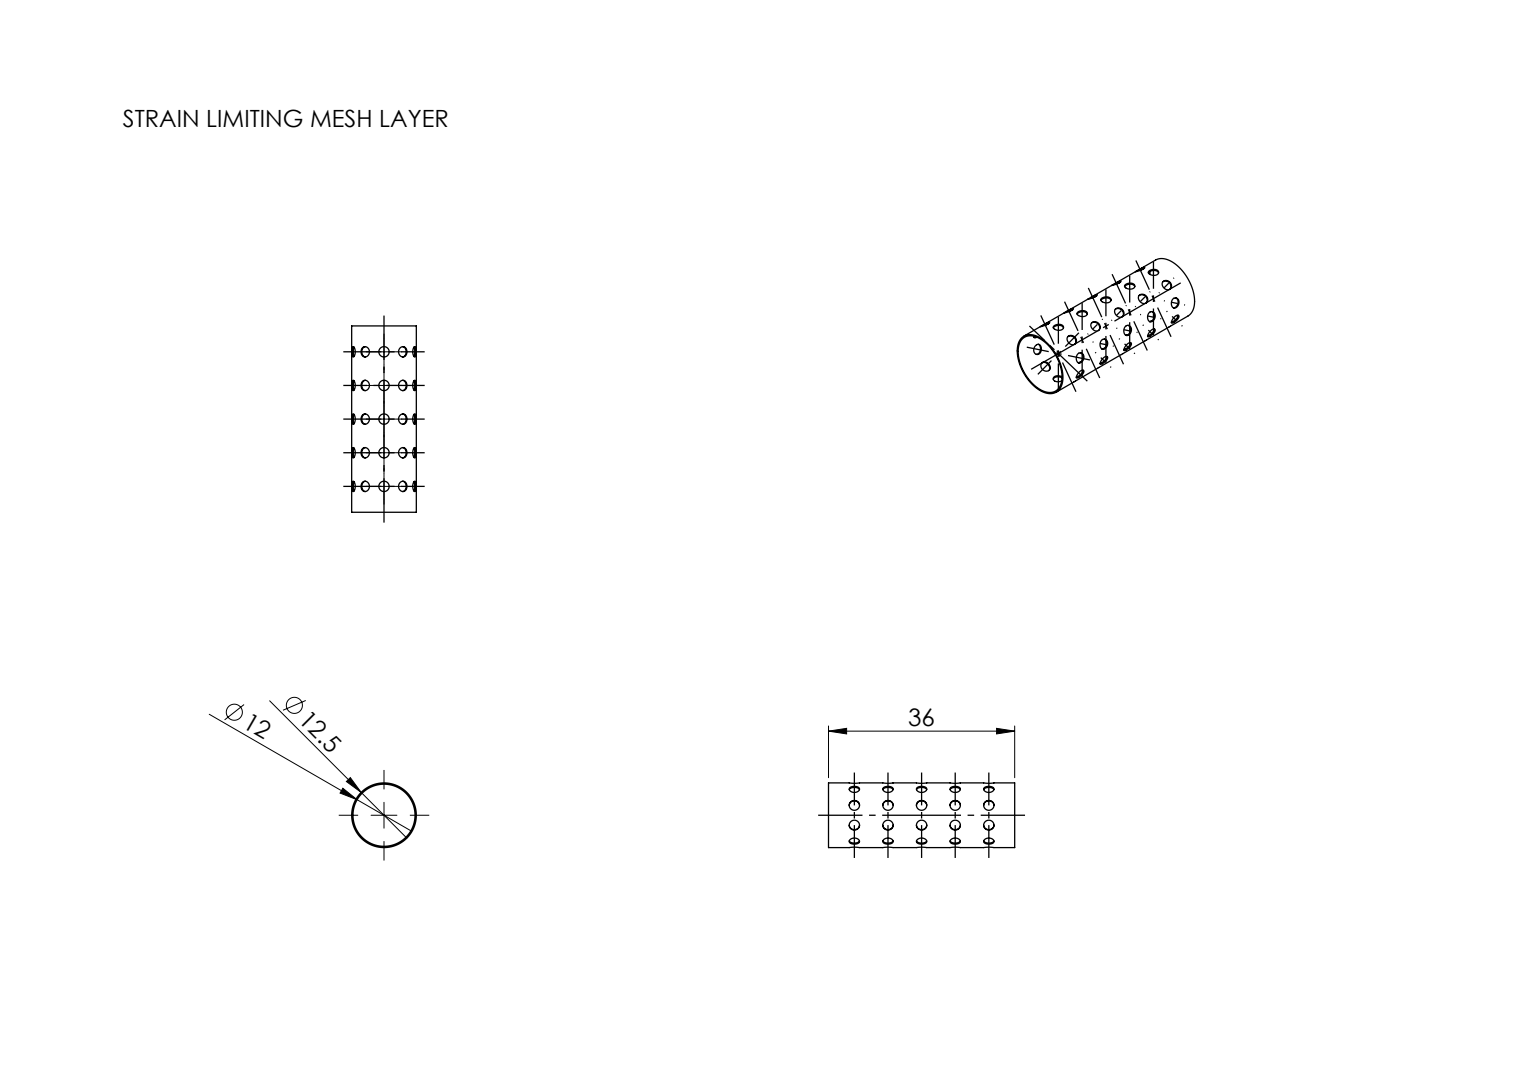
ISO-10303-21;
HEADER;
FILE_DESCRIPTION (('STEP AP214'),
    '1' );
FILE_NAME ('strain limiting mesh layer.step',
    '2026-10-04T10:31:01',
    ( '' ),
    ( '' ),
    'SwSTEP 2.0',
    'SolidWorks 2026',
    '' );
FILE_SCHEMA (( 'AUTOMOTIVE_DESIGN' ));
ENDSEC;

DATA;
#2=CARTESIAN_POINT ( 'NONE',  ( -5.408775798201173046, 2.598833957129639494, 10.88602261056916554 ) ) ;
#3=CARTESIAN_POINT ( 'NONE',  ( 5.866817325727491372, 1.260653813892048003, 4.199777826161211536 ) ) ;
#4=CARTESIAN_POINT ( 'NONE',  ( -5.621278735166248097, 2.101423246382425614, 30.02591947216899015 ) ) ;
#5=ORIENTED_EDGE ( 'NONE', *, *, #943, .F. ) ;
#6=ADVANCED_FACE ( 'NONE', ( #14827 ), #6324, .F. ) ;
#7=VECTOR ( 'NONE', #2853, 1000.000000000000000 ) ;
#11=EDGE_CURVE ( 'NONE', #6555, #15690, #9827, .T. ) ;
#12=EDGE_LOOP ( 'NONE', ( #2014, #1529, #7352, #6634 ) ) ;
#20=FACE_OUTER_BOUND ( 'NONE', #6226, .T. ) ;
#24=CARTESIAN_POINT ( 'NONE',  ( 6.081836621194421255, 1.445163676684907417, 5.873058915543010627 ) ) ;
#27=EDGE_LOOP ( 'NONE', ( #6618, #1977 ) ) ;
#28=VERTEX_POINT ( 'NONE', #11082 ) ;
#30=DIRECTION ( 'NONE',  ( 0.000000000000000000, 1.000000000000000000, 0.000000000000000000 ) ) ;
#32=CARTESIAN_POINT ( 'NONE',  ( -6.176542424588117974, 0.9554180641285662245, 31.13234125634169658 ) ) ;
#34=CARTESIAN_POINT ( 'NONE',  ( -3.107583187530418289, -5.133966411712689748, 12.37380682714709401 ) ) ;
#35=CARTESIAN_POINT ( 'NONE',  ( -5.769755079862331826, 2.405651898698942581, 5.873058915543010627 ) ) ;
#36=CARTESIAN_POINT ( 'NONE',  ( -6.176542424588075342, -0.9554180641288342324, 24.36765874365829987 ) ) ;
#37=CARTESIAN_POINT ( 'NONE',  ( 0.9999502950804096679, -5.916088184763849789, 24.63108149190011176 ) ) ;
#46=FACE_OUTER_BOUND ( 'NONE', #102, .T. ) ;
#47=CARTESIAN_POINT ( 'NONE',  ( 7.799024015210693328, -1.482594289696895551, 24.49999999999999289 ) ) ;
#50=CARTESIAN_POINT ( 'NONE',  ( -3.420311045507875125, 4.931422832349270813, 10.49992038825521767 ) ) ;
#51=EDGE_CURVE ( 'NONE', #13172, #10136, #3947, .T. ) ;
#53=LINE ( 'NONE', #4919, #15568 ) ;
#56=CARTESIAN_POINT ( 'NONE',  ( -4.070051655338111196, 4.744673454622471809, 5.873673286359928802 ) ) ;
#60=CARTESIAN_POINT ( 'NONE',  ( 5.558508435838322548, -2.857531096718671115, 24.49999999999999289 ) ) ;
#62=DIRECTION ( 'NONE',  ( -0.5877852522924685852, -0.8090169943749507819, 0.000000000000000000 ) ) ;
#66=CARTESIAN_POINT ( 'NONE',  ( 3.566234721238059624, 5.134387337253815353, 30.00008258189710730 ) ) ;
#69=CARTESIAN_POINT ( 'NONE',  ( 0.6151877315911880029, -6.220340188095996758, 25.29906673469669443 ) ) ;
#71=CARTESIAN_POINT ( 'NONE',  ( 2.817313151350924638, 5.579000502529565253, 24.49999999999999289 ) ) ;
#72=DIRECTION ( 'NONE',  ( -0.5877852522924685852, -0.8090169943749508930, 0.000000000000000000 ) ) ;
#74=CARTESIAN_POINT ( 'NONE',  ( 4.005785023174416537, -4.467917056767432449, 18.79952054102714243 ) ) ;
#76=CARTESIAN_POINT ( 'NONE',  ( -0.9737778612005270062, -5.920671847850523584, 30.73736375884650585 ) ) ;
#78=EDGE_CURVE ( 'NONE', #4035, #7910, #13252, .T. ) ;
#79=CARTESIAN_POINT ( 'NONE',  ( -0.9740012993918838458, -6.173846968979659344, 18.26164920628437471 ) ) ;
#83=B_SPLINE_CURVE_WITH_KNOTS ( 'NONE', 3,
 ( #5175, #14802, #5099, #8688, #8760, #13593, #1502, #6378, #11290, #544, #7481, #9951, #10027, #7789, #7554, #1580, #2625, #11212 ),
 .UNSPECIFIED., .F., .F.,
 ( 4, 2, 2, 2, 2, 2, 2, 2, 4 ),
 ( 0.000000000000000000, 0.0003914898357794967363, 0.0007829796715589934725, 0.001174469507338490263, 0.001565959343117986945, 0.001957449178897483627, 0.002348939014676980526, 0.002740428850456476991, 0.003131918686235973890 ),
 .UNSPECIFIED. ) ;
#85=ORIENTED_EDGE ( 'NONE', *, *, #14143, .F. ) ;
#86=CARTESIAN_POINT ( 'NONE',  ( -2.692215568229989753, 5.362327947133520567, 24.76229037835931734 ) ) ;
#89=CARTESIAN_POINT ( 'NONE',  ( 5.903472034603520768, 2.056448723545130974, 19.00008219321555103 ) ) ;
#90=CARTESIAN_POINT ( 'NONE',  ( 6.106056299406735555, 1.336851112280737386, 31.79887838423339730 ) ) ;
#92=EDGE_CURVE ( 'NONE', #15044, #5826, #4325, .T. ) ;
#95=LINE ( 'NONE', #7268, #828 ) ;
#97=CARTESIAN_POINT ( 'NONE',  ( 3.421280866381150698, 4.930711975950905490, 6.000049320733126024 ) ) ;
#99=CARTESIAN_POINT ( 'NONE',  ( 4.435347140101059793, -4.403429997944484420, 30.86762589283693714 ) ) ;
#102=EDGE_LOOP ( 'NONE', ( #11466, #15646, #12937, #12328 ) ) ;
#105=CARTESIAN_POINT ( 'NONE',  ( 1.354942165200771727E-13, 6.000000000000000888, 16.99999999999998579 ) ) ;
#107=CARTESIAN_POINT ( 'NONE',  ( 7.347880431581855163E-16, -6.250000000000000888, 4.000000000000004441 ) ) ;
#108=CARTESIAN_POINT ( 'NONE',  ( 3.010624175977998807, -5.190832888732208161, 12.29888242247939623 ) ) ;
#109=VECTOR ( 'NONE', #6035, 1000.000000000000114 ) ;
#111=CARTESIAN_POINT ( 'NONE',  ( 0.5042987395408317086, 5.979983180450071600, 12.37329304179975509 ) ) ;
#112=CARTESIAN_POINT ( 'NONE',  ( -0.2637975869345823843, -6.245592211692903462, 25.47332839949191197 ) ) ;
#114=CARTESIAN_POINT ( 'NONE',  ( -5.858813228503674253, 2.179803269293212331, 5.973772828752684561 ) ) ;
#115=CARTESIAN_POINT ( 'NONE',  ( 5.931828553037963303, 0.9033193133619970006, 30.73805675996854703 ) ) ;
#120=CARTESIAN_POINT ( 'NONE',  ( 5.866817325727508248, 1.260653813891974062, 10.69977782616119732 ) ) ;
#122=EDGE_LOOP ( 'NONE', ( #8457, #957, #1817, #14670 ) ) ;
#123=CARTESIAN_POINT ( 'NONE',  ( -3.735642931251032639, 4.696778275484473575, 5.974080527831013399 ) ) ;
#124=DIRECTION ( 'NONE',  ( -0.3090169943749584980, 0.9510565162951498674, 0.000000000000000000 ) ) ;
#125=CARTESIAN_POINT ( 'NONE',  ( 0.000000000000000000, 6.250000000000000888, 25.49999999999999645 ) ) ;
#126=CARTESIAN_POINT ( 'NONE',  ( 0.5031281619709804254, 5.980084330432649864, 23.62602272744524967 ) ) ;
#128=CARTESIAN_POINT ( 'NONE',  ( -2.782769401326250058, 5.315896561274810139, 10.99571079637980553 ) ) ;
#130=CARTESIAN_POINT ( 'NONE',  ( 5.621197618055712830, -2.101623592078416980, 4.026019798777604741 ) ) ;
#131=AXIS2_PLACEMENT_3D ( 'NONE', #7436, #13712, #10064 ) ;
#132=LINE ( 'NONE', #11034, #13057 ) ;
#137=CARTESIAN_POINT ( 'NONE',  ( 0.7995298244854847081, 5.947211616899245712, 31.61456014619858834 ) ) ;
#138=EDGE_LOOP ( 'NONE', ( #2074, #6168, #2631, #14050 ) ) ;
#141=CARTESIAN_POINT ( 'NONE',  ( -4.290821322214377176, -4.545321419741554791, 12.11441947245482886 ) ) ;
#142=VECTOR ( 'NONE', #3301, 1000.000000000000114 ) ;
#145=CYLINDRICAL_SURFACE ( 'NONE', #13956, 1.000000000000000888 ) ;
#149=DIRECTION ( 'NONE',  ( 0.8090169943749421222, 0.5877852522924802425, 0.000000000000000000 ) ) ;
#151=CARTESIAN_POINT ( 'NONE',  ( 5.782895619916224028, -1.604017620857841386, 25.47408052783099919 ) ) ;
#153=CARTESIAN_POINT ( 'NONE',  ( -1.000079958708118610, -5.916066267613704355, 31.13152738882033788 ) ) ;
#154=CARTESIAN_POINT ( 'NONE',  ( 5.621197618055728817, -2.101623592078373903, 10.52601979877759142 ) ) ;
#155=CARTESIAN_POINT ( 'NONE',  ( -4.435347140101089103, 4.403429997944455110, 31.00000000000000000 ) ) ;
#157=CARTESIAN_POINT ( 'NONE',  ( -5.935543223013860725, 0.8771126767606856056, 30.86760611998365178 ) ) ;
#158=EDGE_CURVE ( 'NONE', #3364, #642, #4897, .T. ) ;
#159=VERTEX_POINT ( 'NONE', #1682 ) ;
#160=EDGE_CURVE ( 'NONE', #4150, #13293, #5091, .T. ) ;
#163=CARTESIAN_POINT ( 'NONE',  ( -5.329907877631262281, -2.755840666746435019, 24.76194324003146008 ) ) ;
#165=ORIENTED_EDGE ( 'NONE', *, *, #10559, .T. ) ;
#172=CARTESIAN_POINT ( 'NONE',  ( -5.558508435838229289, 2.857531096718854524, 5.000000000000004441 ) ) ;
#174=CARTESIAN_POINT ( 'NONE',  ( 2.668367453516629517, 5.373994336898131330, 5.130649613488545313 ) ) ;
#178=EDGE_CURVE ( 'NONE', #5942, #5121, #706, .T. ) ;
#184=B_SPLINE_CURVE_WITH_KNOTS ( 'NONE', 3,
 ( #1419, #11210, #385, #5255, #7552, #10102, #6529, #6608, #14955, #11441, #11134, #235, #4046, #5097, #5411, #8917, #12556, #1655 ),
 .UNSPECIFIED., .F., .F.,
 ( 4, 2, 2, 2, 2, 2, 2, 2, 4 ),
 ( 0.003131918686235975625, 0.003523310662250265894, 0.003914702638264556597, 0.004306094614278846433, 0.004697486590293137136, 0.005088878566307427839, 0.005480270542321717675, 0.005871662518336007511, 0.006263054494350298214 ),
 .UNSPECIFIED. ) ;
#185=CARTESIAN_POINT ( 'NONE',  ( 6.123233995736766282E-16, -6.000000000000000888, 6.000000000000005329 ) ) ;
#186=CARTESIAN_POINT ( 'NONE',  ( 0.1306394121200732117, -6.249999999999998224, 16.99999999999998934 ) ) ;
#189=DIRECTION ( 'NONE',  ( -0.5877852522924685852, -0.8090169943749508930, 0.000000000000000000 ) ) ;
#190=CARTESIAN_POINT ( 'NONE',  ( 5.486982057989218120, -2.429327048029818137, 12.29931806258173488 ) ) ;
#191=CARTESIAN_POINT ( 'NONE',  ( -7.799024015210622274, -1.482594289697344969, 17.99999999999998934 ) ) ;
#203=CARTESIAN_POINT ( 'NONE',  ( -6.176542424588105540, -0.9554180641286327269, 5.000000000000004441 ) ) ;
#204=CARTESIAN_POINT ( 'NONE',  ( -5.859221468178929193, 2.178708437343280568, 23.52591457665828401 ) ) ;
#207=CARTESIAN_POINT ( 'NONE',  ( 6.176542424588116198, 0.9554180641285651143, 11.63060690723497537 ) ) ;
#212=CARTESIAN_POINT ( 'NONE',  ( 4.322356511625485176, 7.650514973136679941, 24.49999999999999289 ) ) ;
#216=CARTESIAN_POINT ( 'NONE',  ( -0.6144300524833441468, -6.220417338033054300, 30.20033372175933550 ) ) ;
#221=CARTESIAN_POINT ( 'NONE',  ( -3.567624405365271478, -5.133384272590760133, 10.50004921015705150 ) ) ;
#223=VECTOR ( 'NONE', #5063, 1000.000000000000114 ) ;
#225=CARTESIAN_POINT ( 'NONE',  ( 6.172651332693116721, -0.9815532474592382206, 18.26190213084011660 ) ) ;
#227=CARTESIAN_POINT ( 'NONE',  ( -3.735642931251134335, -4.696778275484388310, 23.52591947216897594 ) ) ;
#229=CARTESIAN_POINT ( 'NONE',  ( 5.903596343266298341, -2.055998103990583026, 31.99995078984293428 ) ) ;
#230=CARTESIAN_POINT ( 'NONE',  ( 5.131373506000437068, 7.062729720844210135, 24.49999999999999289 ) ) ;
#235=CARTESIAN_POINT ( 'NONE',  ( 3.922396193919112317, -4.541970110199391009, 5.873806827147107334 ) ) ;
#236=CARTESIAN_POINT ( 'NONE',  ( -5.746837578676007752, 1.729433780394243003, 10.50004946353775459 ) ) ;
#243=ORIENTED_EDGE ( 'NONE', *, *, #15436, .T. ) ;
#245=CARTESIAN_POINT ( 'NONE',  ( -2.782713018890816681, 5.315928322779066129, 25.00439760644211518 ) ) ;
#249=CARTESIAN_POINT ( 'NONE',  ( 5.770288754215144422, 2.404361317819916355, 18.87381964045070859 ) ) ;
#253=ADVANCED_FACE ( 'NONE', ( #9289 ), #846, .F. ) ;
#254=DIRECTION ( 'NONE',  ( 0.000000000000000000, 1.000000000000000000, 0.000000000000000000 ) ) ;
#255=DIRECTION ( 'NONE',  ( 0.8090169943749421222, 0.5877852522924802425, 0.000000000000000000 ) ) ;
#257=CARTESIAN_POINT ( 'NONE',  ( -6.155867707731118799, 1.081837891425841747, 30.49563030319847101 ) ) ;
#259=ORIENTED_EDGE ( 'NONE', *, *, #5440, .T. ) ;
#262=CARTESIAN_POINT ( 'NONE',  ( 5.330189595673648917, -2.755293208590215315, 30.73617396794403689 ) ) ;
#263=CARTESIAN_POINT ( 'NONE',  ( 4.153440676704428292, 4.671190581744466108, 4.200455375311575423 ) ) ;
#264=ORIENTED_EDGE ( 'NONE', *, *, #8261, .T. ) ;
#265=CARTESIAN_POINT ( 'NONE',  ( -6.155854678529451895, -1.081900940642234854, 17.49574050496990552 ) ) ;
#266=CARTESIAN_POINT ( 'NONE',  ( -2.849573632035295567, -5.280958870664590243, 18.61561732698604743 ) ) ;
#268=CARTESIAN_POINT ( 'NONE',  ( 3.254737477227910514, -5.337033878705263135, 23.62632671364006498 ) ) ;
#270=CARTESIAN_POINT ( 'NONE',  ( -3.159082487394833105, 5.393634094348302099, 10.70045537531157365 ) ) ;
#271=CARTESIAN_POINT ( 'NONE',  ( 1.000049560716759212, -5.916071405810109596, 24.36967799011533131 ) ) ;
#278=VERTEX_POINT ( 'NONE', #3158 ) ;
#279=CARTESIAN_POINT ( 'NONE',  ( -4.005361199354998014, 4.468319061418771554, 5.800222173838807116 ) ) ;
#281=CARTESIAN_POINT ( 'NONE',  ( -3.420311045507988368, 4.931422832349193541, 23.49992038825522656 ) ) ;
#284=CARTESIAN_POINT ( 'NONE',  ( -4.344762547369668049, -4.493114738039260203, 31.50308643866046054 ) ) ;
#287=CARTESIAN_POINT ( 'NONE',  ( -3.255013540813805673, 5.336859797930734395, 23.62618035954928786 ) ) ;
#290=CARTESIAN_POINT ( 'NONE',  ( 5.665707375537430757, 1.979196487016795292, 6.000079611744768115 ) ) ;
#292=FACE_OUTER_BOUND ( 'NONE', #8134, .T. ) ;
#295=B_SPLINE_CURVE_WITH_KNOTS ( 'NONE', 3,
 ( #10005, #367, #7304, #7609, #8735, #12457, #14777, #9696, #13567, #2677, #130, #7529, #13493, #1395, #2441, #6195, #14533, #1557 ),
 .UNSPECIFIED., .F., .F.,
 ( 4, 2, 2, 2, 2, 2, 2, 2, 4 ),
 ( 0.003131918686235955242, 0.003523310662250247680, 0.003914702638264540117, 0.004306094614278832555, 0.004697486590293124993, 0.005088878566307417431, 0.005480270542321709869, 0.005871662518336002307, 0.006263054494350294744 ),
 .UNSPECIFIED. ) ;
#296=CARTESIAN_POINT ( 'NONE',  ( 2.817313151351047207, 5.579000502529503080, 11.63063932754212892 ) ) ;
#298=AXIS2_PLACEMENT_3D ( 'NONE', #11149, #8855, #14815 ) ;
#300=CARTESIAN_POINT ( 'NONE',  ( 5.858736126997204252, -2.179962889276876314, 18.97359571723300320 ) ) ;
#303=CARTESIAN_POINT ( 'NONE',  ( -3.735642931251081489, -4.696778275484434495, 17.02591947216898305 ) ) ;
#305=B_SPLINE_CURVE_WITH_KNOTS ( 'NONE', 3,
 ( #6852, #13275, #12000, #11047, #9939, #6048, #6284, #2613, #8750, #15671, #227, #12235, #5087, #7393, #2293, #1336, #14715, #2456 ),
 .UNSPECIFIED., .F., .F.,
 ( 4, 2, 2, 2, 2, 2, 2, 2, 4 ),
 ( 0.000000000000000000, 0.0003914898357794977120, 0.0007829796715589954241, 0.001174469507338493082, 0.001565959343117990848, 0.001957449178897487096, 0.002348939014676983995, 0.002740428850456480461, 0.003131918686235977359 ),
 .UNSPECIFIED. ) ;
#306=CARTESIAN_POINT ( 'NONE',  ( -5.842945980534678618, 1.369128644668824446, 4.126215691297385746 ) ) ;
#307=FACE_OUTER_BOUND ( 'NONE', #5177, .T. ) ;
#308=CARTESIAN_POINT ( 'NONE',  ( 3.735808404764892732, 4.696639218303211294, 17.02601979877759319 ) ) ;
#312=CARTESIAN_POINT ( 'NONE',  ( -0.9737725088280894115, -6.173885267451843184, 17.73735758726564882 ) ) ;
#318=EDGE_LOOP ( 'NONE', ( #11239, #13450, #15608, #14902 ) ) ;
#322=CARTESIAN_POINT ( 'NONE',  ( -5.915653884842670962, -1.003805156977642943, 25.00439760644211518 ) ) ;
#324=ORIENTED_EDGE ( 'NONE', *, *, #12407, .T. ) ;
#328=CARTESIAN_POINT ( 'NONE',  ( -5.940390500375766436, 6.474944468551470322, 17.99999999999998934 ) ) ;
#331=CARTESIAN_POINT ( 'NONE',  ( -4.005361199354992685, -4.468319061418773330, 10.69977782616119022 ) ) ;
#332=CARTESIAN_POINT ( 'NONE',  ( 2.692143549875401831, 5.362363179736477470, 5.261943240031468960 ) ) ;
#334=CARTESIAN_POINT ( 'NONE',  ( 5.616116467183661420, -2.743044348085539319, 10.99574050496990019 ) ) ;
#335=CARTESIAN_POINT ( 'NONE',  ( -0.9735954530125078277, 6.173909381473996483, 31.26281793585242852 ) ) ;
#336=ORIENTED_EDGE ( 'NONE', *, *, #9119, .T. ) ;
#337=ORIENTED_EDGE ( 'NONE', *, *, #6167, .T. ) ;
#339=CARTESIAN_POINT ( 'NONE',  ( 0.2638277032950181455, 5.995407492418034501, 18.97332055281517427 ) ) ;
#341=ORIENTED_EDGE ( 'NONE', *, *, #869, .F. ) ;
#344=CARTESIAN_POINT ( 'NONE',  ( 0.8002302970946665317, -5.947135855825865569, 30.38601773212297985 ) ) ;
#345=CARTESIAN_POINT ( 'NONE',  ( -3.255128505894313573, 5.336774832660720058, 31.87380055247395561 ) ) ;
#346=CARTESIAN_POINT ( 'NONE',  ( 0.5030929395821815975, 6.230885867001134670, 17.12600319116549841 ) ) ;
#348=CARTESIAN_POINT ( 'NONE',  ( 5.131373506000546314, 7.062729720844130199, 11.49999999999998224 ) ) ;
#349=CARTESIAN_POINT ( 'NONE',  ( 5.665824935993635236, -1.978765057080846601, 12.49995053646221166 ) ) ;
#350=CARTESIAN_POINT ( 'NONE',  ( -3.882673863916385137, 4.899192824800864265, 18.97408542334169823 ) ) ;
#357=ORIENTED_EDGE ( 'NONE', *, *, #9015, .F. ) ;
#358=EDGE_CURVE ( 'NONE', #3603, #7463, #3951, .T. ) ;
#359=CARTESIAN_POINT ( 'NONE',  ( -6.176542424588100211, 0.9554180641286806885, 17.86762589283693359 ) ) ;
#361=CARTESIAN_POINT ( 'NONE',  ( -0.7993401192311853087, 6.199366368793661763, 5.614832469365748757 ) ) ;
#362=CARTESIAN_POINT ( 'NONE',  ( 5.903472034603497676, 2.056448723545192259, 12.50008219321554570 ) ) ;
#364=EDGE_CURVE ( 'NONE', #4594, #6555, #9214, .T. ) ;
#365=CARTESIAN_POINT ( 'NONE',  ( 2.848235266350880757, -5.281699484015723201, 23.88602261056919218 ) ) ;
#367=CARTESIAN_POINT ( 'NONE',  ( 5.935543223013858061, -0.8771126767606637342, 4.869383044678627925 ) ) ;
#368=CARTESIAN_POINT ( 'NONE',  ( -4.416837305303453753, -4.422286678979054919, 30.73809786915987630 ) ) ;
#370=FACE_BOUND ( 'NONE', #9710, .T. ) ;
#376=CARTESIAN_POINT ( 'NONE',  ( -5.866984344570811416, -1.259800266528728008, 18.79931806258173665 ) ) ;
#378=ORIENTED_EDGE ( 'NONE', *, *, #15661, .F. ) ;
#382=CARTESIAN_POINT ( 'NONE',  ( 3.922396193918944896, 4.541970110199535782, 17.12619317285288645 ) ) ;
#385=CARTESIAN_POINT ( 'NONE',  ( 2.692335458626972766, -5.362264153667172906, 5.262398918055980701 ) ) ;
#386=CARTESIAN_POINT ( 'NONE',  ( -3.923477796648569882, 4.541042560386435945, 30.12696220972948780 ) ) ;
#389=ORIENTED_EDGE ( 'NONE', *, *, #6341, .F. ) ;
#392=ORIENTED_EDGE ( 'NONE', *, *, #2098, .F. ) ;
#394=ORIENTED_EDGE ( 'NONE', *, *, #3851, .T. ) ;
#395=ADVANCED_FACE ( 'NONE', ( #5557 ), #9444, .F. ) ;
#396=CARTESIAN_POINT ( 'NONE',  ( 2.082642335314403343E-14, -6.250000000000000888, 31.00000000000000000 ) ) ;
#397=CYLINDRICAL_SURFACE ( 'NONE', #7859, 1.000000000000000888 ) ;
#398=VERTEX_POINT ( 'NONE', #14205 ) ;
#400=CARTESIAN_POINT ( 'NONE',  ( -4.290821322214388722, 4.545321419741542357, 4.385580527545153373 ) ) ;
#404=CARTESIAN_POINT ( 'NONE',  ( -5.984595133899170527, -1.806709459528687667, 5.999950789842938725 ) ) ;
#405=CARTESIAN_POINT ( 'NONE',  ( -2.849269941561969333, -5.281123252784043487, 10.88480617551147667 ) ) ;
#411=ORIENTED_EDGE ( 'NONE', *, *, #6538, .F. ) ;
#415=CARTESIAN_POINT ( 'NONE',  ( 0.7988914244719601543, 5.947301735519265442, 17.38456289168617985 ) ) ;
#417=ORIENTED_EDGE ( 'NONE', *, *, #12558, .T. ) ;
#418=CARTESIAN_POINT ( 'NONE',  ( -0.5031281619707669295, -5.980084330432671180, 4.126022727445256777 ) ) ;
#419=CARTESIAN_POINT ( 'NONE',  ( -6.176542424588117974, 0.9554180641285661135, 31.00000000000000000 ) ) ;
#420=CARTESIAN_POINT ( 'NONE',  ( -0.5039005892419784471, 6.230833003620553256, 17.12636388911295526 ) ) ;
#421=CARTESIAN_POINT ( 'NONE',  ( 0.2623718222036656722, 6.245654667075778654, 17.02627829713834373 ) ) ;
#425=CARTESIAN_POINT ( 'NONE',  ( 5.935543223013868719, 0.8771126767606117758, 18.13061695532137563 ) ) ;
#430=EDGE_LOOP ( 'NONE', ( #165, #8727 ) ) ;
#432=ORIENTED_EDGE ( 'NONE', *, *, #11524, .T. ) ;
#433=CARTESIAN_POINT ( 'NONE',  ( -5.615973259022290165, 2.743340227996234226, 17.49610786875029689 ) ) ;
#434=CARTESIAN_POINT ( 'NONE',  ( -6.142908455506919552, 1.155755562476170839, 23.88482219624156855 ) ) ;
#436=CARTESIAN_POINT ( 'NONE',  ( 5.571002711501404470, 2.833546409886289030, 11.76379616840804232 ) ) ;
#438=CARTESIAN_POINT ( 'NONE',  ( 2.840966774240223369, 5.567223638426877841, 5.261902130840121039 ) ) ;
#442=B_SPLINE_CURVE_WITH_KNOTS ( 'NONE', 3,
 ( #14232, #2140, #3189, #9317, #15286, #5742, #4389, #1910, #5509, #9242, #12806, #718, #1989, #8126, #11536, #6706, #14078, #6862 ),
 .UNSPECIFIED., .F., .F.,
 ( 4, 2, 2, 2, 2, 2, 2, 2, 4 ),
 ( 0.003131918686235976492, 0.003523310662250267195, 0.003914702638264558332, 0.004306094614278849035, 0.004697486590293139738, 0.005088878566307430441, 0.005480270542321721144, 0.005871662518336011848, 0.006263054494350302551 ),
 .UNSPECIFIED. ) ;
#443=DIRECTION ( 'NONE',  ( 0.000000000000000000, 1.000000000000000000, 0.000000000000000000 ) ) ;
#445=EDGE_CURVE ( 'NONE', #2248, #14335, #14582, .T. ) ;
#449=CARTESIAN_POINT ( 'NONE',  ( -2.997451966578398075, -5.485105005466015982, 10.88482219624155967 ) ) ;
#452=CARTESIAN_POINT ( 'NONE',  ( -2.782713018890758061, 5.315928322779098991, 18.50439760644211518 ) ) ;
#455=CARTESIAN_POINT ( 'NONE',  ( -2.841041022017427142, -5.567186575787240521, 17.73774718278285434 ) ) ;
#456=VECTOR ( 'NONE', #13750, 1000.000000000000000 ) ;
#458=FACE_OUTER_BOUND ( 'NONE', #7735, .T. ) ;
#462=DIRECTION ( 'NONE',  ( 0.5877852522924802425, -0.8090169943749422332, 0.000000000000000000 ) ) ;
#463=CARTESIAN_POINT ( 'NONE',  ( -5.935543223013843850, -0.8771126767607685393, 31.00000000000000000 ) ) ;
#464=AXIS2_PLACEMENT_3D ( 'NONE', #9917, #5307, #2906 ) ;
#465=CYLINDRICAL_SURFACE ( 'NONE', #13069, 1.000000000000000222 ) ;
#467=VECTOR ( 'NONE', #1666, 1000.000000000000000 ) ;
#468=CARTESIAN_POINT ( 'NONE',  ( -5.620879908643933831, -2.102487719021981949, 10.52622176056705428 ) ) ;
#471=VERTEX_POINT ( 'NONE', #4671 ) ;
#472=CARTESIAN_POINT ( 'NONE',  ( -5.915641100987803824, 1.003868594704913519, 25.00428920362019625 ) ) ;
#473=ORIENTED_EDGE ( 'NONE', *, *, #2610, .T. ) ;
#474=EDGE_CURVE ( 'NONE', #3929, #6460, #15716, .T. ) ;
#475=CYLINDRICAL_SURFACE ( 'NONE', #10388, 1.000000000000000666 ) ;
#478=VERTEX_POINT ( 'NONE', #125 ) ;
#479=AXIS2_PLACEMENT_3D ( 'NONE', #15199, #7061, #4294 ) ;
#484=CARTESIAN_POINT ( 'NONE',  ( -6.176542424588106428, -0.9554180641286325049, 5.132374107163055754 ) ) ;
#485=CARTESIAN_POINT ( 'NONE',  ( -4.286401442266578599, -4.198423832313146420, 11.49999999999998224 ) ) ;
#489=CARTESIAN_POINT ( 'NONE',  ( 4.142173849413700815, 4.341773579105447922, 12.11519382448850557 ) ) ;
#490=ORIENTED_EDGE ( 'NONE', *, *, #8030, .T. ) ;
#493=ORIENTED_EDGE ( 'NONE', *, *, #9967, .T. ) ;
#494=EDGE_CURVE ( 'NONE', #11779, #1022, #11976, .T. ) ;
#496=CARTESIAN_POINT ( 'NONE',  ( -6.176542424588095770, -0.9554180641287001174, 11.49999999999998224 ) ) ;
#497=CARTESIAN_POINT ( 'NONE',  ( 5.903596343266263702, 2.055998103990681614, 4.000049210157071045 ) ) ;
#498=EDGE_LOOP ( 'NONE', ( #13781, #14669 ) ) ;
#500=CARTESIAN_POINT ( 'NONE',  ( 1.354942164390165777E-13, -6.250000000000000888, 16.99999999999998579 ) ) ;
#502=CARTESIAN_POINT ( 'NONE',  ( -5.330004929009617420, 2.755647751839342519, 5.262398918055979813 ) ) ;
#505=CARTESIAN_POINT ( 'NONE',  ( 2.668367453516569121, 5.373994336898161528, 11.36938304467859773 ) ) ;
#511=B_SPLINE_CURVE_WITH_KNOTS ( 'NONE', 3,
 ( #8242, #10938, #9758, #13397, #14433, #4661, #3454, #10855, #2341, #13243, #11014, #2259, #5933, #3375, #14601, #14346, #36, #7047 ),
 .UNSPECIFIED., .F., .F.,
 ( 4, 2, 2, 2, 2, 2, 2, 2, 4 ),
 ( 0.003131486019301990727, 0.003522824630466696565, 0.003914163241631402404, 0.004305501852796108676, 0.004696840463960814081, 0.005088179075125522088, 0.005479517686290229228, 0.005870856297454936368, 0.006262194908619643507 ),
 .UNSPECIFIED. ) ;
#513=CARTESIAN_POINT ( 'NONE',  ( -4.070863287254244511, 4.743975846881662406, 17.12694108445698760 ) ) ;
#514=DIRECTION ( 'NONE',  ( 0.9510565162951499785, 0.3090169943749582204, 0.000000000000000000 ) ) ;
#515=CARTESIAN_POINT ( 'NONE',  ( -0.1306394121199367930, 6.250000000000000888, 4.000000000000004441 ) ) ;
#516=CARTESIAN_POINT ( 'NONE',  ( 5.903596343266268143, 2.055998103990667403, 30.00004921015706572 ) ) ;
#518=CARTESIAN_POINT ( 'NONE',  ( 4.142173849413673281, -4.341773579105472791, 23.88480617551147844 ) ) ;
#520=CARTESIAN_POINT ( 'NONE',  ( -4.267838854167106177, -4.217593933790406702, 31.26239891805596827 ) ) ;
#522=CARTESIAN_POINT ( 'NONE',  ( -5.131373506000878493, 7.062729720843910819, 24.49999999999999289 ) ) ;
#527=FACE_BOUND ( 'NONE', #5862, .T. ) ;
#530=CARTESIAN_POINT ( 'NONE',  ( -5.915653884842685173, -1.003805156977577662, 18.50439760644211518 ) ) ;
#535=CARTESIAN_POINT ( 'NONE',  ( -4.286401442266626560, -4.198423832313095794, 17.86935038651143515 ) ) ;
#536=CARTESIAN_POINT ( 'NONE',  ( 5.935543223013878489, -0.8771126767605277319, 17.86938304467860306 ) ) ;
#541=CARTESIAN_POINT ( 'NONE',  ( -0.6139908388540702422, 5.969238533166615568, 30.19977627912012252 ) ) ;
#543=LINE ( 'NONE', #1579, #12817 ) ;
#544=CARTESIAN_POINT ( 'NONE',  ( -5.666074146197981776, -1.978051345703211839, 12.50004932073310471 ) ) ;
#548=ORIENTED_EDGE ( 'NONE', *, *, #8965, .T. ) ;
#549=CARTESIAN_POINT ( 'NONE',  ( -5.317509234263835260, -2.779225709351231366, 24.49999999999999289 ) ) ;
#551=ORIENTED_EDGE ( 'NONE', *, *, #6800, .F. ) ;
#554=FACE_OUTER_BOUND ( 'NONE', #8032, .T. ) ;
#558=CARTESIAN_POINT ( 'NONE',  ( -0.5039079366031161689, 5.980031194523161453, 17.12637068109811977 ) ) ;
#559=CARTESIAN_POINT ( 'NONE',  ( 5.317509234264064411, -2.779225709350791274, 24.49999999999999289 ) ) ;
#566=CARTESIAN_POINT ( 'NONE',  ( 2.668367453516568677, 5.373994336898162416, 11.63064961348853465 ) ) ;
#567=VERTEX_POINT ( 'NONE', #9606 ) ;
#568=AXIS2_PLACEMENT_3D ( 'NONE', #14972, #12418, #11226 ) ;
#571=CARTESIAN_POINT ( 'NONE',  ( -6.142844459177225325, -1.156093792145260979, 10.88439807107078394 ) ) ;
#572=CARTESIAN_POINT ( 'NONE',  ( 6.155912734541117537, 1.081577393120979780, 4.496107868750329750 ) ) ;
#574=CARTESIAN_POINT ( 'NONE',  ( 5.903347812666375205, -1.076697810262440491, 18.61397738943082203 ) ) ;
#576=CARTESIAN_POINT ( 'NONE',  ( -0.9999505860952112579, 6.169489349035827352, 18.13105903165805799 ) ) ;
#577=CARTESIAN_POINT ( 'NONE',  ( 5.859155363331400856, -2.178872204144929992, 30.02599901976670438 ) ) ;
#580=LINE ( 'NONE', #4165, #11320 ) ;
#581=CARTESIAN_POINT ( 'NONE',  ( 3.922396193918995522, 4.541970110199488708, 10.62619317285287934 ) ) ;
#582=EDGE_CURVE ( 'NONE', #9339, #5163, #6425, .T. ) ;
#586=EDGE_CURVE ( 'NONE', #15318, #4525, #2806, .T. ) ;
#588=CARTESIAN_POINT ( 'NONE',  ( 3.011899281037532461, -5.190111395030209351, 4.199777826161210648 ) ) ;
#590=CARTESIAN_POINT ( 'NONE',  ( 4.435347140101073116, -4.403429997944470209, 5.000000000000004441 ) ) ;
#591=DIRECTION ( 'NONE',  ( -0.9510565162951545304, 0.3090169943749447867, 0.000000000000000000 ) ) ;
#593=CARTESIAN_POINT ( 'NONE',  ( -0.8737888311110042494, 5.936248257219510549, 5.503441851412170571 ) ) ;
#595=CARTESIAN_POINT ( 'NONE',  ( 3.882809187878910606, 4.899079348630070108, 10.52599901976669017 ) ) ;
#596=CARTESIAN_POINT ( 'NONE',  ( 4.069684453406305025, 4.744965295353549273, 5.873800552473966263 ) ) ;
#597=CARTESIAN_POINT ( 'NONE',  ( 6.143143148203058956, -1.154591847827712403, 31.61396179408071916 ) ) ;
#600=CARTESIAN_POINT ( 'NONE',  ( 5.935543223013847403, 0.8771126767607483332, 5.130616955321390726 ) ) ;
#604=CARTESIAN_POINT ( 'NONE',  ( 6.172614129015239648, -0.9817721000788448560, 30.73763026556126832 ) ) ;
#610=CARTESIAN_POINT ( 'NONE',  ( -3.922672396097112824, -4.541739265057652020, 17.12635295315576300 ) ) ;
#613=CARTESIAN_POINT ( 'NONE',  ( -5.487348639458814681, 2.428538342494583890, 23.69977782616121331 ) ) ;
#616=LINE ( 'NONE', #4206, #9107 ) ;
#617=CARTESIAN_POINT ( 'NONE',  ( -0.5039079366032207519, 5.980031194523153459, 30.12637068109813043 ) ) ;
#619=CARTESIAN_POINT ( 'NONE',  ( -4.286401442266607020, 4.198423832313117110, 31.00000000000000000 ) ) ;
#620=CARTESIAN_POINT ( 'NONE',  ( -6.176542424588121527, 0.9554180641285457964, 4.867625892836954904 ) ) ;
#621=DIRECTION ( 'NONE',  ( 0.9510565162951499785, 0.3090169943749582204, 0.000000000000000000 ) ) ;
#624=CARTESIAN_POINT ( 'NONE',  ( 2.668367453516611754, 5.373994336898140212, 30.86938304467861727 ) ) ;
#626=CYLINDRICAL_SURFACE ( 'NONE', #9896, 1.000000000000000888 ) ;
#628=CARTESIAN_POINT ( 'NONE',  ( -5.931734679891443207, -0.9039278060244418933, 30.73617396794404044 ) ) ;
#629=CARTESIAN_POINT ( 'NONE',  ( -4.344762547369716899, 4.493114738039211353, 4.496913561339538568 ) ) ;
#634=CARTESIAN_POINT ( 'NONE',  ( -4.196038884587174778, -4.289036423669268849, 10.99610204984015205 ) ) ;
#636=DIRECTION ( 'NONE',  ( -0.9510565162951545304, 0.3090169943749447867, 0.000000000000000000 ) ) ;
#637=CARTESIAN_POINT ( 'NONE',  ( 4.344313232727101237, 4.493553492990120191, 31.50436969680151833 ) ) ;
#641=ORIENTED_EDGE ( 'NONE', *, *, #11646, .T. ) ;
#642=VERTEX_POINT ( 'NONE', #5309 ) ;
#643=CARTESIAN_POINT ( 'NONE',  ( 3.010624175977885120, -5.190832888732274775, 25.29888242247941221 ) ) ;
#647=CARTESIAN_POINT ( 'NONE',  ( -1.000049271338347534, 6.169473353325575005, 17.86969612704546506 ) ) ;
#648=CARTESIAN_POINT ( 'NONE',  ( -2.997451966578351001, -5.485105005466042627, 4.384822196241565884 ) ) ;
#651=CARTESIAN_POINT ( 'NONE',  ( -6.176542424588088664, 0.9554180641287480791, 24.49999999999999289 ) ) ;
#652=EDGE_CURVE ( 'NONE', #2035, #3038, #7565, .T. ) ;
#655=CARTESIAN_POINT ( 'NONE',  ( 2.031800924094035195E-13, 6.250000000000000888, 23.49999999999999289 ) ) ;
#657=CARTESIAN_POINT ( 'NONE',  ( 2.930922878467392856, 5.520395124723619595, 18.50389213124969956 ) ) ;
#663=CARTESIAN_POINT ( 'NONE',  ( 6.105747081304198076, 1.338335777572145613, 23.69973484982322631 ) ) ;
#664=CARTESIAN_POINT ( 'NONE',  ( 7.490007020835686369, -2.433650805992243260, 5.000000000000004441 ) ) ;
#665=AXIS2_PLACEMENT_3D ( 'NONE', #12325, #8839, #2782 ) ;
#667=FACE_BOUND ( 'NONE', #2310, .T. ) ;
#668=CARTESIAN_POINT ( 'NONE',  ( 4.435347140100977192, -4.403429997944567020, 17.86762589283694069 ) ) ;
#671=CARTESIAN_POINT ( 'NONE',  ( 5.409423237178978106, 2.597448116731099876, 5.615617326986045654 ) ) ;
#675=UNCERTAINTY_MEASURE_WITH_UNIT (LENGTH_MEASURE( 1.000000000000000082E-05 ), #4499, 'distance_accuracy_value', 'NONE');
#676=FACE_BOUND ( 'NONE', #9747, .T. ) ;
#677=EDGE_CURVE ( 'NONE', #4035, #7387, #11489, .T. ) ;
#678=CARTESIAN_POINT ( 'NONE',  ( 1.000082492230908615, 6.169467968613676412, 24.63152538105401845 ) ) ;
#682=CARTESIAN_POINT ( 'NONE',  ( -2.997451966578608129, 5.485105005465900518, 25.11517780375843500 ) ) ;
#689=CARTESIAN_POINT ( 'NONE',  ( -5.329907877631303137, 2.755840666746359968, 24.23805675996852926 ) ) ;
#692=DIRECTION ( 'NONE',  ( -0.3090169943749579429, 0.9510565162951502005, 0.000000000000000000 ) ) ;
#695=CARTESIAN_POINT ( 'NONE',  ( 5.570760634536804368, -2.834026536768245563, 5.262252817217141221 ) ) ;
#697=CARTESIAN_POINT ( 'NONE',  ( -3.011139120916464851, -5.190534000030369910, 30.20068193741825979 ) ) ;
#698=ORIENTED_EDGE ( 'NONE', *, *, #8097, .F. ) ;
#704=CARTESIAN_POINT ( 'NONE',  ( -7.490007020835705909, -2.433650805992367161, 5.000000000000004441 ) ) ;
#705=CARTESIAN_POINT ( 'NONE',  ( -3.632151824460997158, -4.777505256984662552, 3.999950679266885523 ) ) ;
#706=B_SPLINE_CURVE_WITH_KNOTS ( 'NONE', 3,
 ( #2538, #5748, #880, #8291, #4628, #9861, #6207, #3345, #66, #4931, #3421, #10590, #13505, #15529, #14713, #1407, #2228, #9481 ),
 .UNSPECIFIED., .F., .F.,
 ( 4, 2, 2, 2, 2, 2, 2, 2, 4 ),
 ( 0.003131486019301977716, 0.003522824630466684856, 0.003914163241631391996, 0.004305501852796100003, 0.004696840463960807142, 0.005088179075125514282, 0.005479517686290222289, 0.005870856297454931164, 0.006262194908619639171 ),
 .UNSPECIFIED. ) ;
#708=CARTESIAN_POINT ( 'NONE',  ( -3.011139120916544787, 5.190534000030322836, 31.79931806258174376 ) ) ;
#709=CARTESIAN_POINT ( 'NONE',  ( 3.566234721237973027, 5.134387337253873973, 17.00008258189708954 ) ) ;
#712=CARTESIAN_POINT ( 'NONE',  ( 5.621197618055776779, -2.101623592078248670, 23.52601979877760030 ) ) ;
#714=AXIS2_PLACEMENT_3D ( 'NONE', #9047, #10461, #4336 ) ;
#717=CYLINDRICAL_SURFACE ( 'NONE', #10044, 0.9999999999999998890 ) ;
#718=CARTESIAN_POINT ( 'NONE',  ( -5.842988226680535746, -1.369004370660826808, 17.12619317285288645 ) ) ;
#719=DIRECTION ( 'NONE',  ( -0.5877852522924685852, -0.8090169943749507819, 0.000000000000000000 ) ) ;
#721=VERTEX_POINT ( 'NONE', #10435 ) ;
#725=CARTESIAN_POINT ( 'NONE',  ( 2.930600586412987152, -5.520563544161741554, 12.00308643866044100 ) ) ;
#727=VERTEX_POINT ( 'NONE', #4463 ) ;
#731=CARTESIAN_POINT ( 'NONE',  ( -0.9735856429310829618, 5.920699391845060333, 24.76285283906726065 ) ) ;
#734=EDGE_CURVE ( 'NONE', #2516, #15573, #442, .T. ) ;
#736=LINE ( 'NONE', #2156, #8210 ) ;
#740=CARTESIAN_POINT ( 'NONE',  ( -5.782947755040659388, -1.603807858344015402, 4.026019798777604741 ) ) ;
#746=ORIENTED_EDGE ( 'NONE', *, *, #9967, .F. ) ;
#747=CARTESIAN_POINT ( 'NONE',  ( -0.9740856415300116478, 6.173834621338605722, 11.23852653055529238 ) ) ;
#748=EDGE_CURVE ( 'NONE', #5121, #5942, #5782, .T. ) ;
#751=EDGE_LOOP ( 'NONE', ( #12486, #12526 ) ) ;
#752=CARTESIAN_POINT ( 'NONE',  ( 4.435347140100961205, 4.403429997944583008, 11.49999999999998224 ) ) ;
#754=CARTESIAN_POINT ( 'NONE',  ( 3.568242062701502793, -5.132954954975523343, 16.99995093123465395 ) ) ;
#757=FILL_AREA_STYLE_COLOUR ( '', #14472 ) ;
#758=CARTESIAN_POINT ( 'NONE',  ( -7.490007020835705909, -2.433650805992367161, 5.000000000000004441 ) ) ;
#762=CARTESIAN_POINT ( 'NONE',  ( 6.176542424588138402, -0.9554180641284093500, 17.86939309276499799 ) ) ;
#764=CARTESIAN_POINT ( 'NONE',  ( -5.531209434046310491, 2.328189801702683415, 18.87303779027050510 ) ) ;
#768=CARTESIAN_POINT ( 'NONE',  ( 7.799024015210637373, -1.482594289697068746, 31.00000000000000000 ) ) ;
#770=DIRECTION ( 'NONE',  ( 0.8090169943749421222, 0.5877852522924802425, 0.000000000000000000 ) ) ;
#772=AXIS2_PLACEMENT_3D ( 'NONE', #14279, #9143, #11588 ) ;
#778=CARTESIAN_POINT ( 'NONE',  ( -5.408775798201170382, -2.598833957129641714, 5.613977389430841569 ) ) ;
#780=FACE_BOUND ( 'NONE', #8537, .T. ) ;
#785=CARTESIAN_POINT ( 'NONE',  ( 3.633127580202252460, 4.776802569231076490, 29.99992038825524432 ) ) ;
#787=DIRECTION ( 'NONE',  ( 0.8090169943749510040, -0.5877852522924683631, 0.000000000000000000 ) ) ;
#789=CARTESIAN_POINT ( 'NONE',  ( -3.632151824461082423, 4.777505256984600379, 32.00004932073311892 ) ) ;
#790=CARTESIAN_POINT ( 'NONE',  ( 5.486982057989201245, 2.429327048029852332, 17.20068193741825269 ) ) ;
#792=EDGE_CURVE ( 'NONE', #15586, #8520, #15272, .T. ) ;
#793=CARTESIAN_POINT ( 'NONE',  ( -0.2619041840692670209, 6.245686665308512353, 23.52605849433794560 ) ) ;
#795=DIRECTION ( 'NONE',  ( 0.000000000000000000, 1.000000000000000000, 0.000000000000000000 ) ) ;
#797=CARTESIAN_POINT ( 'NONE',  ( 0.2619041840695141010, -6.245686665308502583, 30.02605849433794916 ) ) ;
#800=ORIENTED_EDGE ( 'NONE', *, *, #1934, .T. ) ;
#802=ORIENTED_EDGE ( 'NONE', *, *, #3118, .F. ) ;
#804=CARTESIAN_POINT ( 'NONE',  ( -6.176542424588095770, -0.9554180641287002285, 11.36765874365828921 ) ) ;
#806=EDGE_LOOP ( 'NONE', ( #9642, #15273, #10053, #13382 ) ) ;
#809=CARTESIAN_POINT ( 'NONE',  ( -5.487348639458855537, -2.428538342494488855, 31.80022217383877248 ) ) ;
#810=CARTESIAN_POINT ( 'NONE',  ( -4.435347140101010055, -4.403429997944535046, 5.000000000000004441 ) ) ;
#817=B_SPLINE_CURVE_WITH_KNOTS ( 'NONE', 3,
 ( #7421, #9969, #10047, #14663, #2722, #6475, #14577, #8627, #12343, #14895, #3981, #8702, #1438, #6238, #13692, #2486, #3830, #4963 ),
 .UNSPECIFIED., .F., .F.,
 ( 4, 2, 2, 2, 2, 2, 2, 2, 4 ),
 ( 0.003131918686235975191, 0.003523310662250265894, 0.003914702638264556597, 0.004306094614278848168, 0.004697486590293138004, 0.005088878566307429574, 0.005480270542321719410, 0.005871662518336009245, 0.006263054494350298214 ),
 .UNSPECIFIED. ) ;
#818=CARTESIAN_POINT ( 'NONE',  ( -5.842988226680565944, -1.369004370660702463, 4.126193172852896218 ) ) ;
#820=CARTESIAN_POINT ( 'NONE',  ( 4.153663429050664213, 4.670992970568477176, 18.79933148907576168 ) ) ;
#821=ORIENTED_EDGE ( 'NONE', *, *, #13085, .F. ) ;
#825=CARTESIAN_POINT ( 'NONE',  ( -2.997753866155921543, 5.484939622623787869, 17.38439807107078749 ) ) ;
#826=CARTESIAN_POINT ( 'NONE',  ( 7.347880347650999152E-16, -6.000000000000000888, 4.000000000000004441 ) ) ;
#828=VECTOR ( 'NONE', #12028, 1000.000000000000114 ) ;
#829=ORIENTED_EDGE ( 'NONE', *, *, #10697, .T. ) ;
#830=CARTESIAN_POINT ( 'NONE',  ( 4.069800786343749976, 4.744882212776869501, 10.62618035954928075 ) ) ;
#834=CYLINDRICAL_SURFACE ( 'NONE', #6184, 1.000000000000000888 ) ;
#840=CARTESIAN_POINT ( 'NONE',  ( 6.172614129015258300, -0.9817721000787353880, 17.73763026556123634 ) ) ;
#841=CARTESIAN_POINT ( 'NONE',  ( -6.176542424588120639, 0.9554180641285460185, 5.000000000000004441 ) ) ;
#846=CYLINDRICAL_SURFACE ( 'NONE', #9301, 1.000000000000000888 ) ;
#853=CARTESIAN_POINT ( 'NONE',  ( -5.131373506000715068, 7.062729720844030723, 5.000000000000004441 ) ) ;
#854=CARTESIAN_POINT ( 'NONE',  ( 7.490007020835706797, -2.433650805992179755, 11.49999999999998224 ) ) ;
#855=CARTESIAN_POINT ( 'NONE',  ( -0.5044069930203080032, 5.979990686694993229, 31.87335743227904317 ) ) ;
#857=FACE_BOUND ( 'NONE', #1667, .T. ) ;
#858=CARTESIAN_POINT ( 'NONE',  ( -6.155867707731125016, 1.081837891425820430, 4.495630303198471900 ) ) ;
#860=VERTEX_POINT ( 'NONE', #7173 ) ;
#862=CARTESIAN_POINT ( 'NONE',  ( 4.005785023174439630, 4.467917056767417350, 30.20047945897283981 ) ) ;
#863=ORIENTED_EDGE ( 'NONE', *, *, #9514, .T. ) ;
#868=CARTESIAN_POINT ( 'NONE',  ( 5.935543223013889147, -0.8771126767604601193, 24.49999999999999289 ) ) ;
#869=EDGE_CURVE ( 'NONE', #11793, #278, #11659, .T. ) ;
#871=CARTESIAN_POINT ( 'NONE',  ( -5.558508435838188433, -2.857531096718932684, 5.000000000000004441 ) ) ;
#874=CARTESIAN_POINT ( 'NONE',  ( 2.817313151351089395, 5.579000502529482652, 31.13063932754212004 ) ) ;
#880=CARTESIAN_POINT ( 'NONE',  ( 2.841163418881370362, 5.567120626447941589, 30.73763026556126476 ) ) ;
#882=ORIENTED_EDGE ( 'NONE', *, *, #3262, .T. ) ;
#884=CARTESIAN_POINT ( 'NONE',  ( 0.8736516769106962288, -5.936271176698232566, 4.496067715786787211 ) ) ;
#885=CARTESIAN_POINT ( 'NONE',  ( -3.158825713737453800, -5.393784879207189853, 4.200668510924231214 ) ) ;
#888=CARTESIAN_POINT ( 'NONE',  ( 6.155973317223288888, -1.081218830693701394, 4.496913561339538568 ) ) ;
#891=CARTESIAN_POINT ( 'NONE',  ( -5.330004929009576564, -2.755647751839420234, 4.737601081944046832 ) ) ;
#902=VERTEX_POINT ( 'NONE', #11057 ) ;
#903=CARTESIAN_POINT ( 'NONE',  ( 2.817313151351048539, 5.579000502529503969, 11.36939309276499088 ) ) ;
#905=CARTESIAN_POINT ( 'NONE',  ( 3.421280866380972618, 4.930711975951031611, 25.50004932073312247 ) ) ;
#906=FACE_BOUND ( 'NONE', #12968, .T. ) ;
#913=CARTESIAN_POINT ( 'NONE',  ( -5.726307184802590378, -2.506131700382607352, 18.80026515017675592 ) ) ;
#917=CARTESIAN_POINT ( 'NONE',  ( 4.153440676704338586, -4.671190581744546932, 25.29954462468842635 ) ) ;
#921=CARTESIAN_POINT ( 'NONE',  ( -6.155854678529465218, 1.081900940642161135, 18.50425949503010159 ) ) ;
#924=CARTESIAN_POINT ( 'NONE',  ( -5.408775798201112650, 2.598833957129762950, 23.88602261056918152 ) ) ;
#932=FACE_BOUND ( 'NONE', #5455, .T. ) ;
#935=ORIENTED_EDGE ( 'NONE', *, *, #8740, .F. ) ;
#938=CARTESIAN_POINT ( 'NONE',  ( 3.922396193919027496, 4.541970110199465616, 30.12619317285289711 ) ) ;
#939=EDGE_CURVE ( 'NONE', #12601, #2089, #13670, .T. ) ;
#940=B_SPLINE_CURVE_WITH_KNOTS ( 'NONE', 3,
 ( #9001, #2705, #7790, #12637, #4049, #1737, #6532, #468, #12403, #8920, #7555, #11520, #1503, #11213, #2862, #10182, #4129, #4211 ),
 .UNSPECIFIED., .F., .F.,
 ( 4, 2, 2, 2, 2, 2, 2, 2, 4 ),
 ( 0.003131918686235973890, 0.003523310662250264159, 0.003914702638264553995, 0.004306094614278844698, 0.004697486590293134534, 0.005088878566307424370, 0.005480270542321714206, 0.005871662518336004041, 0.006263054494350294744 ),
 .UNSPECIFIED. ) ;
#942=CARTESIAN_POINT ( 'NONE',  ( -3.311384659207067038, -5.004923837169465983, 4.026414045633067040 ) ) ;
#943=EDGE_CURVE ( 'NONE', #2947, #7387, #83, .T. ) ;
#944=CARTESIAN_POINT ( 'NONE',  ( -4.286401442266607020, 4.198423832313117110, 31.00000000000000000 ) ) ;
#945=CARTESIAN_POINT ( 'NONE',  ( 5.915699123067176934, 1.003533581835446276, 17.49610204984016804 ) ) ;
#947=B_SPLINE_CURVE_WITH_KNOTS ( 'NONE', 3,
 ( #4040, #8914, #2855, #6525, #11512, #2696, #306, #1805, #5332, #6371, #9943, #10176, #7547, #15028, #12394, #6679, #11205, #5167 ),
 .UNSPECIFIED., .F., .F.,
 ( 4, 2, 2, 2, 2, 2, 2, 2, 4 ),
 ( 0.000000000000000000, 0.0003914898357794960857, 0.0007829796715589921715, 0.001174469507338488095, 0.001565959343117984343, 0.001957449178897481025, 0.002348939014676977924, 0.002740428850456474389, 0.003131918686235971288 ),
 .UNSPECIFIED. ) ;
#950=CARTESIAN_POINT ( 'NONE',  ( 4.286401442266545736, -4.198423832313181059, 11.36760611998364467 ) ) ;
#954=CARTESIAN_POINT ( 'NONE',  ( 2.817313151351089839, 5.579000502529481764, 31.00000000000000000 ) ) ;
#957=ORIENTED_EDGE ( 'NONE', *, *, #9756, .T. ) ;
#962=CYLINDRICAL_SURFACE ( 'NONE', #2245, 1.000000000000000888 ) ;
#965=CARTESIAN_POINT ( 'NONE',  ( 0.8002302970946603144, -5.947135855825864681, 4.386017732123007384 ) ) ;
#970=CARTESIAN_POINT ( 'NONE',  ( -7.180990026460747799, -3.384707322287517695, 5.000000000000004441 ) ) ;
#973=CARTESIAN_POINT ( 'NONE',  ( 3.459597053047906989, -5.206576120509703642, 30.02591457665829466 ) ) ;
#975=CARTESIAN_POINT ( 'NONE',  ( 5.940390500375535510, 6.474944468551633747, 31.00000000000000000 ) ) ;
#976=ADVANCED_FACE ( 'NONE', ( #7709 ), #3965, .F. ) ;
#979=CARTESIAN_POINT ( 'NONE',  ( 2.782468714962460510, -5.316055268221388630, 4.496102049840168036 ) ) ;
#982=CARTESIAN_POINT ( 'NONE',  ( 0.000000000000000000, 6.250000000000000888, 32.00000000000000000 ) ) ;
#983=CARTESIAN_POINT ( 'NONE',  ( 3.736691294293403409, -4.695920479336392894, 17.02641404563305372 ) ) ;
#985=ORIENTED_EDGE ( 'NONE', *, *, #7956, .T. ) ;
#986=CARTESIAN_POINT ( 'NONE',  ( 3.633127580202278661, -4.776802569231053397, 12.50007961174474502 ) ) ;
#988=AXIS2_PLACEMENT_3D ( 'NONE', #396, #13994, #10114 ) ;
#989=CARTESIAN_POINT ( 'NONE',  ( -0.7988860301920154283, -6.199427171881362497, 23.88455580536193423 ) ) ;
#991=CARTESIAN_POINT ( 'NONE',  ( 0.8002302970947927641, -5.947135855825846917, 17.38601773212298696 ) ) ;
#992=DIRECTION ( 'NONE',  ( 0.9510565162951500895, 0.3090169943749582204, 0.000000000000000000 ) ) ;
#993=EDGE_CURVE ( 'NONE', #12662, #9246, #11351, .T. ) ;
#994=CARTESIAN_POINT ( 'NONE',  ( 5.375913338529056062, 2.664979843780506563, 5.504289203620185589 ) ) ;
#997=CARTESIAN_POINT ( 'NONE',  ( 5.558508435838291462, -2.857531096718732400, 17.99999999999998934 ) ) ;
#1000=ORIENTED_EDGE ( 'NONE', *, *, #3749, .T. ) ;
#1001=CARTESIAN_POINT ( 'NONE',  ( -3.420311045507830272, 4.931422832349302787, 3.999920388255239434 ) ) ;
#1002=CARTESIAN_POINT ( 'NONE',  ( -0.9737778612004891476, -5.920671847850528025, 11.23736375884651473 ) ) ;
#1007=CARTESIAN_POINT ( 'NONE',  ( -5.409007216690667974, -2.598315788643760893, 30.38557478428061032 ) ) ;
#1012=CARTESIAN_POINT ( 'NONE',  ( 5.558508435838282580, 2.857531096718751940, 24.63234125634168237 ) ) ;
#1014=LINE ( 'NONE', #2445, #12121 ) ;
#1016=FACE_BOUND ( 'NONE', #8827, .T. ) ;
#1021=CARTESIAN_POINT ( 'NONE',  ( 5.665824935993652112, 1.978765057080799306, 23.50004946353776702 ) ) ;
#1022=VERTEX_POINT ( 'NONE', #10181 ) ;
#1024=CARTESIAN_POINT ( 'NONE',  ( 0.8738043859792735679, -6.188821459035850125, 25.00341560223748871 ) ) ;
#1025=CARTESIAN_POINT ( 'NONE',  ( -3.107688324358719889, 5.133887830459828550, 31.87378430870261425 ) ) ;
#1028=CARTESIAN_POINT ( 'NONE',  ( 3.736691294293317700, 4.695920479336459508, 18.97358595436693207 ) ) ;
#1030=CARTESIAN_POINT ( 'NONE',  ( 3.632753594129332964, -4.777047695050978149, 10.50004946353775281 ) ) ;
#1032=CARTESIAN_POINT ( 'NONE',  ( 0.1306394121199586922, -6.250000000000000888, 30.00000000000000355 ) ) ;
#1033=CARTESIAN_POINT ( 'NONE',  ( 5.375886393124341467, 2.665038680141373906, 4.495602393557859955 ) ) ;
#1034=CARTESIAN_POINT ( 'NONE',  ( -0.1323602877610810247, -6.000000000000004441, 18.99999999999998224 ) ) ;
#1036=VERTEX_POINT ( 'NONE', #6610 ) ;
#1039=B_SPLINE_CURVE_WITH_KNOTS ( 'NONE', 3,
 ( #8427, #10958, #13183, #15581, #2282, #6993, #5956, #10800, #15659, #4760, #9617, #56, #11822, #14456, #3636, #3559, #10642, #9375 ),
 .UNSPECIFIED., .F., .F.,
 ( 4, 2, 2, 2, 2, 2, 2, 2, 4 ),
 ( 0.000000000000000000, 0.0003914357524127484072, 0.0007828715048254968143, 0.001174307257238245330, 0.001565743009650993629, 0.001957178762063741927, 0.002348614514476490660, 0.002740050266889238959, 0.003131486019301987257 ),
 .UNSPECIFIED. ) ;
#1042=DIRECTION ( 'NONE',  ( 0.000000000000000000, 1.000000000000000000, 0.000000000000000000 ) ) ;
#1046=CARTESIAN_POINT ( 'NONE',  ( 6.172614129015243201, 0.9817721000788186547, 18.26236973443873168 ) ) ;
#1047=LINE ( 'NONE', #5910, #8971 ) ;
#1050=DIRECTION ( 'NONE',  ( -0.5877852522924685852, -0.8090169943749508930, 0.000000000000000000 ) ) ;
#1055=DIRECTION ( 'NONE',  ( -0.5877852522924685852, -0.8090169943749507819, 0.000000000000000000 ) ) ;
#1056=ORIENTED_EDGE ( 'NONE', *, *, #13482, .T. ) ;
#1058=ORIENTED_EDGE ( 'NONE', *, *, #6301, .F. ) ;
#1060=ORIENTED_EDGE ( 'NONE', *, *, #4196, .F. ) ;
#1062=CARTESIAN_POINT ( 'NONE',  ( -5.903061651806595478, -2.057626436184814001, 30.00008258189710730 ) ) ;
#1063=CARTESIAN_POINT ( 'NONE',  ( 3.632753594129279673, -4.777047695051020781, 17.00004946353776702 ) ) ;
#1064=CARTESIAN_POINT ( 'NONE',  ( -4.006441409774807560, -4.467329318258149939, 25.29888242247940155 ) ) ;
#1065=CARTESIAN_POINT ( 'NONE',  ( -5.558508435838177775, -2.857531096718951780, 31.13063932754212004 ) ) ;
#1066=CARTESIAN_POINT ( 'NONE',  ( -0.6144300524833572474, -6.220417338033053412, 4.200333721759340833 ) ) ;
#1067=EDGE_CURVE ( 'NONE', #2087, #12811, #1735, .T. ) ;
#1068=CARTESIAN_POINT ( 'NONE',  ( -3.923477796648549010, -4.541042560386451044, 12.37303779027049444 ) ) ;
#1071=CARTESIAN_POINT ( 'NONE',  ( -4.070863287254225860, -4.743975846881679281, 25.37305891554299819 ) ) ;
#1073=EDGE_CURVE ( 'NONE', #9955, #9045, #3815, .T. ) ;
#1077=CARTESIAN_POINT ( 'NONE',  ( 4.195842658231466515, 4.289229542213170987, 31.50439760644212939 ) ) ;
#1082=CARTESIAN_POINT ( 'NONE',  ( -2.849573632035255599, 5.280958870664612448, 4.384382673013949017 ) ) ;
#1083=CARTESIAN_POINT ( 'NONE',  ( 0.7993282387951774481, -5.947240459526499379, 12.11484358216955393 ) ) ;
#1085=ORIENTED_EDGE ( 'NONE', *, *, #3214, .F. ) ;
#1088=CARTESIAN_POINT ( 'NONE',  ( -2.668367453516768517, 5.373994336898062940, 11.36763921416086198 ) ) ;
#1091=CARTESIAN_POINT ( 'NONE',  ( -0.2623718222034988612, -6.245654667075783983, 30.02627829713834018 ) ) ;
#1093=CARTESIAN_POINT ( 'NONE',  ( 4.322356511625632614, 7.650514973136570696, 31.00000000000000000 ) ) ;
#1095=FACE_BOUND ( 'NONE', #9024, .T. ) ;
#1100=B_SPLINE_CURVE_WITH_KNOTS ( 'NONE', 3,
 ( #15536, #11940, #1046, #5909, #10445, #15299, #4401, #14090, #3200, #89, #15692, #249, #5109, #14813, #9962, #14737, #3898, #10831 ),
 .UNSPECIFIED., .F., .F.,
 ( 4, 2, 2, 2, 2, 2, 2, 2, 4 ),
 ( 0.003131486019301971645, 0.003522824630466680519, 0.003914163241631389394, 0.004305501852796097401, 0.004696840463960806275, 0.005088179075125515149, 0.005479517686290224024, 0.005870856297454932898, 0.006262194908619641773 ),
 .UNSPECIFIED. ) ;
#1103=ORIENTED_EDGE ( 'NONE', *, *, #7106, .F. ) ;
#1104=AXIS2_PLACEMENT_3D ( 'NONE', #3980, #8858, #13769 ) ;
#1105=DIRECTION ( 'NONE',  ( 0.000000000000000000, 0.000000000000000000, 1.000000000000000000 ) ) ;
#1106=CARTESIAN_POINT ( 'NONE',  ( 0.9735954530127236550, -6.173909381473960956, 24.76281793585244628 ) ) ;
#1109=CARTESIAN_POINT ( 'NONE',  ( 2.848235266350879868, 5.281699484015724089, 18.61397738943081848 ) ) ;
#1111=CARTESIAN_POINT ( 'NONE',  ( -0.6156307853269342711, -5.969051238897256972, 31.79870573410679313 ) ) ;
#1112=B_SPLINE_CURVE_WITH_KNOTS ( 'NONE', 3,
 ( #10937, #12359, #3768, #11248, #11013, #7669, #35, #114, #4901, #1455, #8798, #9830, #7361, #13551, #2660, #9986, #7513, #12280 ),
 .UNSPECIFIED., .F., .F.,
 ( 4, 2, 2, 2, 2, 2, 2, 2, 4 ),
 ( 0.003131486019301987257, 0.003522824630466693963, 0.003914163241631400669, 0.004305501852796107809, 0.004696840463960814081, 0.005088179075125520354, 0.005479517686290227493, 0.005870856297454934633, 0.006262194908619640905 ),
 .UNSPECIFIED. ) ;
#1114=CARTESIAN_POINT ( 'NONE',  ( 0.5039005892421511978, -6.230833003620539046, 30.12636388911297658 ) ) ;
#1116=CARTESIAN_POINT ( 'NONE',  ( -5.317509234263960494, 2.779225709350992890, 30.86935038651144936 ) ) ;
#1117=ORIENTED_EDGE ( 'NONE', *, *, #6253, .T. ) ;
#1119=VERTEX_POINT ( 'NONE', #5492 ) ;
#1120=CARTESIAN_POINT ( 'NONE',  ( 1.353717517954364224E-13, -6.250000000000000888, 17.99999999999998934 ) ) ;
#1121=VERTEX_POINT ( 'NONE', #10336 ) ;
#1123=CARTESIAN_POINT ( 'NONE',  ( -5.726307184802615247, -2.506131700382550065, 12.30026515017674882 ) ) ;
#1124=CARTESIAN_POINT ( 'NONE',  ( 4.286401442266544848, -4.198423832313181059, 11.49999999999998224 ) ) ;
#1127=EDGE_CURVE ( 'NONE', #9974, #8460, #9583, .T. ) ;
#1130=FACE_OUTER_BOUND ( 'NONE', #3700, .T. ) ;
#1132=CARTESIAN_POINT ( 'NONE',  ( 5.558508435838189321, 2.857531096718932684, 5.132341256341690361 ) ) ;
#1135=CARTESIAN_POINT ( 'NONE',  ( 7.799024015210652472, -1.482594289697024781, 11.49999999999998224 ) ) ;
#1138=CARTESIAN_POINT ( 'NONE',  ( 0.8738239080080443255, 6.188820299975592576, 31.50355795710145657 ) ) ;
#1141=CARTESIAN_POINT ( 'NONE',  ( -3.312341048453529169, -5.004306261885416163, 25.47398020122239259 ) ) ;
#1142=CARTESIAN_POINT ( 'NONE',  ( 2.668367453516647281, -5.373994336898124224, 11.63061695532137385 ) ) ;
#1144=CARTESIAN_POINT ( 'NONE',  ( 3.922288969639628586, 4.542045818322656636, 25.37378430870261781 ) ) ;
#1146=CARTESIAN_POINT ( 'NONE',  ( -2.841519077896198731, -5.566940434249990410, 18.26379616840806008 ) ) ;
#1147=CARTESIAN_POINT ( 'NONE',  ( 5.903347812666343231, 1.076697810262630783, 30.38602261056917442 ) ) ;
#1153=CARTESIAN_POINT ( 'NONE',  ( -5.558508435838179551, -2.857531096718951336, 31.00000000000000000 ) ) ;
#1155=CARTESIAN_POINT ( 'NONE',  ( -4.435347140101170815, 4.403429997944372509, 17.99999999999998934 ) ) ;
#1159=CARTESIAN_POINT ( 'NONE',  ( 3.253823204785200485, -5.337590213880453405, 31.87305891554300530 ) ) ;
#1161=VERTEX_POINT ( 'NONE', #15348 ) ;
#1162=CARTESIAN_POINT ( 'NONE',  ( 4.153440676704287071, 4.671190581744593118, 23.70045537531157720 ) ) ;
#1167=CARTESIAN_POINT ( 'NONE',  ( -5.648794263291763151, 2.676232015153579447, 12.11441947245483064 ) ) ;
#1169=CARTESIAN_POINT ( 'NONE',  ( 6.768587589771821120E-14, -6.250000000000000888, 11.49999999999998224 ) ) ;
#1172=CARTESIAN_POINT ( 'NONE',  ( 0.6156307853269756825, 5.969051238897252532, 31.79870573410680024 ) ) ;
#1173=VECTOR ( 'NONE', #15159, 1000.000000000000114 ) ;
#1174=ORIENTED_EDGE ( 'NONE', *, *, #15351, .F. ) ;
#1177=CARTESIAN_POINT ( 'NONE',  ( -4.070863287254119278, -4.743975846881772540, 12.37305891554299286 ) ) ;
#1181=CARTESIAN_POINT ( 'NONE',  ( 5.616089948629732653, -2.743103014345535939, 31.50436969680151833 ) ) ;
#1182=DIRECTION ( 'NONE',  ( 0.9510565162951500895, 0.3090169943749582204, 0.000000000000000000 ) ) ;
#1183=CARTESIAN_POINT ( 'NONE',  ( -0.5030929395819625505, -6.230885867001150658, 10.62600319116547887 ) ) ;
#1184=CARTESIAN_POINT ( 'NONE',  ( 2.668367453516689025, -5.373994336898102908, 30.86935038651144936 ) ) ;
#1186=LINE ( 'NONE', #11515, #5034 ) ;
#1187=CARTESIAN_POINT ( 'NONE',  ( 5.665824935993619249, -1.978765057080893008, 31.99995053646223653 ) ) ;
#1188=CARTESIAN_POINT ( 'NONE',  ( -4.416678568553713546, 4.422441866694247103, 30.73763026556126121 ) ) ;
#1189=CARTESIAN_POINT ( 'NONE',  ( 5.620786884546266293, 2.102685372472950398, 4.026414045633067929 ) ) ;
#1195=CYLINDRICAL_SURFACE ( 'NONE', #1471, 1.000000000000000666 ) ;
#1198=CARTESIAN_POINT ( 'NONE',  ( 0.2624013748573172378, 5.995472630654518298, 4.026285596910829767 ) ) ;
#1199=FACE_OUTER_BOUND ( 'NONE', #10909, .T. ) ;
#1204=CARTESIAN_POINT ( 'NONE',  ( -5.665308849928837986, 1.980336949702462990, 31.99992002356261267 ) ) ;
#1207=DIRECTION ( 'NONE',  ( 0.5877852522924802425, -0.8090169943749422332, 0.000000000000000000 ) ) ;
#1210=ORIENTED_EDGE ( 'NONE', *, *, #2448, .T. ) ;
#1211=ORIENTED_EDGE ( 'NONE', *, *, #8936, .F. ) ;
#1212=LINE ( 'NONE', #9499, #3758 ) ;
#1217=CARTESIAN_POINT ( 'NONE',  ( -6.172552660730963758, 0.9821660343539665439, 24.76379616840807074 ) ) ;
#1220=CARTESIAN_POINT ( 'NONE',  ( -2.668367453516813814, -5.373994336898041624, 24.49999999999999289 ) ) ;
#1221=CARTESIAN_POINT ( 'NONE',  ( -6.142908455506939980, -1.155755562476076692, 31.61517780375841369 ) ) ;
#1222=CARTESIAN_POINT ( 'NONE',  ( 2.996417732210474583, -5.485687819086957795, 23.88603820591927729 ) ) ;
#1224=CARTESIAN_POINT ( 'NONE',  ( -3.255013540813683992, -5.336859797930807225, 18.87381964045070504 ) ) ;
#1229=VECTOR ( 'NONE', #2016, 1000.000000000000000 ) ;
#1232=CARTESIAN_POINT ( 'NONE',  ( 5.558508435838260375, -2.857531096718793240, 11.49999999999998224 ) ) ;
#1233=B_SPLINE_CURVE_WITH_KNOTS ( 'NONE', 3,
 ( #13622, #9902, #1686, #2656, #11242, #3997, #2735, #7587, #14990, #4081, #12434, #8952, #344, #5206, #10059, #7664, #13783, #3047 ),
 .UNSPECIFIED., .F., .F.,
 ( 4, 2, 2, 2, 2, 2, 2, 2, 4 ),
 ( 0.000000000000000000, 0.0003914904498596246838, 0.0007829808997192493677, 0.001174471349578873943, 0.001565961799438498735, 0.001957452249298123528, 0.002348942699157747886, 0.002740433149017372678, 0.003131923598876997471 ),
 .UNSPECIFIED. ) ;
#1234=ADVANCED_FACE ( 'NONE', ( #11755 ), #14216, .F. ) ;
#1236=ORIENTED_EDGE ( 'NONE', *, *, #9801, .T. ) ;
#1237=CARTESIAN_POINT ( 'NONE',  ( -5.409007216690679520, 2.598315788643733804, 12.11442521571935949 ) ) ;
#1238=CARTESIAN_POINT ( 'NONE',  ( 6.768587589771821120E-14, -6.000000000000000888, 12.49999999999998401 ) ) ;
#1239=CARTESIAN_POINT ( 'NONE',  ( 5.330189595673696878, 2.755293208590127385, 24.76382603205595956 ) ) ;
#1241=FACE_OUTER_BOUND ( 'NONE', #4971, .T. ) ;
#1243=CARTESIAN_POINT ( 'NONE',  ( 3.158296126777660362, 5.394094919772187247, 23.70112161576660981 ) ) ;
#1245=CARTESIAN_POINT ( 'NONE',  ( -2.817313151351372724, 5.579000502529339656, 24.36765874365829987 ) ) ;
#1246=CARTESIAN_POINT ( 'NONE',  ( 2.082642335314403343E-14, -6.250000000000000888, 32.00000000000000000 ) ) ;
#1251=CARTESIAN_POINT ( 'NONE',  ( 0.9739805876848109945, 5.920636045238163447, 31.26171386814423414 ) ) ;
#1252=VERTEX_POINT ( 'NONE', #5319 ) ;
#1255=DIRECTION ( 'NONE',  ( 0.000000000000000000, 0.000000000000000000, 1.000000000000000000 ) ) ;
#1256=ORIENTED_EDGE ( 'NONE', *, *, #12219, .T. ) ;
#1261=DIRECTION ( 'NONE',  ( 0.8090169943749506709, -0.5877852522924689183, 0.000000000000000000 ) ) ;
#1263=CARTESIAN_POINT ( 'NONE',  ( 4.142173849413661735, 4.341773579105486114, 18.61519382448850024 ) ) ;
#1266=CARTESIAN_POINT ( 'NONE',  ( 5.935543223013869607, -0.8771126767605967878, 11.49999999999998224 ) ) ;
#1267=CARTESIAN_POINT ( 'NONE',  ( -4.070863287254157470, 4.743975846881738789, 30.12694108445699825 ) ) ;
#1268=CARTESIAN_POINT ( 'NONE',  ( -6.176542424588110869, 0.9554180641286129649, 11.49999999999998224 ) ) ;
#1269=CARTESIAN_POINT ( 'NONE',  ( -5.666074146198023520, 1.978051345703084385, 29.99995067926688819 ) ) ;
#1275=CARTESIAN_POINT ( 'NONE',  ( -5.621278735166150398, -2.101423246382678744, 25.47408052783099919 ) ) ;
#1276=B_SPLINE_CURVE_WITH_KNOTS ( 'NONE', 3,
 ( #2879, #12420, #7725, #4143, #9093, #13690, #1753, #3903, #8778, #2799, #1830, #3034, #7887, #5354, #10200, #15051, #6704, #1518 ),
 .UNSPECIFIED., .F., .F.,
 ( 4, 2, 2, 2, 2, 2, 2, 2, 4 ),
 ( 0.003131918686235972155, 0.003523310662250262858, 0.003914702638264553128, 0.004306094614278843831, 0.004697486590293134534, 0.005088878566307425237, 0.005480270542321715940, 0.005871662518336006643, 0.006263054494350297347 ),
 .UNSPECIFIED. ) ;
#1277=ORIENTED_EDGE ( 'NONE', *, *, #7956, .F. ) ;
#1279=CARTESIAN_POINT ( 'NONE',  ( -5.558508435838157347, -2.857531096718993080, 11.49999999999998224 ) ) ;
#1280=CARTESIAN_POINT ( 'NONE',  ( -7.490007020835699691, -2.433650805992386701, 31.00000000000000000 ) ) ;
#1283=CARTESIAN_POINT ( 'NONE',  ( -5.935543223013858949, 0.8771126767606858277, 31.13236078583911137 ) ) ;
#1285=CARTESIAN_POINT ( 'NONE',  ( -5.726307184802553962, -2.506131700382691285, 25.30026515017674882 ) ) ;
#1287=CARTESIAN_POINT ( 'NONE',  ( 4.435347140101058905, -4.403429997944484420, 31.00000000000000000 ) ) ;
#1289=CARTESIAN_POINT ( 'NONE',  ( 5.649200442566134406, 2.675373855294195913, 5.615601928929211617 ) ) ;
#1292=ORIENTED_EDGE ( 'NONE', *, *, #15126, .F. ) ;
#1293=ORIENTED_EDGE ( 'NONE', *, *, #3939, .T. ) ;
#1295=CARTESIAN_POINT ( 'NONE',  ( 0.9740856415300854776, -6.173834621338593287, 4.738526530555332350 ) ) ;
#1296=CARTESIAN_POINT ( 'NONE',  ( -6.105861027178969280, 1.337741388556907385, 31.79954462468843346 ) ) ;
#1297=CARTESIAN_POINT ( 'NONE',  ( 1.000079958708202321, 5.916066267613690144, 11.63152738882033788 ) ) ;
#1298=CARTESIAN_POINT ( 'NONE',  ( 7.347880794884119736E-16, -6.250000000000000888, 4.000000000000004441 ) ) ;
#1299=CARTESIAN_POINT ( 'NONE',  ( 5.317509234264001350, -2.779225709350912954, 11.49999999999998224 ) ) ;
#1300=CARTESIAN_POINT ( 'NONE',  ( 0.9740807849837530563, -5.920620690450666856, 17.73850119700669481 ) ) ;
#1304=B_SPLINE_CURVE_WITH_KNOTS ( 'NONE', 3,
 ( #10279, #6478, #11312, #5359, #489, #7967, #5279, #8863, #7654, #4148, #10050, #13926, #14898, #4227, #13847, #3037, #566, #2960 ),
 .UNSPECIFIED., .F., .F.,
 ( 4, 2, 2, 2, 2, 2, 2, 2, 4 ),
 ( 0.000000000000000000, 0.0003914898357794971157, 0.0007829796715589942314, 0.001174469507338491347, 0.001565959343117988463, 0.001957449178897485362, 0.002348939014676982694, 0.002740428850456480027, 0.003131918686235976926 ),
 .UNSPECIFIED. ) ;
#1309=EDGE_LOOP ( 'NONE', ( #10925, #13095 ) ) ;
#1310=CARTESIAN_POINT ( 'NONE',  ( 0.000000000000000000, 0.000000000000000000, 36.00000000000000711 ) ) ;
#1311=CARTESIAN_POINT ( 'NONE',  ( -0.5031281619707089758, -5.980084330432673845, 10.62602272744524079 ) ) ;
#1313=CARTESIAN_POINT ( 'NONE',  ( 4.153440676704482470, -4.671190581744419035, 31.79954462468844056 ) ) ;
#1317=CARTESIAN_POINT ( 'NONE',  ( -3.312341048453488312, 5.004306261885441032, 10.52601979877758964 ) ) ;
#1323=FACE_BOUND ( 'NONE', #11390, .T. ) ;
#1327=VECTOR ( 'NONE', #1359, 1000.000000000000000 ) ;
#1328=CARTESIAN_POINT ( 'NONE',  ( 5.858736126997162508, 2.179962889276984228, 17.02640428276697904 ) ) ;
#1330=ORIENTED_EDGE ( 'NONE', *, *, #2807, .T. ) ;
#1333=CARTESIAN_POINT ( 'NONE',  ( 5.486982057989233219, 2.429327048029787051, 23.70068193741825269 ) ) ;
#1334=CARTESIAN_POINT ( 'NONE',  ( 4.141923667210567039, -4.342011609040540954, 25.11561732698605098 ) ) ;
#1335=ORIENTED_EDGE ( 'NONE', *, *, #5940, .T. ) ;
#1336=CARTESIAN_POINT ( 'NONE',  ( -4.267992336621275307, -4.217442018459924391, 24.23805675996853992 ) ) ;
#1337=CARTESIAN_POINT ( 'NONE',  ( 0.1306394121201409075, -6.249999999999997335, 23.50000000000000000 ) ) ;
#1339=CARTESIAN_POINT ( 'NONE',  ( 6.081590040723082957, -1.446205118472983164, 31.87367328635992081 ) ) ;
#1341=CARTESIAN_POINT ( 'NONE',  ( -1.000082492230644826, -6.169467968613719044, 11.63152538105391365 ) ) ;
#1342=CARTESIAN_POINT ( 'NONE',  ( 5.531796221294958293, -2.326749136277022512, 25.37378430870261781 ) ) ;
#1345=CARTESIAN_POINT ( 'NONE',  ( 5.935543223013868719, -0.8771126767605967878, 11.36938304467859773 ) ) ;
#1346=CARTESIAN_POINT ( 'NONE',  ( -5.531623157106168698, 2.327208526676430189, 10.62635295315575235 ) ) ;
#1349=CARTESIAN_POINT ( 'NONE',  ( 3.106366801611825768, 5.134708448381389623, 23.62696220972947359 ) ) ;
#1352=EDGE_LOOP ( 'NONE', ( #15708, #4672 ) ) ;
#1354=ORIENTED_EDGE ( 'NONE', *, *, #6985, .F. ) ;
#1357=CARTESIAN_POINT ( 'NONE',  ( -6.142908455506926657, -1.155755562476141973, 12.11517780375842790 ) ) ;
#1358=CARTESIAN_POINT ( 'NONE',  ( 6.176542424588128632, -0.9554180641284775177, 11.49999999999998224 ) ) ;
#1359=DIRECTION ( 'NONE',  ( 0.5877852522924802425, -0.8090169943749422332, 0.000000000000000000 ) ) ;
#1360=VECTOR ( 'NONE', #9407, 1000.000000000000000 ) ;
#1362=CARTESIAN_POINT ( 'NONE',  ( 5.558508435838229289, -2.857531096718853192, 4.867658743658316745 ) ) ;
#1364=DIRECTION ( 'NONE',  ( 0.9510565162951499785, 0.3090169943749582204, 0.000000000000000000 ) ) ;
#1366=ADVANCED_FACE ( 'NONE', ( #7460, #12303 ), #1401, .F. ) ;
#1367=CARTESIAN_POINT ( 'NONE',  ( -5.648559266344550522, 2.676764518775886170, 30.38603820591929505 ) ) ;
#1372=EDGE_LOOP ( 'NONE', ( #10888, #2354, #4868, #12038 ) ) ;
#1373=CARTESIAN_POINT ( 'NONE',  ( 5.317509234263979145, -2.779225709350955142, 31.00000000000000000 ) ) ;
#1375=CARTESIAN_POINT ( 'NONE',  ( -5.769755079862245672, -2.405651898699154412, 17.12694108445698760 ) ) ;
#1376=CARTESIAN_POINT ( 'NONE',  ( -3.736532060718029680, -4.696070028785941375, 18.97377823943292086 ) ) ;
#1377=CARTESIAN_POINT ( 'NONE',  ( 0.2624013748573880700, 5.995472630654516522, 10.52628559691080845 ) ) ;
#1380=CARTESIAN_POINT ( 'NONE',  ( -5.770167736194696140, -2.404664418229167655, 5.873673286359928802 ) ) ;
#1381=CARTESIAN_POINT ( 'NONE',  ( 0.1306497350719363348, -5.999999999999997335, 23.50000000000000000 ) ) ;
#1389=CARTESIAN_POINT ( 'NONE',  ( -6.176542424588090441, 0.9554180641287483011, 24.36762589283695135 ) ) ;
#1391=DIRECTION ( 'NONE',  ( -0.3090169943749584425, 0.9510565162951498674, 0.000000000000000000 ) ) ;
#1395=CARTESIAN_POINT ( 'NONE',  ( 5.409423237179020738, -2.597448116731011947, 4.384382673013947240 ) ) ;
#1396=CARTESIAN_POINT ( 'NONE',  ( -7.799024015210601846, -1.482594289697409140, 24.49999999999999289 ) ) ;
#1399=ADVANCED_FACE ( 'NONE', ( #6747 ), #5475, .F. ) ;
#1401=PLANE ( 'NONE',  #12108 ) ;
#1403=ORIENTED_EDGE ( 'NONE', *, *, #13029, .F. ) ;
#1404=DIRECTION ( 'NONE',  ( 0.000000000000000000, 1.000000000000000000, 0.000000000000000000 ) ) ;
#1406=CARTESIAN_POINT ( 'NONE',  ( -5.935543223013825198, -0.8771126767608831143, 18.13239388001634467 ) ) ;
#1407=CARTESIAN_POINT ( 'NONE',  ( 4.416397290909897855, 4.422724436066440390, 30.73620383159192215 ) ) ;
#1409=ADVANCED_FACE ( 'NONE', ( #4503, #5705, #527, #5395, #4349, #9206, #7924, #10317, #1794, #12767, #9284, #13968, #15328, #15170, #12928, #9134, #10243, #4269, #10549, #15094, #6591, #676, #5627, #9359, #14044, #3153 ), #13886, .F. ) ;
#1410=CYLINDRICAL_SURFACE ( 'NONE', #10422, 1.000000000000000888 ) ;
#1411=CARTESIAN_POINT ( 'NONE',  ( 5.570760634536836342, -2.834026536768180282, 11.76225281721714389 ) ) ;
#1413=CARTESIAN_POINT ( 'NONE',  ( 0.6156133477427008227, 6.220296490279941359, 12.29872387345513474 ) ) ;
#1414=CARTESIAN_POINT ( 'NONE',  ( -0.1306070469492700281, -6.250000000000000888, 10.49999999999998579 ) ) ;
#1415=CARTESIAN_POINT ( 'NONE',  ( 5.375886393124466700, -2.665038680141120331, 25.00439760644211873 ) ) ;
#1419=CARTESIAN_POINT ( 'NONE',  ( 2.668367453516707233, -5.373994336898093138, 5.000000000000004441 ) ) ;
#1420=CARTESIAN_POINT ( 'NONE',  ( -5.915653884842710930, 1.003805156977417345, 10.99560239355786351 ) ) ;
#1422=DIRECTION ( 'NONE',  ( 0.5877852522924802425, -0.8090169943749422332, 0.000000000000000000 ) ) ;
#1423=VERTEX_POINT ( 'NONE', #10398 ) ;
#1426=VERTEX_POINT ( 'NONE', #8007 ) ;
#1428=ORIENTED_EDGE ( 'NONE', *, *, #582, .F. ) ;
#1429=CARTESIAN_POINT ( 'NONE',  ( -3.420659742068546283, 4.931142898501624572, 25.49995053646222232 ) ) ;
#1430=EDGE_LOOP ( 'NONE', ( #1210, #12509 ) ) ;
#1435=DIRECTION ( 'NONE',  ( -0.3090169943749584425, 0.9510565162951498674, 0.000000000000000000 ) ) ;
#1438=CARTESIAN_POINT ( 'NONE',  ( 4.005785023174503579, -4.467917056767357842, 31.79952054102714598 ) ) ;
#1442=EDGE_LOOP ( 'NONE', ( #5750, #13383 ) ) ;
#1443=ORIENTED_EDGE ( 'NONE', *, *, #8639, .T. ) ;
#1445=CARTESIAN_POINT ( 'NONE',  ( 5.317509234263979145, -2.779225709350955142, 30.86763921416088863 ) ) ;
#1448=CARTESIAN_POINT ( 'NONE',  ( 5.770331821586418108, -2.404225004693562262, 31.87380055247395561 ) ) ;
#1449=CARTESIAN_POINT ( 'NONE',  ( 0.2623718222035119063, 6.245654667075785760, 4.026278297138354390 ) ) ;
#1450=EDGE_CURVE ( 'NONE', #2495, #15690, #4190, .T. ) ;
#1451=CARTESIAN_POINT ( 'NONE',  ( -3.107583187530470248, -5.133966411712660438, 18.87380682714710289 ) ) ;
#1452=CARTESIAN_POINT ( 'NONE',  ( 4.435347140100928343, -4.403429997944614982, 24.49999999999999289 ) ) ;
#1455=CARTESIAN_POINT ( 'NONE',  ( -5.984759433607032442, 1.806271833852219899, 6.000082193215567905 ) ) ;
#1456=CARTESIAN_POINT ( 'NONE',  ( -2.997451966578549065, 5.485105005465932493, 18.61517780375842790 ) ) ;
#1458=EDGE_CURVE ( 'NONE', #6001, #1465, #12776, .T. ) ;
#1465=VERTEX_POINT ( 'NONE', #997 ) ;
#1466=CARTESIAN_POINT ( 'NONE',  ( -5.935543223013850955, 0.8771126767607324570, 11.49999999999998224 ) ) ;
#1469=CARTESIAN_POINT ( 'NONE',  ( 6.081590040723058976, 1.446205118473078199, 30.12632671364006143 ) ) ;
#1471=AXIS2_PLACEMENT_3D ( 'NONE', #9482, #10912, #7021 ) ;
#1472=EDGE_CURVE ( 'NONE', #10038, #12139, #7103, .T. ) ;
#1474=AXIS2_PLACEMENT_3D ( 'NONE', #10490, #14056, #15344 ) ;
#1476=CARTESIAN_POINT ( 'NONE',  ( -2.668367453516648169, -5.373994336898123336, 31.00000000000000000 ) ) ;
#1477=FACE_OUTER_BOUND ( 'NONE', #11688, .T. ) ;
#1485=CARTESIAN_POINT ( 'NONE',  ( 6.176542424588140179, -0.9554180641284089059, 17.99999999999998934 ) ) ;
#1489=CARTESIAN_POINT ( 'NONE',  ( -4.267992336621228233, -4.217442018459970576, 17.73805675996853637 ) ) ;
#1490=EDGE_CURVE ( 'NONE', #12426, #567, #3524, .T. ) ;
#1492=CARTESIAN_POINT ( 'NONE',  ( 6.172651332693098958, -0.9815532474593492429, 31.26190213084010949 ) ) ;
#1494=CARTESIAN_POINT ( 'NONE',  ( -0.5042675786778498814, -6.230788509548846221, 12.37331068310445836 ) ) ;
#1496=CARTESIAN_POINT ( 'NONE',  ( 3.106366801611882611, 5.134708448381354984, 17.12696220972948069 ) ) ;
#1501=CARTESIAN_POINT ( 'NONE',  ( -2.841519077896177858, 5.566940434250000180, 30.73620383159193281 ) ) ;
#1502=CARTESIAN_POINT ( 'NONE',  ( -5.842945980534642203, -1.369128644668982542, 12.37378430870260537 ) ) ;
#1503=CARTESIAN_POINT ( 'NONE',  ( -5.866923913994629203, -1.260079467906603634, 10.70047945897284158 ) ) ;
#1504=EDGE_LOOP ( 'NONE', ( #9820, #5203, #3418, #12305 ) ) ;
#1506=ORIENTED_EDGE ( 'NONE', *, *, #1759, .T. ) ;
#1508=( GEOMETRIC_REPRESENTATION_CONTEXT ( 3 ) GLOBAL_UNCERTAINTY_ASSIGNED_CONTEXT ( ( #10618 ) ) GLOBAL_UNIT_ASSIGNED_CONTEXT ( ( #14072, #5503, #3106 ) ) REPRESENTATION_CONTEXT ( 'NONE', 'WORKASPACE' ) );
#1510=CARTESIAN_POINT ( 'NONE',  ( -5.866984344570797205, -1.259800266528794843, 25.29931806258175087 ) ) ;
#1512=VERTEX_POINT ( 'NONE', #1232 ) ;
#1514=CARTESIAN_POINT ( 'NONE',  ( 0.9737778612005509871, 5.920671847850518255, 4.737363758846515616 ) ) ;
#1518=CARTESIAN_POINT ( 'NONE',  ( -2.668367453516831134, 5.373994336898032742, 17.99999999999998934 ) ) ;
#1523=CARTESIAN_POINT ( 'NONE',  ( 5.558508435838260375, -2.857531096718793240, 11.49999999999998224 ) ) ;
#1525=EDGE_CURVE ( 'NONE', #13850, #13656, #6944, .T. ) ;
#1526=ORIENTED_EDGE ( 'NONE', *, *, #2897, .T. ) ;
#1527=EDGE_LOOP ( 'NONE', ( #2291, #5119 ) ) ;
#1529=ORIENTED_EDGE ( 'NONE', *, *, #11347, .T. ) ;
#1530=CARTESIAN_POINT ( 'NONE',  ( 0.7995298244855962855, 5.947211616899230613, 18.61456014619857413 ) ) ;
#1533=CARTESIAN_POINT ( 'NONE',  ( -5.984759433606969381, -1.806271833852430397, 16.99991780678442410 ) ) ;
#1534=CARTESIAN_POINT ( 'NONE',  ( -4.142620314836390705, -4.341347824677495026, 18.61442521571937192 ) ) ;
#1535=EDGE_CURVE ( 'NONE', #2787, #6307, #4658, .T. ) ;
#1537=CARTESIAN_POINT ( 'NONE',  ( 0.9999171162591148354, 6.169494774098524204, 17.86722320330678215 ) ) ;
#1539=PRESENTATION_STYLE_ASSIGNMENT (( #6491 ) ) ;
#1540=DIRECTION ( 'NONE',  ( 0.000000000000000000, 1.000000000000000000, 0.000000000000000000 ) ) ;
#1541=CARTESIAN_POINT ( 'NONE',  ( -4.416837305303601191, 4.422286678978908370, 18.26190213084011660 ) ) ;
#1549=CARTESIAN_POINT ( 'NONE',  ( -6.021167129161051790, 1.680051667990315023, 17.02640428276697904 ) ) ;
#1550=CARTESIAN_POINT ( 'NONE',  ( -6.105925084677665815, 1.337450587213249165, 23.70066851092423477 ) ) ;
#1552=CARTESIAN_POINT ( 'NONE',  ( 6.155912734541118425, 1.081577393120980224, 30.49610786875027912 ) ) ;
#1554=CARTESIAN_POINT ( 'NONE',  ( -3.255013540813579187, -5.336859797930871174, 31.87381964045071214 ) ) ;
#1555=ADVANCED_FACE ( 'NONE', ( #6762 ), #12860, .F. ) ;
#1557=CARTESIAN_POINT ( 'NONE',  ( 5.317509234263970264, -2.779225709350972906, 5.000000000000004441 ) ) ;
#1559=CARTESIAN_POINT ( 'NONE',  ( -2.817313151351126699, -5.579000502529464001, 30.86762589283693359 ) ) ;
#1564=EDGE_CURVE ( 'NONE', #1161, #1036, #8266, .T. ) ;
#1568=CARTESIAN_POINT ( 'NONE',  ( -5.317509234263866347, -2.779225709351170970, 18.13064961348854709 ) ) ;
#1571=CARTESIAN_POINT ( 'NONE',  ( -3.107688324358743426, -5.133887830459814339, 17.12621569129736798 ) ) ;
#1574=CARTESIAN_POINT ( 'NONE',  ( 4.322356511625632614, 7.650514973136570696, 31.00000000000000000 ) ) ;
#1579=CARTESIAN_POINT ( 'NONE',  ( 4.322356511625649489, 7.650514973136559149, 5.000000000000004441 ) ) ;
#1580=CARTESIAN_POINT ( 'NONE',  ( -5.329907877631328006, -2.755840666746313339, 11.76194324003145475 ) ) ;
#1581=FACE_OUTER_BOUND ( 'NONE', #15550, .T. ) ;
#1584=VERTEX_POINT ( 'NONE', #4207 ) ;
#1585=CARTESIAN_POINT ( 'NONE',  ( -5.931734679891415674, -0.9039278060246241919, 24.23617396794404044 ) ) ;
#1587=AXIS2_PLACEMENT_3D ( 'NONE', #5525, #1773, #9037 ) ;
#1588=CARTESIAN_POINT ( 'NONE',  ( -5.903119516422441038, -1.077859910107684227, 25.11519382448850379 ) ) ;
#1592=CARTESIAN_POINT ( 'NONE',  ( -1.000049560716421482, 5.916071405810168216, 17.86967799011532776 ) ) ;
#1594=CARTESIAN_POINT ( 'NONE',  ( 6.123233995736766282E-16, -6.250000000000000888, 6.000000000000005329 ) ) ;
#1596=CARTESIAN_POINT ( 'NONE',  ( -4.143041610105331785, -4.340967609747012013, 10.88602261056916021 ) ) ;
#1597=CARTESIAN_POINT ( 'NONE',  ( -6.021167129161005604, -1.680051667990481779, 25.47359571723300320 ) ) ;
#1599=VECTOR ( 'NONE', #719, 1000.000000000000114 ) ;
#1600=CARTESIAN_POINT ( 'NONE',  ( -5.726307184802663208, 2.506131700382440819, 30.19973484982324763 ) ) ;
#1602=ORIENTED_EDGE ( 'NONE', *, *, #12992, .T. ) ;
#1611=CARTESIAN_POINT ( 'NONE',  ( -2.668367453516752530, -5.373994336898073598, 18.13236078583909361 ) ) ;
#1612=CARTESIAN_POINT ( 'NONE',  ( -3.158825713737541729, 5.393784879207139227, 31.79933148907577234 ) ) ;
#1613=CARTESIAN_POINT ( 'NONE',  ( 2.817313151350985034, 5.579000502529534167, 17.99999999999998934 ) ) ;
#1617=CARTESIAN_POINT ( 'NONE',  ( 5.935543223013866942, 0.8771126767606117758, 17.99999999999998934 ) ) ;
#1625=CARTESIAN_POINT ( 'NONE',  ( -2.692215568229806788, 5.362327947133613826, 5.262290378359323562 ) ) ;
#1628=CARTESIAN_POINT ( 'NONE',  ( -5.558508435838219519, 2.857531096718872732, 31.00000000000000000 ) ) ;
#1629=CARTESIAN_POINT ( 'NONE',  ( -3.312341048453600667, 5.004306261885368201, 23.52601979877760385 ) ) ;
#1630=CARTESIAN_POINT ( 'NONE',  ( 0.1323602877614195317, 5.999999999999997335, 25.50000000000000355 ) ) ;
#1632=CARTESIAN_POINT ( 'NONE',  ( 4.153663429050769906, 4.670992970568382141, 5.799331489075774115 ) ) ;
#1640=EDGE_CURVE ( 'NONE', #8395, #9339, #1014, .T. ) ;
#1641=CARTESIAN_POINT ( 'NONE',  ( -4.416837305303488392, -4.422286678979018504, 11.23809786915986564 ) ) ;
#1644=CARTESIAN_POINT ( 'NONE',  ( 5.616089948629791273, -2.743103014345418700, 18.50436969680152899 ) ) ;
#1646=ORIENTED_EDGE ( 'NONE', *, *, #2416, .F. ) ;
#1648=CYLINDRICAL_SURFACE ( 'NONE', #15697, 1.000000000000000444 ) ;
#1651=DIRECTION ( 'NONE',  ( 1.000000000000000000, 0.000000000000000000, 0.000000000000000000 ) ) ;
#1655=CARTESIAN_POINT ( 'NONE',  ( 4.286401442266591921, -4.198423832313132209, 5.000000000000004441 ) ) ;
#1656=CARTESIAN_POINT ( 'NONE',  ( 5.558508435838322548, -2.857531096718671115, 24.49999999999999289 ) ) ;
#1659=ORIENTED_EDGE ( 'NONE', *, *, #3570, .F. ) ;
#1662=ORIENTED_EDGE ( 'NONE', *, *, #10649, .T. ) ;
#1663=CARTESIAN_POINT ( 'NONE',  ( -5.317509234263939177, 2.779225709351033302, 11.49999999999998224 ) ) ;
#1664=EDGE_LOOP ( 'NONE', ( #12566, #10687, #3663, #8050 ) ) ;
#1666=DIRECTION ( 'NONE',  ( 0.5877852522924802425, -0.8090169943749422332, 0.000000000000000000 ) ) ;
#1667=EDGE_LOOP ( 'NONE', ( #3249, #5046 ) ) ;
#1669=CARTESIAN_POINT ( 'NONE',  ( 0.9739805876848001143, 5.920636045238165224, 5.261713868144209272 ) ) ;
#1670=EDGE_CURVE ( 'NONE', #9215, #1760, #9453, .T. ) ;
#1673=CARTESIAN_POINT ( 'NONE',  ( -5.859221468178966497, -2.178708437343180204, 5.974085423341712442 ) ) ;
#1674=CARTESIAN_POINT ( 'NONE',  ( -2.692215568229781031, -5.362327947133626260, 11.23770962164069687 ) ) ;
#1675=CARTESIAN_POINT ( 'NONE',  ( -5.648559266344434171, -2.676764518776131307, 25.11396179408071205 ) ) ;
#1677=CARTESIAN_POINT ( 'NONE',  ( -0.5039005892421096755, 6.230833003620542598, 30.12636388911297658 ) ) ;
#1678=VERTEX_POINT ( 'NONE', #14213 ) ;
#1682=CARTESIAN_POINT ( 'NONE',  ( 0.000000000000000000, 6.250000000000000888, 12.49999999999998401 ) ) ;
#1683=CARTESIAN_POINT ( 'NONE',  ( 7.180990026460741582, -3.384707322287397790, 5.000000000000004441 ) ) ;
#1685=CARTESIAN_POINT ( 'NONE',  ( 0.2637975869347833902, 6.245592211692893692, 5.973328399491914631 ) ) ;
#1686=CARTESIAN_POINT ( 'NONE',  ( 0.2622916576876764272, -5.995491482261826377, 31.97384942646813855 ) ) ;
#1687=CARTESIAN_POINT ( 'NONE',  ( -5.486741141153813395, 2.429871531109682792, 5.798882422479413101 ) ) ;
#1688=CARTESIAN_POINT ( 'NONE',  ( 0.9740012993921304263, 6.173846968979621153, 18.26164920628446708 ) ) ;
#1690=FACE_OUTER_BOUND ( 'NONE', #9959, .T. ) ;
#1691=AXIS2_PLACEMENT_3D ( 'NONE', #6918, #13984, #7870 ) ;
#1692=CARTESIAN_POINT ( 'NONE',  ( -4.435347140101169927, 4.403429997944371621, 18.13063932754211294 ) ) ;
#1697=ADVANCED_FACE ( 'NONE', ( #5876 ), #14538, .F. ) ;
#1700=ORIENTED_EDGE ( 'NONE', *, *, #6004, .T. ) ;
#1703=CARTESIAN_POINT ( 'NONE',  ( 0.8738043859791279067, -6.188821459035870554, 12.00341560223749759 ) ) ;
#1704=CARTESIAN_POINT ( 'NONE',  ( 5.558508435838199979, 2.857531096718914476, 30.86762589283693359 ) ) ;
#1705=FACE_OUTER_BOUND ( 'NONE', #4012, .T. ) ;
#1706=CARTESIAN_POINT ( 'NONE',  ( -4.154121946520862529, -4.670585111242981036, 31.79887838423339019 ) ) ;
#1708=CARTESIAN_POINT ( 'NONE',  ( -4.286401442266545736, -4.198423832313181059, 31.13061695532138984 ) ) ;
#1710=CARTESIAN_POINT ( 'NONE',  ( 5.783198643800754546, 1.602922020054761365, 5.973778239432934178 ) ) ;
#1716=CARTESIAN_POINT ( 'NONE',  ( 2.930922878467443038, 5.520395124723591174, 12.00389213124966759 ) ) ;
#1720=CARTESIAN_POINT ( 'NONE',  ( -4.143041610105435701, 4.340967609746908096, 18.61397738943082203 ) ) ;
#1723=ORIENTED_EDGE ( 'NONE', *, *, #12237, .T. ) ;
#1724=CARTESIAN_POINT ( 'NONE',  ( -4.196038884587234286, -4.289036423669209341, 17.49610204984018580 ) ) ;
#1730=CYLINDRICAL_SURFACE ( 'NONE', #6064, 1.000000000000000666 ) ;
#1731=CARTESIAN_POINT ( 'NONE',  ( -1.000049560716534502, 5.916071405810148676, 30.86967799011533486 ) ) ;
#1734=CARTESIAN_POINT ( 'NONE',  ( 5.725930890718318622, -2.506952462184073749, 5.799331489075775004 ) ) ;
#1735=LINE ( 'NONE', #11443, #8822 ) ;
#1737=CARTESIAN_POINT ( 'NONE',  ( -5.486741141153752999, -2.429871531109820904, 10.70111757752057358 ) ) ;
#1741=CARTESIAN_POINT ( 'NONE',  ( 7.490007020835728113, -2.433650805992114918, 17.99999999999998934 ) ) ;
#1742=ORIENTED_EDGE ( 'NONE', *, *, #9903, .T. ) ;
#1744=CYLINDRICAL_SURFACE ( 'NONE', #10390, 1.000000000000000666 ) ;
#1748=CARTESIAN_POINT ( 'NONE',  ( -5.935543223013847403, -0.8771126767607489993, 5.000000000000004441 ) ) ;
#1749=CARTESIAN_POINT ( 'NONE',  ( 2.031800923730693940E-13, -6.250000000000000888, 23.49999999999999289 ) ) ;
#1753=CARTESIAN_POINT ( 'NONE',  ( -3.923477796648659144, 4.541042560386356897, 17.12696220972948069 ) ) ;
#1755=CARTESIAN_POINT ( 'NONE',  ( 7.490007020835692586, -2.433650805992223720, 31.00000000000000000 ) ) ;
#1757=CARTESIAN_POINT ( 'NONE',  ( -1.000049271338467216, 6.169473353325554577, 30.86969612704551835 ) ) ;
#1759=EDGE_CURVE ( 'NONE', #5575, #5516, #1039, .T. ) ;
#1760=VERTEX_POINT ( 'NONE', #3321 ) ;
#1761=ORIENTED_EDGE ( 'NONE', *, *, #8988, .T. ) ;
#1762=CARTESIAN_POINT ( 'NONE',  ( 4.435347140101026042, -4.403429997944519059, 11.63234125634166105 ) ) ;
#1763=DIRECTION ( 'NONE',  ( 0.000000000000000000, 1.000000000000000000, 0.000000000000000000 ) ) ;
#1764=ORIENTED_EDGE ( 'NONE', *, *, #3943, .F. ) ;
#1765=CARTESIAN_POINT ( 'NONE',  ( 5.329945432499675562, -2.755769831645047852, 18.26229037835932090 ) ) ;
#1767=CARTESIAN_POINT ( 'NONE',  ( -0.8736772044958448502, 6.188841968496081591, 17.49611573292807520 ) ) ;
#1769=CARTESIAN_POINT ( 'NONE',  ( 0.5042675786779511338, 6.230788509548835563, 18.87331068310452054 ) ) ;
#1773=DIRECTION ( 'NONE',  ( 0.5877852522924802425, -0.8090169943749422332, 0.000000000000000000 ) ) ;
#1775=CARTESIAN_POINT ( 'NONE',  ( -5.317509234263930296, -2.779225709351048401, 5.000000000000004441 ) ) ;
#1779=CARTESIAN_POINT ( 'NONE',  ( 4.005998022990028495, -4.467726698309201439, 4.200681937418260681 ) ) ;
#1780=ORIENTED_EDGE ( 'NONE', *, *, #6602, .F. ) ;
#1781=CARTESIAN_POINT ( 'NONE',  ( -2.817313151351311884, 5.579000502529369854, 17.86765874365829276 ) ) ;
#1783=CARTESIAN_POINT ( 'NONE',  ( -4.196288036172577840, 4.288789315524710766, 23.99687951097622829 ) ) ;
#1784=CARTESIAN_POINT ( 'NONE',  ( -0.8002302970946589822, 5.947135855825866457, 4.386017732123007384 ) ) ;
#1786=B_SPLINE_CURVE_WITH_KNOTS ( 'NONE', 3,
 ( #13951, #14106, #5690, #15157, #8073, #11411, #10228, #3061, #7992, #10536, #15394, #9192, #12833, #12754, #9343, #13871, #14031, #590 ),
 .UNSPECIFIED., .F., .F.,
 ( 4, 2, 2, 2, 2, 2, 2, 2, 4 ),
 ( 0.003131486019301987691, 0.003522824630466695264, 0.003914163241631402404, 0.004305501852796110411, 0.004696840463960817551, 0.005088179075125525558, 0.005479517686290230963, 0.005870856297454938102, 0.006262194908619644375 ),
 .UNSPECIFIED. ) ;
#1787=CARTESIAN_POINT ( 'NONE',  ( 4.344313232727111007, 4.493553492990106868, 5.504369696801527212 ) ) ;
#1790=CARTESIAN_POINT ( 'NONE',  ( -2.931156713028406635, -5.520271803279254819, 30.49563030319847101 ) ) ;
#1794=FACE_BOUND ( 'NONE', #1352, .T. ) ;
#1795=CARTESIAN_POINT ( 'NONE',  ( -5.620879908643947154, 2.102487719021948642, 18.97377823943293151 ) ) ;
#1798=CARTESIAN_POINT ( 'NONE',  ( 2.841163418881286429, -5.567120626447985998, 24.76236973443873879 ) ) ;
#1800=ORIENTED_EDGE ( 'NONE', *, *, #2729, .T. ) ;
#1801=CARTESIAN_POINT ( 'NONE',  ( -3.311384659207173620, -5.004923837169396705, 17.02641404563305372 ) ) ;
#1803=CARTESIAN_POINT ( 'NONE',  ( -0.9740012993920151851, -6.173846968979639804, 5.261649206284398694 ) ) ;
#1805=CARTESIAN_POINT ( 'NONE',  ( -5.783239563508439041, 1.602707436861068313, 4.026414045633067929 ) ) ;
#1808=B_SPLINE_CURVE_WITH_KNOTS ( 'NONE', 3,
 ( #5054, #9908, #14762, #7514, #1456, #6334, #11171, #5134, #11403, #15071, #350, #4086, #14022, #15222, #5215, #1541, #1692, #13789 ),
 .UNSPECIFIED., .F., .F.,
 ( 4, 2, 2, 2, 2, 2, 2, 2, 4 ),
 ( 0.000000000000000000, 0.0003914357524127486240, 0.0007828715048254972480, 0.001174307257238245980, 0.001565743009650994496, 0.001957178762063743228, 0.002348614514476492394, 0.002740050266889241994, 0.003131486019301991160 ),
 .UNSPECIFIED. ) ;
#1810=CARTESIAN_POINT ( 'NONE',  ( -0.8002302970946246763, 5.947135855825869122, 30.38601773212298340 ) ) ;
#1812=CARTESIAN_POINT ( 'NONE',  ( -4.267838854167165685, 4.217593933790345417, 30.73760108194402463 ) ) ;
#1815=ORIENTED_EDGE ( 'NONE', *, *, #4228, .T. ) ;
#1817=ORIENTED_EDGE ( 'NONE', *, *, #9119, .F. ) ;
#1818=CARTESIAN_POINT ( 'NONE',  ( -5.931734679891428108, 0.9039278060245400370, 24.76382603205594179 ) ) ;
#1820=VERTEX_POINT ( 'NONE', #14701 ) ;
#1821=CYLINDRICAL_SURFACE ( 'NONE', #14190, 0.9999999999999998890 ) ;
#1827=CARTESIAN_POINT ( 'NONE',  ( -3.459447313391775136, -5.206669755181035697, 5.974000980233304503 ) ) ;
#1829=CARTESIAN_POINT ( 'NONE',  ( 2.668367453516707233, -5.373994336898093138, 5.000000000000004441 ) ) ;
#1830=CARTESIAN_POINT ( 'NONE',  ( -3.312341048453546932, 5.004306261885401952, 17.02601979877759319 ) ) ;
#1837=B_SPLINE_CURVE_WITH_KNOTS ( 'NONE', 3,
 ( #10194, #15200, #11529, #5579, #1007, #15045, #1899, #11608, #12648, #10270, #13176, #9088, #5501, #9528, #1979, #628, #15277, #14364 ),
 .UNSPECIFIED., .F., .F.,
 ( 4, 2, 2, 2, 2, 2, 2, 2, 4 ),
 ( 0.003131918686235979094, 0.003523310662250268930, 0.003914702638264559199, 0.004306094614278849035, 0.004697486590293138871, 0.005088878566307429574, 0.005480270542321719410, 0.005871662518336009245, 0.006263054494350299081 ),
 .UNSPECIFIED. ) ;
#1838=CARTESIAN_POINT ( 'NONE',  ( 2.817313151351127587, -5.579000502529462224, 11.49999999999998224 ) ) ;
#1843=CARTESIAN_POINT ( 'NONE',  ( -5.317509234263865459, -2.779225709351170526, 17.99999999999998934 ) ) ;
#1849=CARTESIAN_POINT ( 'NONE',  ( 5.487097279078465561, 2.429065649168737462, 18.79952054102714598 ) ) ;
#1854=CARTESIAN_POINT ( 'NONE',  ( 5.131373506000599605, 7.062729720844090231, 5.000000000000004441 ) ) ;
#1855=B_SPLINE_CURVE_WITH_KNOTS ( 'NONE', 3,
 ( #6718, #15218, #4318, #4473, #9565, #15377, #13133, #12974, #10676, #4714, #8058, #13219, #809, #14170, #9327, #9255, #3275, #8138 ),
 .UNSPECIFIED., .F., .F.,
 ( 4, 2, 2, 2, 2, 2, 2, 2, 4 ),
 ( 0.000000000000000000, 0.0003914898357794973868, 0.0007829796715589947735, 0.001174469507338492215, 0.001565959343117989547, 0.001957449178897487096, 0.002348939014676984429, 0.002740428850456481762, 0.003131918686235979094 ),
 .UNSPECIFIED. ) ;
#1860=CARTESIAN_POINT ( 'NONE',  ( -0.5039005892420553856, 6.230833003620545263, 10.62636388911295882 ) ) ;
#1863=DIRECTION ( 'NONE',  ( -0.3090169943749447867, -0.9510565162951544194, 0.000000000000000000 ) ) ;
#1867=CARTESIAN_POINT ( 'NONE',  ( 4.286401442266532413, 4.198423832313196158, 4.867639214160894845 ) ) ;
#1872=CARTESIAN_POINT ( 'NONE',  ( 0.000000000000000000, 0.000000000000000000, 53.67766952966368876 ) ) ;
#1873=CARTESIAN_POINT ( 'NONE',  ( 0.6144300524836082689, 6.220417338033028543, 23.70033372175935682 ) ) ;
#1876=CARTESIAN_POINT ( 'NONE',  ( -4.070051655338261298, 4.744673454622341247, 25.37367328635991370 ) ) ;
#1877=CARTESIAN_POINT ( 'NONE',  ( -0.9999196734180613166, -5.916093360767550102, 24.36725955955066780 ) ) ;
#1880=CARTESIAN_POINT ( 'NONE',  ( 5.531757352715644060, -2.326874507723228458, 17.12619317285288645 ) ) ;
#1889=CARTESIAN_POINT ( 'NONE',  ( 7.180990026460747799, -3.384707322287378695, 31.00000000000000000 ) ) ;
#1896=AXIS2_PLACEMENT_3D ( 'NONE', #10725, #15583, #14373 ) ;
#1899=CARTESIAN_POINT ( 'NONE',  ( -5.531209434046322926, -2.328189801702654549, 30.12696220972948424 ) ) ;
#1901=CARTESIAN_POINT ( 'NONE',  ( 5.620786884546309814, 2.102685372472837599, 17.02641404563306082 ) ) ;
#1903=CARTESIAN_POINT ( 'NONE',  ( 5.903230462362999198, -1.077253041748644558, 23.88557478428062097 ) ) ;
#1909=FACE_OUTER_BOUND ( 'NONE', #122, .T. ) ;
#1910=CARTESIAN_POINT ( 'NONE',  ( -5.620879908643915179, -2.102487719022031243, 17.02622176056705783 ) ) ;
#1911=CARTESIAN_POINT ( 'NONE',  ( -0.9999196734181325930, -5.916093360767538556, 17.86725955955069978 ) ) ;
#1913=ORIENTED_EDGE ( 'NONE', *, *, #792, .F. ) ;
#1914=ORIENTED_EDGE ( 'NONE', *, *, #2090, .T. ) ;
#1916=CARTESIAN_POINT ( 'NONE',  ( -6.155854678529464330, -1.081900940642162690, 10.99574050496990196 ) ) ;
#1918=ADVANCED_FACE ( 'NONE', ( #292, #10009, #1323, #4025, #14855, #8817, #13646, #8901, #4999, #2762, #12460, #11270, #2844, #7690, #370, #5237, #10083, #14933, #14624, #6724, #4923, #3713, #8589, #13424, #2527, #7383 ), #12224, .T. ) ;
#1919=ORIENTED_EDGE ( 'NONE', *, *, #13965, .F. ) ;
#1920=CARTESIAN_POINT ( 'NONE',  ( 5.782895619916205376, -1.604017620857909998, 18.97408052783099563 ) ) ;
#1922=CARTESIAN_POINT ( 'NONE',  ( -0.5043776560896956473, 6.230795654995843869, 18.87337476296005079 ) ) ;
#1923=CARTESIAN_POINT ( 'NONE',  ( 3.159612573729055907, 5.393342049074733247, 25.30026515017675948 ) ) ;
#1926=DIRECTION ( 'NONE',  ( 0.9510565162951499785, 0.3090169943749582204, 0.000000000000000000 ) ) ;
#1932=ORIENTED_EDGE ( 'NONE', *, *, #7820, .F. ) ;
#1934=EDGE_CURVE ( 'NONE', #8231, #10984, #6388, .T. ) ;
#1935=ORIENTED_EDGE ( 'NONE', *, *, #4528, .T. ) ;
#1936=CARTESIAN_POINT ( 'NONE',  ( -4.344762547369822592, 4.493114738039108325, 17.49691356133953590 ) ) ;
#1938=CARTESIAN_POINT ( 'NONE',  ( -0.6152055445546463774, 5.969096820685154015, 5.799049686702669071 ) ) ;
#1940=B_SPLINE_CURVE_WITH_KNOTS ( 'NONE', 3,
 ( #3323, #15424, #9455, #9536, #8025, #11908, #14290, #2123, #9226, #10802, #11754, #8187, #2284, #11990, #8109, #14059, #13024, #7072 ),
 .UNSPECIFIED., .F., .F.,
 ( 4, 2, 2, 2, 2, 2, 2, 2, 4 ),
 ( 0.000000000000000000, 0.0003914357524127449377, 0.0007828715048254898754, 0.001174307257238234922, 0.001565743009650979751, 0.001957178762063724580, 0.002348614514476469843, 0.002740050266889214672, 0.003131486019301959502 ),
 .UNSPECIFIED. ) ;
#1946=CARTESIAN_POINT ( 'NONE',  ( 7.799024015210631156, -1.482594289697088730, 5.000000000000004441 ) ) ;
#1955=CARTESIAN_POINT ( 'NONE',  ( 3.458623254138621483, -5.207221900902879952, 25.47377282875268278 ) ) ;
#1956=CARTESIAN_POINT ( 'NONE',  ( 0.000000000000000000, 0.000000000000000000, 0.000000000000000000 ) ) ;
#1958=LINE ( 'NONE', #9216, #11943 ) ;
#1961=CARTESIAN_POINT ( 'NONE',  ( -5.375763363753385704, 2.665284979407666732, 23.99610204984015382 ) ) ;
#1967=FACE_BOUND ( 'NONE', #9173, .T. ) ;
#1975=CARTESIAN_POINT ( 'NONE',  ( 5.375886393124376994, -2.665038680141303740, 5.504397606442131163 ) ) ;
#1977=ORIENTED_EDGE ( 'NONE', *, *, #6193, .F. ) ;
#1978=CYLINDRICAL_SURFACE ( 'NONE', #8634, 1.000000000000000444 ) ;
#1979=CARTESIAN_POINT ( 'NONE',  ( -5.915641100987819812, -1.003868594704814932, 30.49571079637979665 ) ) ;
#1980=CARTESIAN_POINT ( 'NONE',  ( -3.922672396097092840, 4.541739265057668007, 31.87364704684421923 ) ) ;
#1984=CARTESIAN_POINT ( 'NONE',  ( -0.9740856415298599913, 6.173834621338629702, 24.23852653055524442 ) ) ;
#1988=CARTESIAN_POINT ( 'NONE',  ( -5.570722351696168140, -2.834100162822159596, 24.76190213084012370 ) ) ;
#1989=CARTESIAN_POINT ( 'NONE',  ( -5.866923913994614104, -1.260079467906668027, 17.20047945897285047 ) ) ;
#1993=ORIENTED_EDGE ( 'NONE', *, *, #6351, .T. ) ;
#1994=CARTESIAN_POINT ( 'NONE',  ( 2.930600586412925868, -5.520563544161773528, 18.50308643866044633 ) ) ;
#2000=CARTESIAN_POINT ( 'NONE',  ( -0.1306497350715297157, 6.000000000000007105, 23.50000000000000000 ) ) ;
#2008=CARTESIAN_POINT ( 'NONE',  ( -5.746996058422766396, -1.729015645941953672, 3.999920388255239434 ) ) ;
#2012=VERTEX_POINT ( 'NONE', #2212 ) ;
#2013=CARTESIAN_POINT ( 'NONE',  ( 4.142173849413810949, -4.341773579105344893, 4.384806175511481996 ) ) ;
#2014=ORIENTED_EDGE ( 'NONE', *, *, #3349, .T. ) ;
#2015=CARTESIAN_POINT ( 'NONE',  ( -4.290821322214496192, 4.545321419741441105, 17.38558052754515160 ) ) ;
#2016=DIRECTION ( 'NONE',  ( 0.5877852522924802425, -0.8090169943749422332, 0.000000000000000000 ) ) ;
#2018=ORIENTED_EDGE ( 'NONE', *, *, #1640, .F. ) ;
#2019=CARTESIAN_POINT ( 'NONE',  ( 4.416397290909871209, 4.422724436066468812, 11.23620383159194702 ) ) ;
#2020=LINE ( 'NONE', #10465, #6923 ) ;
#2028=CARTESIAN_POINT ( 'NONE',  ( 6.021135683317733189, -1.680226122398085220, 17.02622717124729945 ) ) ;
#2030=CARTESIAN_POINT ( 'NONE',  ( 1.353717517954364224E-13, -6.250000000000000888, 18.99999999999998934 ) ) ;
#2034=DIRECTION ( 'NONE',  ( 0.000000000000000000, 0.000000000000000000, 1.000000000000000000 ) ) ;
#2035=VERTEX_POINT ( 'NONE', #11918 ) ;
#2039=CARTESIAN_POINT ( 'NONE',  ( -5.746837578675966896, 1.729433780394384446, 23.50004946353776702 ) ) ;
#2042=ADVANCED_FACE ( 'NONE', ( #4696, #8441 ), #7322, .F. ) ;
#2043=CARTESIAN_POINT ( 'NONE',  ( 5.985119669071150561, 1.805077827356446507, 25.49991741810288559 ) ) ;
#2047=CARTESIAN_POINT ( 'NONE',  ( -2.668367453516725885, 5.373994336898083368, 31.00000000000000000 ) ) ;
#2048=CARTESIAN_POINT ( 'NONE',  ( -5.558508435838230177, 2.857531096718855412, 4.869360672457871075 ) ) ;
#2049=CARTESIAN_POINT ( 'NONE',  ( 5.131373506000437068, 7.062729720844210135, 24.49999999999999289 ) ) ;
#2052=B_SPLINE_CURVE_WITH_KNOTS ( 'NONE', 3,
 ( #1452, #2503, #4977, #13393, #9754, #6174, #3917, #7433, #10935, #6330, #8795, #268, #8488, #1222, #9982, #2418, #13623, #5130 ),
 .UNSPECIFIED., .F., .F.,
 ( 4, 2, 2, 2, 2, 2, 2, 2, 4 ),
 ( 0.000000000000000000, 0.0003914357524127467266, 0.0007828715048254934533, 0.001174307257238240126, 0.001565743009650986907, 0.001957178762063733687, 0.002348614514476480251, 0.002740050266889227249, 0.003131486019301973813 ),
 .UNSPECIFIED. ) ;
#2053=CARTESIAN_POINT ( 'NONE',  ( 6.768587589771821120E-14, 6.000000000000000888, 12.49999999999998401 ) ) ;
#2055=CARTESIAN_POINT ( 'NONE',  ( -4.267992336621131422, -4.217442018460069164, 4.738056759968542586 ) ) ;
#2059=CARTESIAN_POINT ( 'NONE',  ( -3.883588957979163592, -4.898466244119004998, 5.973772828752684561 ) ) ;
#2061=CARTESIAN_POINT ( 'NONE',  ( 2.782468714962387235, -5.316055268221427710, 10.99610204984017336 ) ) ;
#2066=CARTESIAN_POINT ( 'NONE',  ( 3.779681992289790404, 4.979315417303903146, 31.99995078984292007 ) ) ;
#2069=ORIENTED_EDGE ( 'NONE', *, *, #4392, .T. ) ;
#2070=ORIENTED_EDGE ( 'NONE', *, *, #652, .F. ) ;
#2073=CARTESIAN_POINT ( 'NONE',  ( -2.668367453516768517, 5.373994336898063828, 11.63239388001634822 ) ) ;
#2074=ORIENTED_EDGE ( 'NONE', *, *, #10232, .F. ) ;
#2077=CARTESIAN_POINT ( 'NONE',  ( 0.2622916576876685446, -5.995491482261829042, 5.973849426468138546 ) ) ;
#2078=CARTESIAN_POINT ( 'NONE',  ( -3.779082820360602835, -4.979770177899319528, 3.999950931234675711 ) ) ;
#2081=CARTESIAN_POINT ( 'NONE',  ( -2.668367453516708565, 5.373994336898094026, 5.000000000000004441 ) ) ;
#2084=CARTESIAN_POINT ( 'NONE',  ( -5.375605342016492649, -2.665598297262314897, 4.496879510976233618 ) ) ;
#2087=VERTEX_POINT ( 'NONE', #10735 ) ;
#2089=VERTEX_POINT ( 'NONE', #12160 ) ;
#2090=EDGE_CURVE ( 'NONE', #12192, #1426, #8671, .T. ) ;
#2091=CARTESIAN_POINT ( 'NONE',  ( -0.8736772044959224548, 6.188841968496069157, 10.99611573292808764 ) ) ;
#2094=AXIS2_PLACEMENT_3D ( 'NONE', #4822, #8719, #14516 ) ;
#2096=CARTESIAN_POINT ( 'NONE',  ( -5.666074146197985328, 1.978051345703193187, 16.99995067926685977 ) ) ;
#2098=EDGE_CURVE ( 'NONE', #14280, #471, #13746, .T. ) ;
#2099=CARTESIAN_POINT ( 'NONE',  ( -4.286401442266628337, -4.198423832313095794, 17.99999999999998934 ) ) ;
#2100=CARTESIAN_POINT ( 'NONE',  ( -4.070051655338168040, 4.744673454622424735, 12.37367328635990660 ) ) ;
#2102=CARTESIAN_POINT ( 'NONE',  ( -3.567258970016065955, -5.133675764669609620, 25.50008219321555458 ) ) ;
#2103=CARTESIAN_POINT ( 'NONE',  ( 2.817313151351187983, -5.579000502529432026, 5.000000000000004441 ) ) ;
#2107=CARTESIAN_POINT ( 'NONE',  ( -6.105925084677658710, -1.337450587213287356, 18.79933148907576523 ) ) ;
#2108=DIRECTION ( 'NONE',  ( 0.000000000000000000, 1.000000000000000000, 0.000000000000000000 ) ) ;
#2109=ADVANCED_FACE ( 'NONE', ( #11358 ), #1648, .F. ) ;
#2112=CARTESIAN_POINT ( 'NONE',  ( -4.435347140101218777, 4.403429997944323659, 24.49999999999999289 ) ) ;
#2113=CARTESIAN_POINT ( 'NONE',  ( 5.131373506000437068, 7.062729720844210135, 24.49999999999999289 ) ) ;
#2115=CARTESIAN_POINT ( 'NONE',  ( -6.142844459177225325, 1.156093792145259203, 18.61560192892921251 ) ) ;
#2118=LINE ( 'NONE', #9924, #11741 ) ;
#2119=CARTESIAN_POINT ( 'NONE',  ( 6.143020266951002561, 1.155160780047578495, 25.11441947245484485 ) ) ;
#2121=DIRECTION ( 'NONE',  ( -0.5877852522924685852, -0.8090169943749507819, 0.000000000000000000 ) ) ;
#2123=CARTESIAN_POINT ( 'NONE',  ( 5.858736126997138527, 2.179962889277050841, 10.52640428276697726 ) ) ;
#2124=CARTESIAN_POINT ( 'NONE',  ( -5.859221468178994918, 2.178708437343097160, 4.025914576658297328 ) ) ;
#2126=ORIENTED_EDGE ( 'NONE', *, *, #14143, .T. ) ;
#2128=CARTESIAN_POINT ( 'NONE',  ( 2.848727059636023018, 5.281416301279862502, 30.38557478428061742 ) ) ;
#2129=ORIENTED_EDGE ( 'NONE', *, *, #7561, .T. ) ;
#2130=ADVANCED_FACE ( 'NONE', ( #458 ), #12315, .F. ) ;
#2131=CYLINDRICAL_SURFACE ( 'NONE', #13944, 1.000000000000000666 ) ;
#2132=CARTESIAN_POINT ( 'NONE',  ( -4.196038884587202311, 4.289036423669238651, 31.50389795015983552 ) ) ;
#2133=CARTESIAN_POINT ( 'NONE',  ( 2.817313151350985923, 5.579000502529535055, 17.86939309276500154 ) ) ;
#2140=CARTESIAN_POINT ( 'NONE',  ( -5.317509234263866347, -2.779225709351170526, 17.86938304467859595 ) ) ;
#2141=CARTESIAN_POINT ( 'NONE',  ( -0.1306171417087258479, -6.000000000000002665, 16.99999999999998224 ) ) ;
#2145=ORIENTED_EDGE ( 'NONE', *, *, #494, .T. ) ;
#2147=DIRECTION ( 'NONE',  ( 0.000000000000000000, 0.000000000000000000, 1.000000000000000000 ) ) ;
#2148=ORIENTED_EDGE ( 'NONE', *, *, #9837, .F. ) ;
#2151=CARTESIAN_POINT ( 'NONE',  ( -0.2622916576874523287, 5.995491482261837035, 25.47384942646813499 ) ) ;
#2153=CARTESIAN_POINT ( 'NONE',  ( -4.416837305303439543, -4.422286678979068242, 4.738097869159890507 ) ) ;
#2156=CARTESIAN_POINT ( 'NONE',  ( -4.322356511625772058, 7.650514973136511188, 5.000000000000004441 ) ) ;
#2159=CARTESIAN_POINT ( 'NONE',  ( 2.840966774240303305, -5.567223638426833432, 4.738097869159889619 ) ) ;
#2162=ORIENTED_EDGE ( 'NONE', *, *, #6351, .F. ) ;
#2167=CARTESIAN_POINT ( 'NONE',  ( -5.558508435838136919, 2.857531096719036601, 24.63060690723497359 ) ) ;
#2168=EDGE_CURVE ( 'NONE', #1512, #7314, #4089, .T. ) ;
#2169=CARTESIAN_POINT ( 'NONE',  ( -2.841041022017486650, -5.567186575787210323, 24.23774718278286500 ) ) ;
#2171=ORIENTED_EDGE ( 'NONE', *, *, #6889, .T. ) ;
#2173=CARTESIAN_POINT ( 'NONE',  ( -0.1323408341374885389, -6.250000000000001776, 6.000000000000007105 ) ) ;
#2174=FACE_BOUND ( 'NONE', #7752, .T. ) ;
#2175=CARTESIAN_POINT ( 'NONE',  ( -3.567258970016013997, -5.133675764669648700, 19.00008219321555103 ) ) ;
#2176=CARTESIAN_POINT ( 'NONE',  ( 0.7993282387952456158, -5.947240459526492273, 18.61484358216956636 ) ) ;
#2177=FACE_OUTER_BOUND ( 'NONE', #6106, .T. ) ;
#2182=CARTESIAN_POINT ( 'NONE',  ( -6.081464507797595509, -1.446657058464349666, 18.87380055247394850 ) ) ;
#2185=CARTESIAN_POINT ( 'NONE',  ( -2.782769401326203429, 5.315896561274835896, 4.495710796379801977 ) ) ;
#2187=CARTESIAN_POINT ( 'NONE',  ( -0.6144377077729259451, -5.969178481556073557, 10.70033966857734775 ) ) ;
#2188=CARTESIAN_POINT ( 'NONE',  ( -0.5031281619705731956, -5.980084330432684503, 23.62602272744524967 ) ) ;
#2190=CYLINDRICAL_SURFACE ( 'NONE', #988, 1.000000000000000888 ) ;
#2191=DIRECTION ( 'NONE',  ( -0.9510565162951544194, 0.3090169943749447312, 0.000000000000000000 ) ) ;
#2193=CARTESIAN_POINT ( 'NONE',  ( -5.621278735166179708, 2.101423246382604582, 23.52591947216898305 ) ) ;
#2197=CARTESIAN_POINT ( 'NONE',  ( 6.176542424588136626, 0.9554180641284277797, 24.49999999999999289 ) ) ;
#2203=FACE_BOUND ( 'NONE', #15210, .T. ) ;
#2205=CARTESIAN_POINT ( 'NONE',  ( -4.143041610105294481, -4.340967609747044875, 30.38602261056917442 ) ) ;
#2206=EDGE_CURVE ( 'NONE', #15154, #14884, #5871, .T. ) ;
#2209=FACE_OUTER_BOUND ( 'NONE', #12234, .T. ) ;
#2210=ORIENTED_EDGE ( 'NONE', *, *, #14325, .T. ) ;
#2212=CARTESIAN_POINT ( 'NONE',  ( 5.558508435838189321, 2.857531096718932240, 5.000000000000004441 ) ) ;
#2213=DIRECTION ( 'NONE',  ( -0.5877852522924685852, -0.8090169943749507819, 0.000000000000000000 ) ) ;
#2216=CARTESIAN_POINT ( 'NONE',  ( 4.005998022990015173, -4.467726698309212097, 30.20068193741824913 ) ) ;
#2218=CARTESIAN_POINT ( 'NONE',  ( 3.736691294293456700, -4.695920479336350262, 10.52641404563304839 ) ) ;
#2222=CARTESIAN_POINT ( 'NONE',  ( 5.782895619916144980, 1.604017620858124271, 4.025919472168997260 ) ) ;
#2223=CARTESIAN_POINT ( 'NONE',  ( -0.6156307853268060404, -5.969051238897268519, 18.79870573410680379 ) ) ;
#2224=ORIENTED_EDGE ( 'NONE', *, *, #5208, .F. ) ;
#2225=B_SPLINE_CURVE_WITH_KNOTS ( 'NONE', 3,
 ( #8320, #7208, #9589, #3614, #13159, #11966, #10780, #4740, #8569, #12048, #15638, #3537, #15722, #1147, #9677, #115, #8408, #14515 ),
 .UNSPECIFIED., .F., .F.,
 ( 4, 2, 2, 2, 2, 2, 2, 2, 4 ),
 ( 0.000000000000000000, 0.0003914898357794963026, 0.0007829796715589926051, 0.001174469507338488962, 0.001565959343117985210, 0.001957449178897481459, 0.002348939014676977924, 0.002740428850456473955, 0.003131918686235970421 ),
 .UNSPECIFIED. ) ;
#2228=CARTESIAN_POINT ( 'NONE',  ( 4.435347140100996732, 4.403429997944549257, 30.86765874365831408 ) ) ;
#2230=ORIENTED_EDGE ( 'NONE', *, *, #14566, .F. ) ;
#2233=CARTESIAN_POINT ( 'NONE',  ( -0.9999502950800045475, 5.916088184763918179, 24.63108149190010820 ) ) ;
#2241=CARTESIAN_POINT ( 'NONE',  ( 2.840966774240286430, -5.567223638426841426, 30.73809786915987274 ) ) ;
#2243=LINE ( 'NONE', #5997, #8257 ) ;
#2244=EDGE_LOOP ( 'NONE', ( #13848, #357 ) ) ;
#2245=AXIS2_PLACEMENT_3D ( 'NONE', #11936, #1042, #3422 ) ;
#2246=ORIENTED_EDGE ( 'NONE', *, *, #10297, .T. ) ;
#2248=VERTEX_POINT ( 'NONE', #2334 ) ;
#2249=B_SPLINE_CURVE_WITH_KNOTS ( 'NONE', 3,
 ( #12899, #2313, #2151, #8217, #5599, #8381, #11631, #731, #2233, #9406, #14242, #13053, #7026, #11854, #15613, #5831, #2000, #4633 ),
 .UNSPECIFIED., .F., .F.,
 ( 4, 2, 2, 2, 2, 2, 2, 2, 4 ),
 ( 0.000000000000000000, 0.0003914904498596244128, 0.0007829808997192488256, 0.001174471349578873293, 0.001565961799438497651, 0.001957452249298122227, 0.002348942699157746585, 0.002740433149017370944, 0.003131923598876995302 ),
 .UNSPECIFIED. ) ;
#2250=ORIENTED_EDGE ( 'NONE', *, *, #4656, .T. ) ;
#2251=CARTESIAN_POINT ( 'NONE',  ( 0.8730628416137486969, 6.188929913094962210, 30.49504929893118899 ) ) ;
#2252=CARTESIAN_POINT ( 'NONE',  ( -2.931156713028560734, -5.520271803279174883, 23.99563030319847812 ) ) ;
#2256=CARTESIAN_POINT ( 'NONE',  ( 5.317509234264033324, -2.779225709350852114, 17.99999999999998934 ) ) ;
#2258=CARTESIAN_POINT ( 'NONE',  ( -4.435347140101121965, 4.403429997944421359, 11.49999999999998224 ) ) ;
#2259=CARTESIAN_POINT ( 'NONE',  ( -6.081509788407695183, -1.446521464462901196, 23.62618035954929141 ) ) ;
#2260=CARTESIAN_POINT ( 'NONE',  ( -2.817313151351291012, -5.579000502529381400, 24.63234125634167526 ) ) ;
#2261=SURFACE_SIDE_STYLE ('',( #11731 ) ) ;
#2264=CARTESIAN_POINT ( 'NONE',  ( 3.011899281037421883, 5.190111395030274188, 31.80022217383877958 ) ) ;
#2267=DIRECTION ( 'NONE',  ( 0.5877852522924802425, -0.8090169943749422332, 0.000000000000000000 ) ) ;
#2269=CARTESIAN_POINT ( 'NONE',  ( 4.286401442266438266, 4.198423832313292081, 17.86763921416087797 ) ) ;
#2270=B_SPLINE_CURVE_WITH_KNOTS ( 'NONE', 3,
 ( #4615, #4536, #15516, #7084, #11691, #790, #13996, #1901, #9468, #13113, #11921, #3252, #3332, #5657, #945, #10503, #15359, #5581 ),
 .UNSPECIFIED., .F., .F.,
 ( 4, 2, 2, 2, 2, 2, 2, 2, 4 ),
 ( 0.000000000000000000, 0.0003914898357794948389, 0.0007829796715589896778, 0.001174469507338484625, 0.001565959343117979356, 0.001957449178897474086, 0.002348939014676969250, 0.002740428850456463981, 0.003131918686235958711 ),
 .UNSPECIFIED. ) ;
#2272=ORIENTED_EDGE ( 'NONE', *, *, #15433, .F. ) ;
#2275=ORIENTED_EDGE ( 'NONE', *, *, #7022, .T. ) ;
#2276=CARTESIAN_POINT ( 'NONE',  ( -4.006441409774651241, -4.467329318258288495, 5.798882422479411325 ) ) ;
#2280=CARTESIAN_POINT ( 'NONE',  ( -0.6156133477426608547, -6.220296490279944024, 31.79872387345512053 ) ) ;
#2282=CARTESIAN_POINT ( 'NONE',  ( -2.997451966578419835, 5.485105005466003547, 5.615177803758428787 ) ) ;
#2284=CARTESIAN_POINT ( 'NONE',  ( 6.105747081304174095, 1.338335777572260854, 10.69973484982323342 ) ) ;
#2287=CARTESIAN_POINT ( 'NONE',  ( 5.940390500375388072, 6.474944468551740329, 24.49999999999999289 ) ) ;
#2289=CARTESIAN_POINT ( 'NONE',  ( 5.915699123067185816, 1.003533581835384769, 23.99610204984015382 ) ) ;
#2290=EDGE_CURVE ( 'NONE', #6278, #6786, #11548, .T. ) ;
#2291=ORIENTED_EDGE ( 'NONE', *, *, #3366, .F. ) ;
#2293=CARTESIAN_POINT ( 'NONE',  ( -4.196038884587270701, -4.289036423669171150, 23.99610204984015738 ) ) ;
#2294=CARTESIAN_POINT ( 'NONE',  ( 0.2619041840696964552, -6.245686665308495478, 23.52605849433794916 ) ) ;
#2296=CARTESIAN_POINT ( 'NONE',  ( -5.131373506000769247, 7.062729720843990755, 11.49999999999998224 ) ) ;
#2298=CARTESIAN_POINT ( 'NONE',  ( 4.286401442266496886, -4.198423832313229020, 17.99999999999998934 ) ) ;
#2300=CARTESIAN_POINT ( 'NONE',  ( -5.769755079862298963, -2.405651898699021629, 4.126941084456994702 ) ) ;
#2301=CARTESIAN_POINT ( 'NONE',  ( 5.375886393124385876, -2.665038680141283756, 31.50439760644212939 ) ) ;
#2303=CARTESIAN_POINT ( 'NONE',  ( -6.142908455506947085, 1.155755562476039833, 10.88482219624155967 ) ) ;
#2306=VERTEX_POINT ( 'NONE', #12706 ) ;
#2307=EDGE_CURVE ( 'NONE', #10183, #7094, #8724, .T. ) ;
#2310=EDGE_LOOP ( 'NONE', ( #1236, #473 ) ) ;
#2311=PRODUCT ( 'strain limiting mesh layer', 'strain limiting mesh layer', '', ( #5135 ) ) ;
#2313=CARTESIAN_POINT ( 'NONE',  ( -0.1323933160973585210, 6.000000000000004441, 25.49999999999999289 ) ) ;
#2314=CARTESIAN_POINT ( 'NONE',  ( 6.176542424588110869, 0.9554180641286114106, 31.13060690723498425 ) ) ;
#2322=ORIENTED_EDGE ( 'NONE', *, *, #13868, .T. ) ;
#2323=AXIS2_PLACEMENT_3D ( 'NONE', #6472, #7570, #1435 ) ;
#2328=CARTESIAN_POINT ( 'NONE',  ( 0.9737725088282426222, 6.173885267451817427, 30.73735758726564882 ) ) ;
#2329=CARTESIAN_POINT ( 'NONE',  ( -3.567624405365383833, -5.133384272590680197, 23.50004921015705150 ) ) ;
#2330=CARTESIAN_POINT ( 'NONE',  ( 0.8736772044959983941, -6.188841968496061163, 4.496115732928122277 ) ) ;
#2331=ADVANCED_FACE ( 'NONE', ( #10328 ), #9674, .F. ) ;
#2332=CARTESIAN_POINT ( 'NONE',  ( -5.570722351696249852, -2.834100162821999280, 31.26190213084010239 ) ) ;
#2334=CARTESIAN_POINT ( 'NONE',  ( 2.031800923283433283E-13, -6.000000000000000888, 23.49999999999999289 ) ) ;
#2335=PRODUCT_DEFINITION ( 'UNKNOWN', '', #9596, #7853 ) ;
#2337=VECTOR ( 'NONE', #10079, 1000.000000000000000 ) ;
#2338=B_SPLINE_CURVE_WITH_KNOTS ( 'NONE', 3,
 ( #10075, #207, #8893, #11262, #2834, #11104, #5310, #11339, #7681, #362, #12530, #6266, #3934, #15084, #9049, #436, #5386, #2910 ),
 .UNSPECIFIED., .F., .F.,
 ( 4, 2, 2, 2, 2, 2, 2, 2, 4 ),
 ( 0.003131486019301959502, 0.003522824630466669243, 0.003914163241631378985, 0.004305501852796088727, 0.004696840463960799336, 0.005088179075125509945, 0.005479517686290219687, 0.005870856297454930296, 0.006262194908619640905 ),
 .UNSPECIFIED. ) ;
#2340=EDGE_CURVE ( 'NONE', #13429, #8130, #2827, .T. ) ;
#2341=CARTESIAN_POINT ( 'NONE',  ( -5.903061651806536858, -2.057626436184982754, 23.50008258189710020 ) ) ;
#2346=CARTESIAN_POINT ( 'NONE',  ( -6.176542424588083335, -0.9554180641287667308, 17.99999999999998934 ) ) ;
#2347=CARTESIAN_POINT ( 'NONE',  ( 5.317509234263941842, 2.779225709351030638, 31.00000000000000000 ) ) ;
#2350=CARTESIAN_POINT ( 'NONE',  ( 5.317509234263963158, 2.779225709350988449, 11.49999999999998224 ) ) ;
#2351=B_SPLINE_CURVE_WITH_KNOTS ( 'NONE', 3,
 ( #13311, #2167, #8483, #7040, #4571, #9667, #2412, #3605, #4733, #13236, #7279, #10691, #6964, #15551, #12115, #1217, #6087, #10929 ),
 .UNSPECIFIED., .F., .F.,
 ( 4, 2, 2, 2, 2, 2, 2, 2, 4 ),
 ( 0.003131486019301974680, 0.003522824630466682688, 0.003914163241631390261, 0.004305501852796098268, 0.004696840463960806275, 0.005088179075125514282, 0.005479517686290222289, 0.005870856297454930296, 0.006262194908619638303 ),
 .UNSPECIFIED. ) ;
#2353=CARTESIAN_POINT ( 'NONE',  ( 5.867109477881260027, 1.259218163100832566, 25.29888242247940866 ) ) ;
#2354=ORIENTED_EDGE ( 'NONE', *, *, #11370, .T. ) ;
#2357=ORIENTED_EDGE ( 'NONE', *, *, #8275, .T. ) ;
#2358=CARTESIAN_POINT ( 'NONE',  ( 2.841163418881210490, 5.567120626448023302, 24.23763026556123279 ) ) ;
#2361=CARTESIAN_POINT ( 'NONE',  ( -5.725684683139623310, 2.507514573674738845, 12.29887838423337953 ) ) ;
#2368=ORIENTED_EDGE ( 'NONE', *, *, #6341, .T. ) ;
#2372=ORIENTED_EDGE ( 'NONE', *, *, #6889, .F. ) ;
#2374=DIRECTION ( 'NONE',  ( 0.000000000000000000, 1.000000000000000000, 0.000000000000000000 ) ) ;
#2375=EDGE_CURVE ( 'NONE', #2588, #10768, #2052, .T. ) ;
#2376=CARTESIAN_POINT ( 'NONE',  ( 0.000000000000000000, 0.000000000000000000, 0.000000000000000000 ) ) ;
#2378=CARTESIAN_POINT ( 'NONE',  ( 0.7995524673975999974, 6.199337389817264565, 12.11453679452461429 ) ) ;
#2380=CARTESIAN_POINT ( 'NONE',  ( 4.267936573529138577, 4.217499624512312195, 18.26229037835932090 ) ) ;
#2382=CARTESIAN_POINT ( 'NONE',  ( -0.7995298244854430747, -5.947211616899250153, 31.61456014619858124 ) ) ;
#2384=CARTESIAN_POINT ( 'NONE',  ( -0.9999171162588356143, -6.169494774098570389, 17.86722320330672886 ) ) ;
#2385=CARTESIAN_POINT ( 'NONE',  ( -6.021167129161070442, 1.680051667990249520, 10.52640428276697548 ) ) ;
#2386=CARTESIAN_POINT ( 'NONE',  ( -5.866984344570854049, 1.259800266528525725, 30.20068193741825624 ) ) ;
#2388=ORIENTED_EDGE ( 'NONE', *, *, #15476, .F. ) ;
#2391=CYLINDRICAL_SURFACE ( 'NONE', #9882, 1.000000000000000888 ) ;
#2394=CARTESIAN_POINT ( 'NONE',  ( 7.347881242120658060E-16, 6.000000000000000888, 4.000000000000004441 ) ) ;
#2395=CARTESIAN_POINT ( 'NONE',  ( -5.317509234263900098, -2.779225709351108797, 11.49999999999998224 ) ) ;
#2399=CARTESIAN_POINT ( 'NONE',  ( -5.842988226680579267, 1.369004370660639180, 31.87380682714711355 ) ) ;
#2403=CARTESIAN_POINT ( 'NONE',  ( 3.883716939929148459, -4.898343590941119707, 4.026404282766995912 ) ) ;
#2405=LINE ( 'NONE', #7004, #15628 ) ;
#2412=CARTESIAN_POINT ( 'NONE',  ( -5.769755079862251890, 2.405651898699137092, 25.37305891554299819 ) ) ;
#2414=CARTESIAN_POINT ( 'NONE',  ( 4.005998022989933460, -4.467726698309286704, 17.20068193741824558 ) ) ;
#2416=EDGE_CURVE ( 'NONE', #5984, #11745, #7358, .T. ) ;
#2417=CARTESIAN_POINT ( 'NONE',  ( 2.848727059636059433, -5.281416301279842962, 12.11442521571937192 ) ) ;
#2418=CARTESIAN_POINT ( 'NONE',  ( 2.840966774240121673, -5.567223638426926691, 24.23809786915986919 ) ) ;
#2420=CARTESIAN_POINT ( 'NONE',  ( -3.779082820360738282, 4.979770177899218275, 12.50004906876531230 ) ) ;
#2421=CARTESIAN_POINT ( 'NONE',  ( 0.2622916576877915573, -5.995491482261821048, 18.97384942646813144 ) ) ;
#2426=CARTESIAN_POINT ( 'NONE',  ( 5.726049995854516794, -2.506679546901767974, 17.20045537531157365 ) ) ;
#2430=B_SPLINE_CURVE_WITH_KNOTS ( 'NONE', 3,
 ( #1775, #12825, #891, #2084, #11638, #12747, #11790, #4246, #13945, #2008, #740, #818, #9335, #5606, #10453, #15306, #9263, #6882 ),
 .UNSPECIFIED., .F., .F.,
 ( 4, 2, 2, 2, 2, 2, 2, 2, 4 ),
 ( 0.003131918686235953507, 0.003523310662250245945, 0.003914702638264538383, 0.004306094614278830821, 0.004697486590293124126, 0.005088878566307415696, 0.005480270542321709001, 0.005871662518336001439, 0.006263054494350293877 ),
 .UNSPECIFIED. ) ;
#2431=CARTESIAN_POINT ( 'NONE',  ( -5.317509234263937401, 2.779225709351033746, 11.63061695532135786 ) ) ;
#2432=CARTESIAN_POINT ( 'NONE',  ( -0.1323602877611484707, -6.000000000000003553, 12.49999999999998401 ) ) ;
#2435=EDGE_LOOP ( 'NONE', ( #12638, #13087 ) ) ;
#2438=B_SPLINE_CURVE_WITH_KNOTS ( 'NONE', 3,
 ( #11494, #668, #14793, #12393, #10236, #10391, #5620, #11728, #15164, #754, #9052, #14038, #15240, #6895, #3879, #6817, #12690, #4261 ),
 .UNSPECIFIED., .F., .F.,
 ( 4, 2, 2, 2, 2, 2, 2, 2, 4 ),
 ( 0.000000000000000000, 0.0003914357524127461845, 0.0007828715048254923691, 0.001174307257238238608, 0.001565743009650985822, 0.001957178762063732820, 0.002348614514476479818, 0.002740050266889227683, 0.003131486019301974247 ),
 .UNSPECIFIED. ) ;
#2439=CARTESIAN_POINT ( 'NONE',  ( -4.286401442266639883, 4.198423832313084247, 11.36938304467859417 ) ) ;
#2441=CARTESIAN_POINT ( 'NONE',  ( 5.375913338529100471, -2.664979843780421298, 4.495710796379801977 ) ) ;
#2443=CARTESIAN_POINT ( 'NONE',  ( -0.7995524673975431540, -6.199337389817270783, 31.61453679452459653 ) ) ;
#2445=CARTESIAN_POINT ( 'NONE',  ( -5.940390500375820615, 6.474944468551430354, 24.49999999999999289 ) ) ;
#2448=EDGE_CURVE ( 'NONE', #1252, #7643, #15534, .T. ) ;
#2450=ORIENTED_EDGE ( 'NONE', *, *, #12036, .T. ) ;
#2456=CARTESIAN_POINT ( 'NONE',  ( -4.286401442266675410, -4.198423832313046944, 24.49999999999999289 ) ) ;
#2458=DIRECTION ( 'NONE',  ( -0.5877852522924685852, -0.8090169943749507819, 0.000000000000000000 ) ) ;
#2459=VECTOR ( 'NONE', #14120, 1000.000000000000114 ) ;
#2462=CARTESIAN_POINT ( 'NONE',  ( 3.011899281037340614, 5.190111395030321262, 18.80022217383878669 ) ) ;
#2465=CARTESIAN_POINT ( 'NONE',  ( 5.866817325727516241, -1.260653813891924546, 31.80022217383877248 ) ) ;
#2466=CARTESIAN_POINT ( 'NONE',  ( -3.883588957979242640, 4.898466244118940160, 30.02622717124731722 ) ) ;
#2467=CARTESIAN_POINT ( 'NONE',  ( 5.915699123067152954, 1.003533581835587274, 4.496102049840166259 ) ) ;
#2469=CARTESIAN_POINT ( 'NONE',  ( -5.915653884842715371, 1.003805156977378932, 30.49560239355786351 ) ) ;
#2470=B_SPLINE_CURVE_WITH_KNOTS ( 'NONE', 3,
 ( #11598, #11910, #13026, #12949, #11827, #697, #15191, #7947, #13105, #14140, #3170, #4289, #12787, #2205, #9379, #7074, #14217, #9153 ),
 .UNSPECIFIED., .F., .F.,
 ( 4, 2, 2, 2, 2, 2, 2, 2, 4 ),
 ( 0.000000000000000000, 0.0003914898357794963568, 0.0007829796715589927136, 0.001174469507338488962, 0.001565959343117985427, 0.001957449178897482760, 0.002348939014676979225, 0.002740428850456475256, 0.003131918686235972155 ),
 .UNSPECIFIED. ) ;
#2471=ORIENTED_EDGE ( 'NONE', *, *, #4839, .F. ) ;
#2472=ORIENTED_EDGE ( 'NONE', *, *, #12897, .F. ) ;
#2474=CARTESIAN_POINT ( 'NONE',  ( -2.668367453516892418, 5.373994336898001656, 24.63239388001634111 ) ) ;
#2476=B_SPLINE_CURVE_WITH_KNOTS ( 'NONE', 3,
 ( #10656, #2133, #4381, #11764, #5733, #4455, #11610, #14299, #709, #7959, #8119, #9310, #14225, #3408, #12799, #15437, #9387, #10427 ),
 .UNSPECIFIED., .F., .F.,
 ( 4, 2, 2, 2, 2, 2, 2, 2, 4 ),
 ( 0.003131486019301992028, 0.003522824630466699167, 0.003914163241631405873, 0.004305501852796113013, 0.004696840463960820153, 0.005088179075125527293, 0.005479517686290232698, 0.005870856297454939837, 0.006262194908619645242 ),
 .UNSPECIFIED. ) ;
#2479=CARTESIAN_POINT ( 'NONE',  ( -6.105925084677672920, -1.337450587213226072, 12.29933148907575990 ) ) ;
#2485=CARTESIAN_POINT ( 'NONE',  ( -5.866923913994654072, 1.260079467906490391, 31.79952054102715309 ) ) ;
#2486=CARTESIAN_POINT ( 'NONE',  ( 4.267558728637244059, -4.217879122113751933, 31.26382603205595601 ) ) ;
#2488=FACE_OUTER_BOUND ( 'NONE', #14030, .T. ) ;
#2490=CARTESIAN_POINT ( 'NONE',  ( 6.176542424588107316, 0.9554180641286319497, 5.130606907234995795 ) ) ;
#2491=ORIENTED_EDGE ( 'NONE', *, *, #11796, .F. ) ;
#2493=VECTOR ( 'NONE', #6616, 1000.000000000000114 ) ;
#2494=ORIENTED_EDGE ( 'NONE', *, *, #13420, .F. ) ;
#2495=VERTEX_POINT ( 'NONE', #9179 ) ;
#2500=EDGE_CURVE ( 'NONE', #7716, #4668, #5113, .T. ) ;
#2501=CARTESIAN_POINT ( 'NONE',  ( 2.668367453516645504, -5.373994336898123336, 11.49999999999998224 ) ) ;
#2503=CARTESIAN_POINT ( 'NONE',  ( 4.435347140100927454, -4.403429997944614982, 24.36762589283694069 ) ) ;
#2505=CARTESIAN_POINT ( 'NONE',  ( -4.344762547369766637, 4.493114738039160727, 10.99691356133951992 ) ) ;
#2506=CARTESIAN_POINT ( 'NONE',  ( 0.6152055445547642831, -5.969096820685141580, 18.79904968670266996 ) ) ;
#2508=EDGE_CURVE ( 'NONE', #1119, #4626, #12680, .T. ) ;
#2512=AXIS2_PLACEMENT_3D ( 'NONE', #12106, #1207, #6078 ) ;
#2514=CARTESIAN_POINT ( 'NONE',  ( 5.935543223013856284, 0.8771126767606806096, 11.49999999999998224 ) ) ;
#2516=VERTEX_POINT ( 'NONE', #1843 ) ;
#2517=DIRECTION ( 'NONE',  ( -1.000000000000000000, 0.000000000000000000, 0.000000000000000000 ) ) ;
#2519=CARTESIAN_POINT ( 'NONE',  ( 5.409423237179071364, 2.597448116730906253, 25.11561732698605098 ) ) ;
#2525=CARTESIAN_POINT ( 'NONE',  ( -0.8730628416137050651, -6.188929913094965762, 30.49504929893117122 ) ) ;
#2527=FACE_BOUND ( 'NONE', #12681, .T. ) ;
#2531=LINE ( 'NONE', #7386, #7975 ) ;
#2532=VECTOR ( 'NONE', #3932, 1000.000000000000000 ) ;
#2535=EDGE_CURVE ( 'NONE', #9028, #13870, #1855, .T. ) ;
#2537=CARTESIAN_POINT ( 'NONE',  ( 5.375886393124428508, 2.665038680141196270, 23.99560239355785640 ) ) ;
#2538=CARTESIAN_POINT ( 'NONE',  ( 2.817313151351089839, 5.579000502529481764, 31.00000000000000000 ) ) ;
#2541=CARTESIAN_POINT ( 'NONE',  ( 0.6139731865241975228, -6.220476368274032275, 23.69975545601931799 ) ) ;
#2542=EDGE_CURVE ( 'NONE', #3463, #3038, #10755, .T. ) ;
#2545=CARTESIAN_POINT ( 'NONE',  ( 5.935543223013889147, -0.8771126767604601193, 24.49999999999999289 ) ) ;
#2547=DIRECTION ( 'NONE',  ( -0.9510565162951544194, 0.3090169943749447312, 0.000000000000000000 ) ) ;
#2548=CARTESIAN_POINT ( 'NONE',  ( 5.620786884546307149, -2.102685372472853143, 31.97358595436693918 ) ) ;
#2549=CARTESIAN_POINT ( 'NONE',  ( -0.2623718222033848413, -6.245654667075791089, 17.02627829713834018 ) ) ;
#2551=CARTESIAN_POINT ( 'NONE',  ( 5.409423237179016297, 2.597448116731026602, 12.11561732698603855 ) ) ;
#2552=EDGE_LOOP ( 'NONE', ( #4370, #493, #15450, #8595 ) ) ;
#2557=ORIENTED_EDGE ( 'NONE', *, *, #14453, .T. ) ;
#2560=CARTESIAN_POINT ( 'NONE',  ( 6.155973317223280894, 1.081218830693758903, 31.50308643866045344 ) ) ;
#2563=CARTESIAN_POINT ( 'NONE',  ( -5.375605342016520183, 2.665598297262264715, 31.50312048902376816 ) ) ;
#2564=CARTESIAN_POINT ( 'NONE',  ( -7.799024015210663130, -1.482594289697217294, 5.000000000000004441 ) ) ;
#2566=CARTESIAN_POINT ( 'NONE',  ( 6.123233995736766282E-16, -6.250000000000000888, 5.000000000000004441 ) ) ;
#2568=ORIENTED_EDGE ( 'NONE', *, *, #6631, .F. ) ;
#2573=CARTESIAN_POINT ( 'NONE',  ( 2.817313151351107159, 5.579000502529472882, 4.869393092765015751 ) ) ;
#2574=CARTESIAN_POINT ( 'NONE',  ( -0.2624013748573160165, -5.995472630654518298, 4.026285596910829767 ) ) ;
#2575=CARTESIAN_POINT ( 'NONE',  ( -4.267838854167186113, -4.217593933790326766, 18.26239891805597537 ) ) ;
#2576=CARTESIAN_POINT ( 'NONE',  ( 0.7995298244855156833, 5.947211616899241271, 12.11456014619857946 ) ) ;
#2578=CARTESIAN_POINT ( 'NONE',  ( 5.409274167810689704, -2.597759609440573492, 12.11519382448850557 ) ) ;
#2580=LINE ( 'NONE', #7363, #10244 ) ;
#2583=AXIS2_PLACEMENT_3D ( 'NONE', #10617, #9196, #6737 ) ;
#2586=EDGE_CURVE ( 'NONE', #6402, #4624, #13832, .T. ) ;
#2588=VERTEX_POINT ( 'NONE', #4558 ) ;
#2589=CARTESIAN_POINT ( 'NONE',  ( -3.311384659207134984, 5.004923837169420686, 5.973585954366940953 ) ) ;
#2590=CARTESIAN_POINT ( 'NONE',  ( -5.558508435838217743, 2.857531096718874952, 30.86936067245787640 ) ) ;
#2596=CARTESIAN_POINT ( 'NONE',  ( -2.931212650151840293, 5.520239928492722825, 23.99574050496988065 ) ) ;
#2597=LINE ( 'NONE', #1396, #109 ) ;
#2600=EDGE_CURVE ( 'NONE', #6522, #6002, #2249, .T. ) ;
#2603=AXIS2_PLACEMENT_3D ( 'NONE', #14738, #13220, #3825 ) ;
#2607=B_SPLINE_CURVE_WITH_KNOTS ( 'NONE', 3,
 ( #12396, #14796, #8755, #7630, #10099, #13587, #1496, #11207, #11285, #5015, #308, #382, #5169, #10022, #3960, #8834, #2269, #7140 ),
 .UNSPECIFIED., .F., .F.,
 ( 4, 2, 2, 2, 2, 2, 2, 2, 4 ),
 ( 0.003131918686235974757, 0.003523310662250265460, 0.003914702638264555730, 0.004306094614278846433, 0.004697486590293137136, 0.005088878566307427839, 0.005480270542321717675, 0.005871662518336008378, 0.006263054494350299081 ),
 .UNSPECIFIED. ) ;
#2609=CARTESIAN_POINT ( 'NONE',  ( -3.735642931251144994, 4.696778275484382092, 18.97408052783099563 ) ) ;
#2610=EDGE_CURVE ( 'NONE', #3990, #13214, #1100, .T. ) ;
#2612=EDGE_LOOP ( 'NONE', ( #12888, #3745 ) ) ;
#2613=CARTESIAN_POINT ( 'NONE',  ( -3.311384659207235792, -5.004923837169353185, 23.52641404563305016 ) ) ;
#2614=CARTESIAN_POINT ( 'NONE',  ( 5.940390500375496430, 6.474944468551661281, 11.49999999999998224 ) ) ;
#2616=EDGE_CURVE ( 'NONE', #7910, #4035, #11161, .T. ) ;
#2617=CARTESIAN_POINT ( 'NONE',  ( 5.649053410273082498, -2.675685104943239523, 31.61517780375841369 ) ) ;
#2620=CARTESIAN_POINT ( 'NONE',  ( 5.317509234264064411, -2.779225709350791274, 24.49999999999999289 ) ) ;
#2624=CARTESIAN_POINT ( 'NONE',  ( -5.317509234263939177, 2.779225709351033302, 11.49999999999998224 ) ) ;
#2625=CARTESIAN_POINT ( 'NONE',  ( -5.317509234263898321, -2.779225709351108797, 11.63064961348853465 ) ) ;
#2626=CARTESIAN_POINT ( 'NONE',  ( 3.922396193918885832, 4.541970110199584632, 23.62619317285288645 ) ) ;
#2627=ORIENTED_EDGE ( 'NONE', *, *, #10989, .T. ) ;
#2631=ORIENTED_EDGE ( 'NONE', *, *, #1073, .T. ) ;
#2632=ORIENTED_EDGE ( 'NONE', *, *, #12161, .F. ) ;
#2633=CARTESIAN_POINT ( 'NONE',  ( -5.935543223013816316, -0.8771126767609508379, 24.49999999999999289 ) ) ;
#2634=ORIENTED_EDGE ( 'NONE', *, *, #4191, .F. ) ;
#2636=B_SPLINE_CURVE_WITH_KNOTS ( 'NONE', 3,
 ( #10897, #7395, #13508, #1181, #2617, #4776, #1448, #3648, #229, #7472, #12238, #1339, #11571, #597, #12921, #1492, #13960, #4182 ),
 .UNSPECIFIED., .F., .F.,
 ( 4, 2, 2, 2, 2, 2, 2, 2, 4 ),
 ( 0.000000000000000000, 0.0003914357524127471061, 0.0007828715048254942122, 0.001174307257238241427, 0.001565743009650988424, 0.001957178762063735422, 0.002348614514476482854, 0.002740050266889229851, 0.003131486019301976849 ),
 .UNSPECIFIED. ) ;
#2637=CARTESIAN_POINT ( 'NONE',  ( -5.558508435838158235, -2.857531096718993524, 11.63063932754212892 ) ) ;
#2640=VECTOR ( 'NONE', #3726, 1000.000000000000000 ) ;
#2643=FACE_OUTER_BOUND ( 'NONE', #6380, .T. ) ;
#2645=CARTESIAN_POINT ( 'NONE',  ( 4.267936573529233613, 4.217499624512214496, 5.262290378359326226 ) ) ;
#2647=CARTESIAN_POINT ( 'NONE',  ( 6.106056299406760424, -1.336851112280608378, 10.70112161576659560 ) ) ;
#2650=ORIENTED_EDGE ( 'NONE', *, *, #3508, .F. ) ;
#2652=ORIENTED_EDGE ( 'NONE', *, *, #4161, .T. ) ;
#2654=CARTESIAN_POINT ( 'NONE',  ( 3.780072143464216605, 4.979057943639748629, 3.999917806784441865 ) ) ;
#2655=CARTESIAN_POINT ( 'NONE',  ( 0.8738239080080354437, 6.188820299975593464, 5.503557957101424591 ) ) ;
#2656=CARTESIAN_POINT ( 'NONE',  ( 0.5044069930203494145, -5.979990686694992341, 31.87335743227903606 ) ) ;
#2657=CARTESIAN_POINT ( 'NONE',  ( 0.1306171417089282139, 6.000000000000000000, 10.49999999999998401 ) ) ;
#2660=CARTESIAN_POINT ( 'NONE',  ( -6.155854678529491864, 1.081900940642012587, 5.504259495030091820 ) ) ;
#2661=CARTESIAN_POINT ( 'NONE',  ( -2.668367453516813814, -5.373994336898041624, 24.49999999999999289 ) ) ;
#2666=AXIS2_PLACEMENT_3D ( 'NONE', #1854, #8067, #9265 ) ;
#2669=ORIENTED_EDGE ( 'NONE', *, *, #6985, .T. ) ;
#2671=CARTESIAN_POINT ( 'NONE',  ( -6.172639027853100480, 0.9816353142772724638, 24.23774718278285789 ) ) ;
#2673=CARTESIAN_POINT ( 'NONE',  ( 5.770331821586383469, 2.404225004693643086, 30.12619944752605150 ) ) ;
#2675=CARTESIAN_POINT ( 'NONE',  ( -4.435347140101024266, -4.403429997944519947, 31.00000000000000000 ) ) ;
#2677=CARTESIAN_POINT ( 'NONE',  ( 5.665707375537461843, -1.979196487016705586, 3.999920388255239434 ) ) ;
#2679=CARTESIAN_POINT ( 'NONE',  ( 6.768587589771821120E-14, -6.250000000000000888, 12.49999999999998401 ) ) ;
#2684=CARTESIAN_POINT ( 'NONE',  ( 3.568242062701468598, 5.132954954975548212, 12.50004906876531052 ) ) ;
#2687=CARTESIAN_POINT ( 'NONE',  ( -5.746837578675960678, -1.729433780394401099, 18.99995053646221521 ) ) ;
#2690=ORIENTED_EDGE ( 'NONE', *, *, #7017, .F. ) ;
#2691=CARTESIAN_POINT ( 'NONE',  ( -2.931156713028501670, -5.520271803279203304, 17.49563030319846746 ) ) ;
#2693=CARTESIAN_POINT ( 'NONE',  ( 5.558508435838260375, -2.857531096718793240, 11.49999999999998224 ) ) ;
#2696=CARTESIAN_POINT ( 'NONE',  ( -5.866984344570858489, 1.259800266528510182, 4.200681937418259793 ) ) ;
#2698=CARTESIAN_POINT ( 'NONE',  ( 5.746619684944337614, -1.730157667110624908, 25.50004932073311892 ) ) ;
#2703=CARTESIAN_POINT ( 'NONE',  ( -4.344762547369738215, 4.493114738039190925, 30.49691356133954301 ) ) ;
#2705=CARTESIAN_POINT ( 'NONE',  ( -5.317509234263900098, -2.779225709351109241, 11.36938304467859417 ) ) ;
#2708=ORIENTED_EDGE ( 'NONE', *, *, #8523, .F. ) ;
#2709=DIRECTION ( 'NONE',  ( 0.5877852522924802425, -0.8090169943749422332, 0.000000000000000000 ) ) ;
#2711=CARTESIAN_POINT ( 'NONE',  ( -4.267992336621335703, 4.217442018459861330, 24.76194324003146008 ) ) ;
#2713=AXIS2_PLACEMENT_3D ( 'NONE', #1872, #6669, #8091 ) ;
#2722=CARTESIAN_POINT ( 'NONE',  ( 2.848727059636091408, -5.281416301279826087, 31.61442521571938258 ) ) ;
#2724=CARTESIAN_POINT ( 'NONE',  ( 6.176542424588128632, -0.9554180641284775177, 11.49999999999998224 ) ) ;
#2729=EDGE_CURVE ( 'NONE', #3463, #7351, #6098, .T. ) ;
#2730=CARTESIAN_POINT ( 'NONE',  ( 5.487097279078454015, -2.429065649168769436, 30.20047945897283981 ) ) ;
#2734=CARTESIAN_POINT ( 'NONE',  ( -0.7988914244718240409, -5.947301735519284094, 4.384562891686187847 ) ) ;
#2735=CARTESIAN_POINT ( 'NONE',  ( 0.8737888311110264539, -5.936248257219505220, 31.50344185141217679 ) ) ;
#2739=SURFACE_SIDE_STYLE ('',( #4002 ) ) ;
#2741=CYLINDRICAL_SURFACE ( 'NONE', #14104, 1.000000000000000888 ) ;
#2742=CARTESIAN_POINT ( 'NONE',  ( 0.8736516769108820801, -5.936271176698206808, 23.99606771578674369 ) ) ;
#2749=ORIENTED_EDGE ( 'NONE', *, *, #51, .T. ) ;
#2750=CARTESIAN_POINT ( 'NONE',  ( -2.782713018890638157, 5.315928322779165605, 5.504397606442132940 ) ) ;
#2751=CARTESIAN_POINT ( 'NONE',  ( 4.435347140101024266, -4.403429997944519947, 11.36762589283694425 ) ) ;
#2752=CARTESIAN_POINT ( 'NONE',  ( 0.9740856415301589744, -6.173834621338581741, 11.23852653055533857 ) ) ;
#2753=CARTESIAN_POINT ( 'NONE',  ( -7.490007020835664164, -2.433650805992495503, 17.99999999999998934 ) ) ;
#2754=CYLINDRICAL_SURFACE ( 'NONE', #4874, 0.9999999999999998890 ) ;
#2755=CIRCLE ( 'NONE', #11641, 6.000000000000000888 ) ;
#2756=FACE_BOUND ( 'NONE', #4547, .T. ) ;
#2760=DIRECTION ( 'NONE',  ( 0.9510565162951500895, 0.3090169943749582204, 0.000000000000000000 ) ) ;
#2762=FACE_BOUND ( 'NONE', #11521, .T. ) ;
#2769=CARTESIAN_POINT ( 'NONE',  ( -2.692215568229928468, 5.362327947133553430, 18.26229037835931379 ) ) ;
#2772=ORIENTED_EDGE ( 'NONE', *, *, #9307, .T. ) ;
#2773=CARTESIAN_POINT ( 'NONE',  ( -4.291255145204092791, -4.544933371694659385, 17.38603820591928439 ) ) ;
#2781=CARTESIAN_POINT ( 'NONE',  ( 6.143143148203054515, -1.154591847827728390, 5.613961794080713830 ) ) ;
#2782=DIRECTION ( 'NONE',  ( -0.3090169943749447867, -0.9510565162951544194, 0.000000000000000000 ) ) ;
#2783=CARTESIAN_POINT ( 'NONE',  ( 4.267558728637053100, 4.217879122113947332, 24.23617396794403334 ) ) ;
#2784=EDGE_LOOP ( 'NONE', ( #6710, #2749, #1117, #11930 ) ) ;
#2787=VERTEX_POINT ( 'NONE', #1748 ) ;
#2788=CARTESIAN_POINT ( 'NONE',  ( 5.940390500375443139, 6.474944468551700361, 17.99999999999998934 ) ) ;
#2795=CARTESIAN_POINT ( 'NONE',  ( -2.817313151351189315, 5.579000502529432026, 4.867658743658316745 ) ) ;
#2799=CARTESIAN_POINT ( 'NONE',  ( -3.420311045507932857, 4.931422832349230845, 16.99992038825522656 ) ) ;
#2802=CARTESIAN_POINT ( 'NONE',  ( 4.286401442266532413, 4.198423832313196158, 5.000000000000004441 ) ) ;
#2804=CARTESIAN_POINT ( 'NONE',  ( -6.021167129161077547, 1.680051667990220432, 30.02640428276698259 ) ) ;
#2806=B_SPLINE_CURVE_WITH_KNOTS ( 'NONE', 3,
 ( #3933, #11338, #8892, #10230, #9919, #5145, #1703, #2909, #13637, #13874, #2752, #6505, #2986, #4177, #7759, #12686, #14772, #7603 ),
 .UNSPECIFIED., .F., .F.,
 ( 4, 2, 2, 2, 2, 2, 2, 2, 4 ),
 ( 0.000000000000000000, 0.0003914362731607611522, 0.0007828725463215223043, 0.001174308819482283456, 0.001565745092643044609, 0.001957181365803805761, 0.002348617638964566913, 0.002740053912125328065, 0.003131490185286089217 ),
 .UNSPECIFIED. ) ;
#2807=EDGE_CURVE ( 'NONE', #5516, #5575, #15389, .T. ) ;
#2809=EDGE_LOOP ( 'NONE', ( #15512, #3317, #2949, #4891 ) ) ;
#2811=ORIENTED_EDGE ( 'NONE', *, *, #4181, .F. ) ;
#2815=CARTESIAN_POINT ( 'NONE',  ( -4.006441409774754270, -4.467329318258197901, 18.79888242247939800 ) ) ;
#2816=CARTESIAN_POINT ( 'NONE',  ( -0.6151877315909333177, 6.220340188096021627, 18.79906673469662337 ) ) ;
#2817=CARTESIAN_POINT ( 'NONE',  ( 5.571002711501426674, -2.833546409886251283, 30.73620383159192571 ) ) ;
#2819=CARTESIAN_POINT ( 'NONE',  ( -6.176542424588110869, 0.9554180641286129649, 11.49999999999998224 ) ) ;
#2820=CARTESIAN_POINT ( 'NONE',  ( -4.290821322214440237, 4.545321419741492619, 10.88558052754513383 ) ) ;
#2821=EDGE_CURVE ( 'NONE', #10136, #13172, #8945, .T. ) ;
#2822=CARTESIAN_POINT ( 'NONE',  ( 3.419318284370178596, 4.932111238568190892, 10.50007997643736424 ) ) ;
#2827=B_SPLINE_CURVE_WITH_KNOTS ( 'NONE', 3,
 ( #13316, #2657, #1377, #7511, #3842, #6251, #13474, #12278, #3609, #1297, #7588, #11243, #2576, #14758, #111, #12355, #11167, #13548 ),
 .UNSPECIFIED., .F., .F.,
 ( 4, 2, 2, 2, 2, 2, 2, 2, 4 ),
 ( 0.003131923598876996170, 0.003523316383094313078, 0.003914709167311630419, 0.004306101951528947328, 0.004697494735746264236, 0.005088887519963581144, 0.005480280304180898052, 0.005871673088398214960, 0.006263065872615531868 ),
 .UNSPECIFIED. ) ;
#2829=EDGE_CURVE ( 'NONE', #10051, #13722, #2476, .T. ) ;
#2830=VERTEX_POINT ( 'NONE', #8278 ) ;
#2831=CARTESIAN_POINT ( 'NONE',  ( -4.267992336621191818, 4.217442018460005215, 5.261943240031468960 ) ) ;
#2833=CARTESIAN_POINT ( 'NONE',  ( -3.107583187530600810, 5.133966411712579614, 23.62619317285289000 ) ) ;
#2834=CARTESIAN_POINT ( 'NONE',  ( 6.143020266950977692, 1.155160780047711944, 12.11441947245482353 ) ) ;
#2835=DIRECTION ( 'NONE',  ( -0.5877852522924685852, -0.8090169943749508930, 0.000000000000000000 ) ) ;
#2837=CARTESIAN_POINT ( 'NONE',  ( -2.931212650151596932, -5.520239928492851611, 31.50425949503010514 ) ) ;
#2838=VECTOR ( 'NONE', #5540, 1000.000000000000114 ) ;
#2842=CYLINDRICAL_SURFACE ( 'NONE', #13854, 1.000000000000000666 ) ;
#2844=FACE_BOUND ( 'NONE', #12793, .T. ) ;
#2847=CARTESIAN_POINT ( 'NONE',  ( -2.931156713028435501, -5.520271803279239720, 10.99563030319846746 ) ) ;
#2850=LINE ( 'NONE', #5244, #10363 ) ;
#2853=DIRECTION ( 'NONE',  ( 0.000000000000000000, 1.000000000000000000, 0.000000000000000000 ) ) ;
#2854=DIRECTION ( 'NONE',  ( 0.8090169943749510040, -0.5877852522924683631, 0.000000000000000000 ) ) ;
#2855=CARTESIAN_POINT ( 'NONE',  ( -5.931817299736865223, 0.9033986943601339803, 4.737709621640688873 ) ) ;
#2860=CARTESIAN_POINT ( 'NONE',  ( -2.849573632035271586, 5.280958870664604454, 30.38438267301394902 ) ) ;
#2862=CARTESIAN_POINT ( 'NONE',  ( -5.915641100987811818, -1.003868594704857342, 10.99571079637978599 ) ) ;
#2865=ORIENTED_EDGE ( 'NONE', *, *, #13918, .T. ) ;
#2866=CARTESIAN_POINT ( 'NONE',  ( -5.317509234263837037, -2.779225709351230922, 24.36938304467860306 ) ) ;
#2867=ORIENTED_EDGE ( 'NONE', *, *, #7594, .T. ) ;
#2868=VECTOR ( 'NONE', #1926, 1000.000000000000114 ) ;
#2869=CARTESIAN_POINT ( 'NONE',  ( 7.799024015210672900, -1.482594289696959944, 17.99999999999998934 ) ) ;
#2870=CARTESIAN_POINT ( 'NONE',  ( 7.490007020835748541, -2.433650805992050969, 24.49999999999999289 ) ) ;
#2871=ORIENTED_EDGE ( 'NONE', *, *, #6631, .T. ) ;
#2873=CARTESIAN_POINT ( 'NONE',  ( -4.416678568553696671, 4.422441866694263979, 4.737630265561251441 ) ) ;
#2879=CARTESIAN_POINT ( 'NONE',  ( -4.286401442266688733, 4.198423832313033621, 17.99999999999998934 ) ) ;
#2880=DIRECTION ( 'NONE',  ( 0.000000000000000000, 0.000000000000000000, 1.000000000000000000 ) ) ;
#2882=CARTESIAN_POINT ( 'NONE',  ( -0.8736772044959679739, 6.188841968496064716, 30.49611573292809652 ) ) ;
#2886=CARTESIAN_POINT ( 'NONE',  ( 0.8738118504727017122, 5.936246475285011925, 18.50357242174242245 ) ) ;
#2887=CARTESIAN_POINT ( 'NONE',  ( 5.649053410273043418, 2.675685104943323012, 4.384822196241565884 ) ) ;
#2889=CARTESIAN_POINT ( 'NONE',  ( -6.172552660730961094, -0.9821660343539843074, 17.73620383159192926 ) ) ;
#2890=CIRCLE ( 'NONE', #12790, 6.250000000000000888 ) ;
#2891=CARTESIAN_POINT ( 'NONE',  ( 0.5039005892422661059, -6.230833003620530164, 17.12636388911296592 ) ) ;
#2893=CARTESIAN_POINT ( 'NONE',  ( -0.1306394121197964608, 6.250000000000004441, 16.99999999999998934 ) ) ;
#2897=EDGE_CURVE ( 'NONE', #860, #15705, #2270, .T. ) ;
#2906=DIRECTION ( 'NONE',  ( 1.000000000000000000, 0.000000000000000000, 0.000000000000000000 ) ) ;
#2909=CARTESIAN_POINT ( 'NONE',  ( 0.9735954530125885409, -6.173909381473981384, 11.76281793585243918 ) ) ;
#2910=CARTESIAN_POINT ( 'NONE',  ( 5.558508435838221295, 2.857531096718871844, 11.49999999999998224 ) ) ;
#2912=CARTESIAN_POINT ( 'NONE',  ( 3.632753594129220165, -4.777047695051066967, 23.50004946353777413 ) ) ;
#2914=CARTESIAN_POINT ( 'NONE',  ( 4.286401442266532413, 4.198423832313196158, 5.000000000000004441 ) ) ;
#2917=CARTESIAN_POINT ( 'NONE',  ( 5.903230462362944131, 1.077253041748938989, 5.614425215719392348 ) ) ;
#2922=CARTESIAN_POINT ( 'NONE',  ( 5.858736126997225568, -2.179962889276819027, 25.47359571723300675 ) ) ;
#2927=CARTESIAN_POINT ( 'NONE',  ( -5.931817299736830584, -0.9033986943603558029, 18.26229037835932090 ) ) ;
#2930=CARTESIAN_POINT ( 'NONE',  ( -2.997451966578457139, -5.485105005465983119, 17.38482219624156855 ) ) ;
#2932=CARTESIAN_POINT ( 'NONE',  ( 6.081590040723096280, -1.446205118472926099, 12.37367328635990837 ) ) ;
#2937=DIRECTION ( 'NONE',  ( -0.5877852522924685852, -0.8090169943749507819, 0.000000000000000000 ) ) ;
#2938=CARTESIAN_POINT ( 'NONE',  ( -0.8737888311109888173, 5.936248257219512325, 31.50344185141217679 ) ) ;
#2940=CARTESIAN_POINT ( 'NONE',  ( 6.155912734541134412, -1.081577393120893182, 5.503892131249681796 ) ) ;
#2947=VERTEX_POINT ( 'NONE', #7005 ) ;
#2949=ORIENTED_EDGE ( 'NONE', *, *, #12636, .T. ) ;
#2950=CARTESIAN_POINT ( 'NONE',  ( -2.668367453516630849, -5.373994336898131330, 5.132360785839114925 ) ) ;
#2953=CARTESIAN_POINT ( 'NONE',  ( -2.931212650151651555, 5.520239928492821413, 4.495740504969916174 ) ) ;
#2957=CYLINDRICAL_SURFACE ( 'NONE', #1104, 0.9999999999999998890 ) ;
#2958=CARTESIAN_POINT ( 'NONE',  ( -5.615973259022225328, -2.743340227996369673, 25.00389213124970311 ) ) ;
#2960=CARTESIAN_POINT ( 'NONE',  ( 2.668367453516568677, 5.373994336898162416, 11.49999999999998224 ) ) ;
#2965=CARTESIAN_POINT ( 'NONE',  ( 4.069800786343793497, -4.744882212776830421, 12.37381964045070681 ) ) ;
#2966=LINE ( 'NONE', #1683, #10890 ) ;
#2970=CARTESIAN_POINT ( 'NONE',  ( -5.842988226680587260, 1.369004370660612313, 5.873806827147107334 ) ) ;
#2971=CARTESIAN_POINT ( 'NONE',  ( 0.1306070469494795272, 6.249999999999999112, 16.99999999999998579 ) ) ;
#2973=DIRECTION ( 'NONE',  ( 0.8090169943749421222, 0.5877852522924802425, 0.000000000000000000 ) ) ;
#2981=EDGE_CURVE ( 'NONE', #15355, #159, #8173, .T. ) ;
#2983=EDGE_LOOP ( 'NONE', ( #8310, #11623 ) ) ;
#2985=CARTESIAN_POINT ( 'NONE',  ( -4.435347140101170815, 4.403429997944374286, 17.86939309276499799 ) ) ;
#2986=CARTESIAN_POINT ( 'NONE',  ( 0.8002720181891768148, -6.199262377003395663, 10.88606262465556895 ) ) ;
#2988=DIRECTION ( 'NONE',  ( 0.8090169943749506709, -0.5877852522924686962, 0.000000000000000000 ) ) ;
#2989=ADVANCED_FACE ( 'NONE', ( #12004 ), #11129, .F. ) ;
#2998=CARTESIAN_POINT ( 'NONE',  ( 6.106056299406778187, -1.336851112280531995, 17.20112161576660981 ) ) ;
#3000=ADVANCED_FACE ( 'NONE', ( #1199 ), #10815, .F. ) ;
#3006=ORIENTED_EDGE ( 'NONE', *, *, #14994, .T. ) ;
#3007=LINE ( 'NONE', #14944, #3307 ) ;
#3008=CARTESIAN_POINT ( 'NONE',  ( 3.107278289587024567, 5.134157760522150227, 25.37364704684422279 ) ) ;
#3012=LINE ( 'NONE', #5488, #456 ) ;
#3013=CARTESIAN_POINT ( 'NONE',  ( -5.317509234263930296, -2.779225709351048401, 5.000000000000004441 ) ) ;
#3016=CARTESIAN_POINT ( 'NONE',  ( 6.143020266951017661, -1.155160780047501445, 23.88558052754514804 ) ) ;
#3019=EDGE_LOOP ( 'NONE', ( #10341, #3265 ) ) ;
#3021=ORIENTED_EDGE ( 'NONE', *, *, #8094, .F. ) ;
#3022=CARTESIAN_POINT ( 'NONE',  ( -5.903057025253887424, 1.078199533779612640, 25.11561732698604388 ) ) ;
#3023=ORIENTED_EDGE ( 'NONE', *, *, #13034, .F. ) ;
#3024=ADVANCED_FACE ( 'NONE', ( #3492 ), #8680, .F. ) ;
#3025=FACE_OUTER_BOUND ( 'NONE', #12229, .T. ) ;
#3026=DIRECTION ( 'NONE',  ( -0.9510565162951545304, 0.3090169943749447867, 0.000000000000000000 ) ) ;
#3029=CARTESIAN_POINT ( 'NONE',  ( -4.196288036172359348, -4.288789315524921264, 5.503120489023787698 ) ) ;
#3030=CARTESIAN_POINT ( 'NONE',  ( 0.8730424326980882332, 5.936362132114464174, 4.495006902185632036 ) ) ;
#3034=CARTESIAN_POINT ( 'NONE',  ( -3.107583187530535529, 5.133966411712619582, 17.12619317285288645 ) ) ;
#3035=DIRECTION ( 'NONE',  ( -0.3090169943749446202, -0.9510565162951544194, 0.000000000000000000 ) ) ;
#3036=CARTESIAN_POINT ( 'NONE',  ( 3.568242062701521444, 5.132954954975510908, 32.00004906876532829 ) ) ;
#3037=CARTESIAN_POINT ( 'NONE',  ( 2.692143549875342767, 5.362363179736505003, 11.76194324003145830 ) ) ;
#3038=VERTEX_POINT ( 'NONE', #14553 ) ;
#3042=CARTESIAN_POINT ( 'NONE',  ( 2.841163418881408553, -5.567120626447921161, 11.76236973443872280 ) ) ;
#3043=CARTESIAN_POINT ( 'NONE',  ( 5.558508435838189321, 2.857531096718932240, 5.000000000000004441 ) ) ;
#3045=CARTESIAN_POINT ( 'NONE',  ( 5.665824935993658329, -1.978765057080782652, 18.99995053646221521 ) ) ;
#3046=B_SPLINE_CURVE_WITH_KNOTS ( 'NONE', 3,
 ( #10711, #11974, #4592, #7372, #3546, #10868, #15647, #14274, #14524, #1001, #6186, #9521, #7139, #1082, #2185, #4749, #3624, #14610 ),
 .UNSPECIFIED., .F., .F.,
 ( 4, 2, 2, 2, 2, 2, 2, 2, 4 ),
 ( 0.003131918686235958278, 0.003523310662250251149, 0.003914702638264544454, 0.004306094614278836892, 0.004697486590293130197, 0.005088878566307422635, 0.005480270542321715940, 0.005871662518336009245, 0.006263054494350301683 ),
 .UNSPECIFIED. ) ;
#3047=CARTESIAN_POINT ( 'NONE',  ( 2.094888798833199608E-14, -6.000000000000000888, 30.00000000000000000 ) ) ;
#3048=CARTESIAN_POINT ( 'NONE',  ( -4.291255145204075916, 4.544933371694674484, 31.61396179408071561 ) ) ;
#3052=CARTESIAN_POINT ( 'NONE',  ( 5.621197618055726153, 2.101623592078383673, 18.97398020122238904 ) ) ;
#3056=CARTESIAN_POINT ( 'NONE',  ( 2.817313151350985034, 5.579000502529534167, 17.99999999999998934 ) ) ;
#3057=ORIENTED_EDGE ( 'NONE', *, *, #6193, .T. ) ;
#3061=CARTESIAN_POINT ( 'NONE',  ( 3.458623254138784908, -5.207221900902769818, 5.973772828752683672 ) ) ;
#3062=LINE ( 'NONE', #12755, #5347 ) ;
#3064=CARTESIAN_POINT ( 'NONE',  ( 5.903596343266329427, 2.055998103990495540, 23.50004921015706216 ) ) ;
#3065=CARTESIAN_POINT ( 'NONE',  ( -5.866984344570831844, 1.259800266528639190, 17.20068193741824558 ) ) ;
#3066=CARTESIAN_POINT ( 'NONE',  ( 5.317509234264027107, 2.779225709350867213, 24.49999999999999289 ) ) ;
#3072=EDGE_CURVE ( 'NONE', #1584, #2830, #8526, .T. ) ;
#3076=B_SPLINE_CURVE_WITH_KNOTS ( 'NONE', 3,
 ( #3288, #8152, #6961, #4569, #9419, #14254, #8230, #7037, #11867, #3970, #13911, #5180, #11448, #3022, #472, #1818, #10186, #4133 ),
 .UNSPECIFIED., .F., .F.,
 ( 4, 2, 2, 2, 2, 2, 2, 2, 4 ),
 ( 0.003131918686235976492, 0.003523310662250265894, 0.003914702638264555730, 0.004306094614278844698, 0.004697486590293134534, 0.005088878566307424370, 0.005480270542321714206, 0.005871662518336004041, 0.006263054494350294744 ),
 .UNSPECIFIED. ) ;
#3077=CARTESIAN_POINT ( 'NONE',  ( 6.143020266950986574, -1.155160780047669755, 30.38558052754516225 ) ) ;
#3080=CYLINDRICAL_SURFACE ( 'NONE', #12155, 1.000000000000000666 ) ;
#3082=ORIENTED_EDGE ( 'NONE', *, *, #1490, .T. ) ;
#3085=B_SPLINE_CURVE_WITH_KNOTS ( 'NONE', 3,
 ( #6561, #14906, #7739, #5289, #14755, #9901, #1375, #11165, #12510, #1533, #11397, #5049, #7509, #14989, #265, #2889, #10058, #11321 ),
 .UNSPECIFIED., .F., .F.,
 ( 4, 2, 2, 2, 2, 2, 2, 2, 4 ),
 ( 0.003131486019301992028, 0.003522824630466698734, 0.003914163241631405006, 0.004305501852796111278, 0.004696840463960818418, 0.005088179075125524690, 0.005479517686290230963, 0.005870856297454938102, 0.006262194908619644375 ),
 .UNSPECIFIED. ) ;
#3092=CARTESIAN_POINT ( 'NONE',  ( 5.571002711501508387, -2.833546409886088302, 24.23620383159193636 ) ) ;
#3093=CARTESIAN_POINT ( 'NONE',  ( -6.176542424588120639, 0.9554180641285460185, 5.000000000000004441 ) ) ;
#3094=VECTOR ( 'NONE', #14694, 1000.000000000000000 ) ;
#3096=ORIENTED_EDGE ( 'NONE', *, *, #4101, .F. ) ;
#3099=CARTESIAN_POINT ( 'NONE',  ( -0.2619456584321428472, 5.995505046955617701, 10.52607193928646545 ) ) ;
#3104=CARTESIAN_POINT ( 'NONE',  ( -4.286401442266531525, -4.198423832313195270, 5.000000000000004441 ) ) ;
#3105=CARTESIAN_POINT ( 'NONE',  ( 0.2623718222035977821, 6.245654667075780431, 10.52627829713834018 ) ) ;
#3106=( NAMED_UNIT ( * ) SI_UNIT ( $, .STERADIAN. ) SOLID_ANGLE_UNIT ( ) );
#3107=CARTESIAN_POINT ( 'NONE',  ( 5.375913338529189289, -2.664979843780238777, 23.99571079637979665 ) ) ;
#3109=CARTESIAN_POINT ( 'NONE',  ( 1.354942164306246880E-13, -6.000000000000000888, 16.99999999999998579 ) ) ;
#3112=CARTESIAN_POINT ( 'NONE',  ( 3.254737477227979792, 5.337033878705218726, 31.87367328635992791 ) ) ;
#3117=ORIENTED_EDGE ( 'NONE', *, *, #5811, .F. ) ;
#3118=EDGE_CURVE ( 'NONE', #4626, #1119, #947, .T. ) ;
#3119=ORIENTED_EDGE ( 'NONE', *, *, #7586, .T. ) ;
#3120=CARTESIAN_POINT ( 'NONE',  ( 4.290130679986573270, -4.545972905167727340, 12.11560192892920718 ) ) ;
#3122=ORIENTED_EDGE ( 'NONE', *, *, #2307, .T. ) ;
#3129=DIRECTION ( 'NONE',  ( 0.9510565162951500895, 0.3090169943749582204, 0.000000000000000000 ) ) ;
#3140=DIRECTION ( 'NONE',  ( 0.8090169943749421222, 0.5877852522924802425, 0.000000000000000000 ) ) ;
#3145=FACE_OUTER_BOUND ( 'NONE', #14163, .T. ) ;
#3147=CARTESIAN_POINT ( 'NONE',  ( 4.195795028115047565, 4.289273350251304073, 4.495710796379801089 ) ) ;
#3148=( NAMED_UNIT ( * ) SI_UNIT ( $, .STERADIAN. ) SOLID_ANGLE_UNIT ( ) );
#3153=FACE_BOUND ( 'NONE', #12056, .T. ) ;
#3154=CARTESIAN_POINT ( 'NONE',  ( 0.000000000000000000, 6.250000000000000888, 25.49999999999999645 ) ) ;
#3157=CARTESIAN_POINT ( 'NONE',  ( 4.435347140100928343, -4.403429997944614982, 24.49999999999999289 ) ) ;
#3158=CARTESIAN_POINT ( 'NONE',  ( 5.935543223013846514, 0.8771126767607477781, 5.000000000000004441 ) ) ;
#3161=CARTESIAN_POINT ( 'NONE',  ( -5.783239563508382197, 1.602707436861265267, 23.52641404563304661 ) ) ;
#3163=CARTESIAN_POINT ( 'NONE',  ( 6.176542424588135738, 0.9554180641284293340, 24.63060690723497359 ) ) ;
#3168=CARTESIAN_POINT ( 'NONE',  ( -6.142908455506956855, 1.155755562475985654, 4.384822196241565884 ) ) ;
#3170=CARTESIAN_POINT ( 'NONE',  ( -3.735642931250987342, -4.696778275484508214, 30.02591947216899371 ) ) ;
#3178=CARTESIAN_POINT ( 'NONE',  ( -2.692693252389511294, -5.362085866495146291, 5.263826032055955118 ) ) ;
#3182=FILL_AREA_STYLE_COLOUR ( '', #3534 ) ;
#3183=CARTESIAN_POINT ( 'NONE',  ( 5.330189595673735958, -2.755293208590051890, 24.23617396794404044 ) ) ;
#3185=FACE_OUTER_BOUND ( 'NONE', #8944, .T. ) ;
#3189=CARTESIAN_POINT ( 'NONE',  ( -5.330004929009514392, -2.755647751839538806, 17.73760108194401752 ) ) ;
#3192=ORIENTED_EDGE ( 'NONE', *, *, #4450, .T. ) ;
#3193=ORIENTED_EDGE ( 'NONE', *, *, #10472, .F. ) ;
#3194=CARTESIAN_POINT ( 'NONE',  ( 2.817313151351127143, -5.579000502529464889, 11.63060690723496116 ) ) ;
#3196=B_SPLINE_CURVE_WITH_KNOTS ( 'NONE', 3,
 ( #2197, #3163, #3392, #9532, #2119, #9373, #4440, #12858, #2043, #14211, #13020, #5794, #15502, #4600, #11903, #8260, #1012, #7068 ),
 .UNSPECIFIED., .F., .F.,
 ( 4, 2, 2, 2, 2, 2, 2, 2, 4 ),
 ( 0.003131486019301973813, 0.003522824630466683121, 0.003914163241631392863, 0.004305501852796101737, 0.004696840463960811479, 0.005088179075125520354, 0.005479517686290230095, 0.005870856297454939837, 0.006262194908619648712 ),
 .UNSPECIFIED. ) ;
#3197=ORIENTED_EDGE ( 'NONE', *, *, #7064, .T. ) ;
#3200=CARTESIAN_POINT ( 'NONE',  ( 5.985119669071130133, 1.805077827356515341, 18.99991741810287493 ) ) ;
#3204=CARTESIAN_POINT ( 'NONE',  ( 5.375913338529122676, 2.664979843780374669, 18.50428920362019625 ) ) ;
#3209=CARTESIAN_POINT ( 'NONE',  ( 3.736691294293501109, -4.695920479336315623, 4.026414045633067040 ) ) ;
#3212=CARTESIAN_POINT ( 'NONE',  ( -5.935543223013861613, 0.8771126767606655106, 5.000000000000004441 ) ) ;
#3213=CARTESIAN_POINT ( 'NONE',  ( -0.9740807849836103927, 5.920620690450690837, 4.738501197006693921 ) ) ;
#3214=EDGE_CURVE ( 'NONE', #15454, #9028, #4514, .T. ) ;
#3217=AXIS2_PLACEMENT_3D ( 'NONE', #15248, #15406, #11580 ) ;
#3222=CARTESIAN_POINT ( 'NONE',  ( 5.317509234263932072, 2.779225709351047957, 5.000000000000004441 ) ) ;
#3226=CARTESIAN_POINT ( 'NONE',  ( 6.176542424588140179, -0.9554180641284089059, 17.99999999999998934 ) ) ;
#3227=CARTESIAN_POINT ( 'NONE',  ( -5.665308849928801571, 1.980336949702567129, 18.99992002356260912 ) ) ;
#3230=CARTESIAN_POINT ( 'NONE',  ( -3.158825713737709595, 5.393784879207039751, 25.29933148907577944 ) ) ;
#3232=ORIENTED_EDGE ( 'NONE', *, *, #13510, .T. ) ;
#3233=CARTESIAN_POINT ( 'NONE',  ( -5.570820891630761551, 2.833901239560411955, 18.26236973443873168 ) ) ;
#3236=CARTESIAN_POINT ( 'NONE',  ( -5.131373506000769247, 7.062729720843990755, 11.49999999999998224 ) ) ;
#3240=CARTESIAN_POINT ( 'NONE',  ( -5.915653884842702936, -1.003805156977440438, 5.504397606442129387 ) ) ;
#3242=CYLINDRICAL_SURFACE ( 'NONE', #1896, 6.000000000000000888 ) ;
#3244=CARTESIAN_POINT ( 'NONE',  ( 0.5031281619707989039, 5.980084330432664963, 30.12602272744524967 ) ) ;
#3245=EDGE_LOOP ( 'NONE', ( #7236, #2162, #2129, #10520 ) ) ;
#3247=LINE ( 'NONE', #5648, #4274 ) ;
#3248=AXIS2_PLACEMENT_3D ( 'NONE', #8997, #6375, #9148 ) ;
#3249=ORIENTED_EDGE ( 'NONE', *, *, #6004, .F. ) ;
#3250=CARTESIAN_POINT ( 'NONE',  ( -2.782713018890565770, -5.315928322779200244, 4.495602393557862619 ) ) ;
#3252=CARTESIAN_POINT ( 'NONE',  ( 5.843075991566594851, 1.368655265451002911, 17.12635295315575590 ) ) ;
#3255=LINE ( 'NONE', #1749, #14025 ) ;
#3257=CARTESIAN_POINT ( 'NONE',  ( -5.984759433607005796, -1.806271833852304054, 3.999917806784440977 ) ) ;
#3259=LINE ( 'NONE', #14305, #9529 ) ;
#3260=CARTESIAN_POINT ( 'NONE',  ( 3.883716939929066303, 4.898343590941186321, 31.97359571723301741 ) ) ;
#3261=CARTESIAN_POINT ( 'NONE',  ( -0.5042987395406310913, -5.979983180450088476, 18.87329304179975864 ) ) ;
#3262=EDGE_CURVE ( 'NONE', #14829, #11779, #15713, .T. ) ;
#3263=ORIENTED_EDGE ( 'NONE', *, *, #8275, .F. ) ;
#3264=B_SPLINE_CURVE_WITH_KNOTS ( 'NONE', 3,
 ( #4108, #600, #14853, #8977, #2917, #11497, #6355, #1710, #5152, #290, #8815, #13644, #11806, #671, #994, #12763, #13079, #3222 ),
 .UNSPECIFIED., .F., .F.,
 ( 4, 2, 2, 2, 2, 2, 2, 2, 4 ),
 ( 0.003131918686235971722, 0.003523310662250261557, 0.003914702638264551393, 0.004306094614278841229, 0.004697486590293131065, 0.005088878566307420900, 0.005480270542321711603, 0.005871662518336001439, 0.006263054494350291275 ),
 .UNSPECIFIED. ) ;
#3265=ORIENTED_EDGE ( 'NONE', *, *, #78, .T. ) ;
#3268=VERTEX_POINT ( 'NONE', #4437 ) ;
#3270=CARTESIAN_POINT ( 'NONE',  ( 2.817313151351066747, -5.579000502529495975, 18.13060690723497004 ) ) ;
#3271=DIRECTION ( 'NONE',  ( 0.000000000000000000, 1.000000000000000000, 0.000000000000000000 ) ) ;
#3272=EDGE_LOOP ( 'NONE', ( #5512, #7097, #2471, #8178 ) ) ;
#3274=ADVANCED_FACE ( 'NONE', ( #6914 ), #6989, .F. ) ;
#3275=CARTESIAN_POINT ( 'NONE',  ( -5.317509234263918749, -2.779225709351067053, 31.13064961348856130 ) ) ;
#3276=CARTESIAN_POINT ( 'NONE',  ( -4.152999119457922106, -4.671604476854401611, 4.199734849823242300 ) ) ;
#3279=CARTESIAN_POINT ( 'NONE',  ( 5.409423237179044719, 2.597448116730965317, 18.61561732698605454 ) ) ;
#3282=STYLED_ITEM ( 'NONE', ( #1539 ), #15531 ) ;
#3284=CARTESIAN_POINT ( 'NONE',  ( 4.416779112813715713, -4.422345839825735148, 4.737747182782874766 ) ) ;
#3286=DIRECTION ( 'NONE',  ( -0.5877852522924685852, -0.8090169943749507819, 0.000000000000000000 ) ) ;
#3288=CARTESIAN_POINT ( 'NONE',  ( -5.317509234263873452, 2.779225709351156315, 24.49999999999999289 ) ) ;
#3290=CARTESIAN_POINT ( 'NONE',  ( -1.000049271338417256, 6.169473353325564347, 11.36969612704547750 ) ) ;
#3293=CARTESIAN_POINT ( 'NONE',  ( -0.8736516769106945635, 5.936271176698233454, 4.496067715786786323 ) ) ;
#3294=ORIENTED_EDGE ( 'NONE', *, *, #1670, .T. ) ;
#3295=CARTESIAN_POINT ( 'NONE',  ( 3.158296126777773605, 5.394094919772124186, 10.70112161576660270 ) ) ;
#3298=CARTESIAN_POINT ( 'NONE',  ( -2.817313151351250156, 5.579000502529401828, 11.63237410716304865 ) ) ;
#3301=DIRECTION ( 'NONE',  ( -0.9510565162951544194, 0.3090169943749447312, 0.000000000000000000 ) ) ;
#3305=CARTESIAN_POINT ( 'NONE',  ( -5.558508435838126260, -2.857531096719055252, 17.99999999999998934 ) ) ;
#3307=VECTOR ( 'NONE', #9068, 1000.000000000000000 ) ;
#3308=CARTESIAN_POINT ( 'NONE',  ( 2.817313151351047207, 5.579000502529503080, 11.49999999999998224 ) ) ;
#3312=CARTESIAN_POINT ( 'NONE',  ( -3.255128505894475666, 5.336774832660618806, 25.37380055247395916 ) ) ;
#3313=EDGE_CURVE ( 'NONE', #12601, #8963, #511, .T. ) ;
#3314=DIRECTION ( 'NONE',  ( -0.5877852522924685852, -0.8090169943749508930, 0.000000000000000000 ) ) ;
#3316=FACE_OUTER_BOUND ( 'NONE', #14983, .T. ) ;
#3317=ORIENTED_EDGE ( 'NONE', *, *, #15341, .F. ) ;
#3318=CARTESIAN_POINT ( 'NONE',  ( -5.903119516422456137, 1.077859910107602515, 23.88480617551148555 ) ) ;
#3320=FACE_OUTER_BOUND ( 'NONE', #6675, .T. ) ;
#3321=CARTESIAN_POINT ( 'NONE',  ( -4.435347140101024266, -4.403429997944519947, 31.00000000000000000 ) ) ;
#3323=CARTESIAN_POINT ( 'NONE',  ( 5.558508435838221295, 2.857531096718871844, 11.49999999999998224 ) ) ;
#3326=ORIENTED_EDGE ( 'NONE', *, *, #12016, .F. ) ;
#3328=CARTESIAN_POINT ( 'NONE',  ( 3.106366801611981643, 5.134708448381295476, 30.12696220972948780 ) ) ;
#3330=CARTESIAN_POINT ( 'NONE',  ( -3.420659742068303810, -4.931142898501790661, 4.000049463537775907 ) ) ;
#3332=CARTESIAN_POINT ( 'NONE',  ( 5.866817325727523347, 1.260653813891904784, 17.19977782616120621 ) ) ;
#3334=CARTESIAN_POINT ( 'NONE',  ( 4.005998022989861518, 4.467726698309353317, 18.79931806258173665 ) ) ;
#3338=CARTESIAN_POINT ( 'NONE',  ( 4.286401442266591921, -4.198423832313132209, 5.000000000000004441 ) ) ;
#3340=CARTESIAN_POINT ( 'NONE',  ( -0.8738118504724315949, -5.936246475285051005, 18.50357242174242600 ) ) ;
#3341=EDGE_LOOP ( 'NONE', ( #8251, #9877 ) ) ;
#3342=ORIENTED_EDGE ( 'NONE', *, *, #7064, .F. ) ;
#3344=VECTOR ( 'NONE', #4978, 1000.000000000000000 ) ;
#3345=CARTESIAN_POINT ( 'NONE',  ( 3.458623254138704084, 5.207221900902825773, 30.02622717124732077 ) ) ;
#3346=CARTESIAN_POINT ( 'NONE',  ( -4.286401442266642547, 4.198423832313083359, 11.63064961348853288 ) ) ;
#3349=EDGE_CURVE ( 'NONE', #9247, #8051, #2225, .T. ) ;
#3351=CARTESIAN_POINT ( 'NONE',  ( 0.9999502950802097168, -5.916088184763882651, 5.131081491900111757 ) ) ;
#3352=CARTESIAN_POINT ( 'NONE',  ( -3.458467055437195459, -5.207305717053890781, 4.026404282766992360 ) ) ;
#3355=CARTESIAN_POINT ( 'NONE',  ( 6.172614129015236983, -0.9817721000788701691, 4.737630265561252330 ) ) ;
#3357=VECTOR ( 'NONE', #3410, 1000.000000000000114 ) ;
#3364=VERTEX_POINT ( 'NONE', #4902 ) ;
#3366=EDGE_CURVE ( 'NONE', #9045, #3737, #4533, .T. ) ;
#3367=CARTESIAN_POINT ( 'NONE',  ( -3.779082820360757378, -4.979770177899202288, 23.49995093123465750 ) ) ;
#3371=CARTESIAN_POINT ( 'NONE',  ( -5.408775798201138407, 2.598833957129706551, 17.38602261056917087 ) ) ;
#3372=CARTESIAN_POINT ( 'NONE',  ( 4.142173849413612885, 4.341773579105533187, 25.11519382448850379 ) ) ;
#3373=CARTESIAN_POINT ( 'NONE',  ( 2.031800923367348393E-13, -6.250000000000000888, 23.49999999999999289 ) ) ;
#3375=CARTESIAN_POINT ( 'NONE',  ( -6.142844459177198679, -1.156093792145410193, 23.88439807107078039 ) ) ;
#3380=CARTESIAN_POINT ( 'NONE',  ( -5.648559266344464369, -2.676764518776065138, 18.61396179408071205 ) ) ;
#3386=CYLINDRICAL_SURFACE ( 'NONE', #479, 1.000000000000000666 ) ;
#3387=CARTESIAN_POINT ( 'NONE',  ( -6.176542424588101099, 0.9554180641286806885, 18.13234125634167526 ) ) ;
#3388=ORIENTED_EDGE ( 'NONE', *, *, #6253, .F. ) ;
#3392=CARTESIAN_POINT ( 'NONE',  ( 6.172614129015254747, 0.9817721000787504870, 24.76236973443873524 ) ) ;
#3399=CARTESIAN_POINT ( 'NONE',  ( 5.940390500375535510, 6.474944468551633747, 31.00000000000000000 ) ) ;
#3400=VERTEX_POINT ( 'NONE', #1829 ) ;
#3403=CARTESIAN_POINT ( 'NONE',  ( 4.286401442266448036, -4.198423832313277870, 24.49999999999999289 ) ) ;
#3405=DIRECTION ( 'NONE',  ( -0.9510565162951545304, 0.3090169943749447867, 0.000000000000000000 ) ) ;
#3408=CARTESIAN_POINT ( 'NONE',  ( 4.290130679986468465, 4.545972905167828593, 17.38439807107078749 ) ) ;
#3410=DIRECTION ( 'NONE',  ( 0.9510565162951499785, 0.3090169943749582204, 0.000000000000000000 ) ) ;
#3416=DIRECTION ( 'NONE',  ( -0.5877852522924685852, -0.8090169943749508930, 0.000000000000000000 ) ) ;
#3418=ORIENTED_EDGE ( 'NONE', *, *, #3214, .T. ) ;
#3421=CARTESIAN_POINT ( 'NONE',  ( 3.882809187878927926, 4.899079348630055009, 30.02599901976670438 ) ) ;
#3422=DIRECTION ( 'NONE',  ( 0.000000000000000000, 0.000000000000000000, 1.000000000000000000 ) ) ;
#3425=CARTESIAN_POINT ( 'NONE',  ( 0.5044069930203403107, -5.979990686694992341, 5.873357432279041390 ) ) ;
#3429=B_SPLINE_CURVE_WITH_KNOTS ( 'NONE', 3,
 ( #6690, #624, #14220, #9382, #2128, #15196, #3328, #14295, #6927, #785, #11759, #938, #862, #15354, #5729, #10420, #8115, #11526 ),
 .UNSPECIFIED., .F., .F.,
 ( 4, 2, 2, 2, 2, 2, 2, 2, 4 ),
 ( 0.003131918686235979528, 0.003523310662250269364, 0.003914702638264559199, 0.004306094614278849035, 0.004697486590293139738, 0.005088878566307429574, 0.005480270542321720277, 0.005871662518336010980, 0.006263054494350301683 ),
 .UNSPECIFIED. ) ;
#3431=CARTESIAN_POINT ( 'NONE',  ( 5.859155363331391975, -2.178872204144952196, 4.025999019766705267 ) ) ;
#3436=CARTESIAN_POINT ( 'NONE',  ( 5.903472034603470142, 2.056448723545269974, 6.000082193215566129 ) ) ;
#3438=ORIENTED_EDGE ( 'NONE', *, *, #158, .F. ) ;
#3439=AXIS2_PLACEMENT_3D ( 'NONE', #14275, #8253, #6909 ) ;
#3440=CARTESIAN_POINT ( 'NONE',  ( -5.558508435838219519, 2.857531096718872732, 31.00000000000000000 ) ) ;
#3441=ORIENTED_EDGE ( 'NONE', *, *, #2600, .T. ) ;
#3443=DIRECTION ( 'NONE',  ( 0.000000000000000000, 1.000000000000000000, 0.000000000000000000 ) ) ;
#3444=CARTESIAN_POINT ( 'NONE',  ( 2.692143549875356534, -5.362363179736500562, 17.73805675996853637 ) ) ;
#3445=CARTESIAN_POINT ( 'NONE',  ( -2.782769401326306902, -5.315896561274780829, 25.00428920362020335 ) ) ;
#3446=ORIENTED_EDGE ( 'NONE', *, *, #3072, .F. ) ;
#3447=CARTESIAN_POINT ( 'NONE',  ( -6.105925084677685355, -1.337450587213164566, 31.79933148907577234 ) ) ;
#3450=LINE ( 'NONE', #1298, #3344 ) ;
#3454=CARTESIAN_POINT ( 'NONE',  ( -5.769755079862221692, -2.405651898699208147, 23.62694108445698049 ) ) ;
#3460=CARTESIAN_POINT ( 'NONE',  ( 5.649200442566231217, -2.675373855293995184, 17.38439807107078394 ) ) ;
#3463=VERTEX_POINT ( 'NONE', #14975 ) ;
#3465=CARTESIAN_POINT ( 'NONE',  ( 0.9999502950802738876, -5.916088184763872881, 11.63108149190010288 ) ) ;
#3468=CARTESIAN_POINT ( 'NONE',  ( 3.158296126777893953, -5.394094919772051355, 31.79887838423339019 ) ) ;
#3469=CARTESIAN_POINT ( 'NONE',  ( 2.082642335314403343E-14, -6.250000000000000888, 32.00000000000000000 ) ) ;
#3475=DIRECTION ( 'NONE',  ( 0.000000000000000000, 0.000000000000000000, 1.000000000000000000 ) ) ;
#3485=CARTESIAN_POINT ( 'NONE',  ( -2.841519077896137002, -5.566940434250017056, 11.76379616840804410 ) ) ;
#3488=CARTESIAN_POINT ( 'NONE',  ( -3.735642931250969134, -4.696778275484520648, 4.025919472168996371 ) ) ;
#3490=CARTESIAN_POINT ( 'NONE',  ( 5.620786884546293827, -2.102685372472877567, 5.973585954366940065 ) ) ;
#3492=FACE_OUTER_BOUND ( 'NONE', #11024, .T. ) ;
#3494=CARTESIAN_POINT ( 'NONE',  ( 2.848727059635998149, -5.281416301279876713, 18.61442521571936837 ) ) ;
#3496=CARTESIAN_POINT ( 'NONE',  ( -5.570820891630784644, -2.833901239560364438, 4.737630265561251441 ) ) ;
#3500=CARTESIAN_POINT ( 'NONE',  ( -5.859221468178978043, 2.178708437343151783, 10.52591457665827335 ) ) ;
#3503=ORIENTED_EDGE ( 'NONE', *, *, #4548, .T. ) ;
#3507=CARTESIAN_POINT ( 'NONE',  ( -3.922672396097124814, 4.541739265057643138, 12.37364704684421213 ) ) ;
#3508=EDGE_CURVE ( 'NONE', #13977, #4648, #14592, .T. ) ;
#3510=VECTOR ( 'NONE', #7057, 1000.000000000000114 ) ;
#3512=CARTESIAN_POINT ( 'NONE',  ( 1.000049560716553154, -5.916071405810146899, 4.869677990115314437 ) ) ;
#3513=CARTESIAN_POINT ( 'NONE',  ( 5.649200442566148617, 2.675373855294168823, 31.61560192892921251 ) ) ;
#3516=CARTESIAN_POINT ( 'NONE',  ( -5.317509234263959605, 2.779225709350992002, 31.00000000000000000 ) ) ;
#3519=CARTESIAN_POINT ( 'NONE',  ( 3.779681992289875669, -4.979315417303840974, 4.000049210157071045 ) ) ;
#3521=CARTESIAN_POINT ( 'NONE',  ( 6.106056299406729337, 1.336851112280767140, 5.798878384233397298 ) ) ;
#3522=ORIENTED_EDGE ( 'NONE', *, *, #8143, .F. ) ;
#3524=B_SPLINE_CURVE_WITH_KNOTS ( 'NONE', 3,
 ( #4826, #7215, #9438, #1077, #15644, #9518, #5783, #3620, #8326, #9682, #7294, #13165, #2264, #5938, #11971, #6978, #7135, #14439 ),
 .UNSPECIFIED., .F., .F.,
 ( 4, 2, 2, 2, 2, 2, 2, 2, 4 ),
 ( 0.000000000000000000, 0.0003914898357794968447, 0.0007829796715589936893, 0.001174469507338490480, 0.001565959343117988463, 0.001957449178897486229, 0.002348939014676983995, 0.002740428850456482195, 0.003131918686235979528 ),
 .UNSPECIFIED. ) ;
#3526=DIRECTION ( 'NONE',  ( -0.5877852522924685852, -0.8090169943749508930, 0.000000000000000000 ) ) ;
#3527=ORIENTED_EDGE ( 'NONE', *, *, #12992, .F. ) ;
#3528=EDGE_LOOP ( 'NONE', ( #12583, #5924 ) ) ;
#3529=CARTESIAN_POINT ( 'NONE',  ( -6.155854678529470547, -1.081900940642134046, 30.49574050496988775 ) ) ;
#3531=CARTESIAN_POINT ( 'NONE',  ( -2.668367453516813370, -5.373994336898042512, 24.63236078583910427 ) ) ;
#3532=CARTESIAN_POINT ( 'NONE',  ( 4.286401442266544848, -4.198423832313181059, 11.49999999999998224 ) ) ;
#3533=CARTESIAN_POINT ( 'NONE',  ( 2.782468714962200274, 5.316055268221527186, 25.00389795015983196 ) ) ;
#3534=COLOUR_RGB ( '', 0.09019608, 0.27058824, 0.51372549) ;
#3535=CARTESIAN_POINT ( 'NONE',  ( 5.935543223013862502, -0.8771126767606430841, 31.00000000000000000 ) ) ;
#3536=CARTESIAN_POINT ( 'NONE',  ( -4.152999119458038457, 4.671604476854301247, 12.30026515017674527 ) ) ;
#3537=CARTESIAN_POINT ( 'NONE',  ( 5.843075991566567318, 1.368655265451115932, 30.12635295315577011 ) ) ;
#3538=CARTESIAN_POINT ( 'NONE',  ( 0.2622916576878590589, -5.995491482261820160, 25.47384942646813499 ) ) ;
#3543=CARTESIAN_POINT ( 'NONE',  ( 5.531757352715570342, 2.326874507723404761, 31.87380682714711355 ) ) ;
#3544=VECTOR ( 'NONE', #7320, 1000.000000000000000 ) ;
#3545=ORIENTED_EDGE ( 'NONE', *, *, #2829, .T. ) ;
#3546=CARTESIAN_POINT ( 'NONE',  ( -4.142620314836359618, 4.341347824677524336, 4.385574784280628080 ) ) ;
#3547=DIRECTION ( 'NONE',  ( 0.000000000000000000, 0.000000000000000000, 1.000000000000000000 ) ) ;
#3548=CARTESIAN_POINT ( 'NONE',  ( 5.903230462362981434, 1.077253041748728490, 25.11442521571936481 ) ) ;
#3550=CARTESIAN_POINT ( 'NONE',  ( 4.069800786343840571, -4.744882212776791341, 31.87381964045071214 ) ) ;
#3551=CARTESIAN_POINT ( 'NONE',  ( 7.490007020835692586, -2.433650805992223720, 31.00000000000000000 ) ) ;
#3552=CARTESIAN_POINT ( 'NONE',  ( -3.107583187530477353, 5.133966411712655109, 10.62619317285287934 ) ) ;
#3557=CARTESIAN_POINT ( 'NONE',  ( -5.858813228503651160, 2.179803269293273615, 12.47377282875266324 ) ) ;
#3559=CARTESIAN_POINT ( 'NONE',  ( -4.416837305303504380, 4.422286678979004293, 5.261902130840119263 ) ) ;
#3567=CARTESIAN_POINT ( 'NONE',  ( -4.344762547369706240, -4.493114738039222011, 12.00308643866043568 ) ) ;
#3568=ORIENTED_EDGE ( 'NONE', *, *, #3313, .F. ) ;
#3570=EDGE_CURVE ( 'NONE', #4648, #13977, #15179, .T. ) ;
#3572=CARTESIAN_POINT ( 'NONE',  ( 0.8730628416138148662, 6.188929913094951551, 10.99504929893119609 ) ) ;
#3576=CARTESIAN_POINT ( 'NONE',  ( 2.082642335314403343E-14, -6.000000000000000888, 32.00000000000000000 ) ) ;
#3583=EDGE_CURVE ( 'NONE', #7332, #7142, #13820, .T. ) ;
#3586=CARTESIAN_POINT ( 'NONE',  ( -4.005361199355045088, 4.468319061418729810, 12.30022217383878846 ) ) ;
#3590=CARTESIAN_POINT ( 'NONE',  ( 5.770288754215095572, 2.404361317820031374, 31.87381964045071925 ) ) ;
#3598=CARTESIAN_POINT ( 'NONE',  ( 2.817313151351047207, 5.579000502529503080, 11.49999999999998224 ) ) ;
#3603=VERTEX_POINT ( 'NONE', #7010 ) ;
#3605=CARTESIAN_POINT ( 'NONE',  ( -5.858813228503603199, 2.179803269293398404, 25.47377282875267923 ) ) ;
#3606=CARTESIAN_POINT ( 'NONE',  ( -4.291255145204137200, -4.544933371694618529, 23.88603820591928084 ) ) ;
#3607=CARTESIAN_POINT ( 'NONE',  ( 6.780834061396424457E-14, 6.250000000000000888, 10.49999999999998224 ) ) ;
#3608=CARTESIAN_POINT ( 'NONE',  ( -6.155854678529483870, 1.081900940642043452, 31.50425949503011225 ) ) ;
#3609=CARTESIAN_POINT ( 'NONE',  ( 0.9999196734183355417, 5.916093360767503917, 11.36725955955069622 ) ) ;
#3613=CARTESIAN_POINT ( 'NONE',  ( -2.841041022017453344, 5.567186575787228087, 11.76225281721714566 ) ) ;
#3614=CARTESIAN_POINT ( 'NONE',  ( 5.375886393124347684, 2.665038680141360139, 30.49560239355787417 ) ) ;
#3615=CARTESIAN_POINT ( 'NONE',  ( 5.935543223013849179, 0.8771126767607271280, 31.00000000000000000 ) ) ;
#3620=CARTESIAN_POINT ( 'NONE',  ( 3.736691294293418508, 4.695920479336378683, 31.97358595436693918 ) ) ;
#3621=CARTESIAN_POINT ( 'NONE',  ( 5.867109477881222723, 1.259218163101011534, 31.79888242247940511 ) ) ;
#3624=CARTESIAN_POINT ( 'NONE',  ( -2.668367453516709009, 5.373994336898094915, 4.867639214160893957 ) ) ;
#3625=CARTESIAN_POINT ( 'NONE',  ( -0.2638277032948134759, -5.995407492418042494, 12.47332055281516716 ) ) ;
#3626=CARTESIAN_POINT ( 'NONE',  ( 5.935543223013877601, 0.8771126767605438301, 24.63061695532138629 ) ) ;
#3628=CARTESIAN_POINT ( 'NONE',  ( 3.566234721238137784, -5.134387337253762063, 31.99991741810289625 ) ) ;
#3630=CARTESIAN_POINT ( 'NONE',  ( 4.435347140100866170, 4.403429997944679819, 24.49999999999999289 ) ) ;
#3632=CARTESIAN_POINT ( 'NONE',  ( -4.344762547369864336, 4.493114738039070133, 23.99691356133952169 ) ) ;
#3633=AXIS2_PLACEMENT_3D ( 'NONE', #15287, #12965, #7093 ) ;
#3636=CARTESIAN_POINT ( 'NONE',  ( -4.344502777243558711, 4.493369211529237184, 5.503892131249680908 ) ) ;
#3639=CARTESIAN_POINT ( 'NONE',  ( 5.984377695197246716, 1.807429553002209976, 16.99995093123465750 ) ) ;
#3640=ORIENTED_EDGE ( 'NONE', *, *, #5939, .F. ) ;
#3643=CARTESIAN_POINT ( 'NONE',  ( -2.817313151351169775, -5.579000502529442684, 11.49999999999998224 ) ) ;
#3644=VERTEX_POINT ( 'NONE', #15601 ) ;
#3647=CARTESIAN_POINT ( 'NONE',  ( 0.9999505860955437697, -6.169489349035773174, 24.63105903165811839 ) ) ;
#3648=CARTESIAN_POINT ( 'NONE',  ( 5.858736126997158955, -2.179962889276996663, 31.97359571723301741 ) ) ;
#3654=CARTESIAN_POINT ( 'NONE',  ( 5.867109477881251145, -1.259218163100882970, 10.70111757752057002 ) ) ;
#3655=CARTESIAN_POINT ( 'NONE',  ( -3.781065399486017053, 4.978303713186439161, 30.00008258189711441 ) ) ;
#3656=CARTESIAN_POINT ( 'NONE',  ( -5.903843691985231956, 2.055287728870642816, 10.49995093123465395 ) ) ;
#3657=CARTESIAN_POINT ( 'NONE',  ( -5.408775798201197027, 2.598833957129591532, 30.38602261056917442 ) ) ;
#3659=ORIENTED_EDGE ( 'NONE', *, *, #9996, .F. ) ;
#3661=ADVANCED_FACE ( 'NONE', ( #3185 ), #6859, .F. ) ;
#3663=ORIENTED_EDGE ( 'NONE', *, *, #9140, .T. ) ;
#3664=B_SPLINE_CURVE_WITH_KNOTS ( 'NONE', 3,
 ( #11770, #7172, #14394, #8206, #7013, #14481, #10583, #4621, #13042, #9556, #12010, #8285, #15444, #8450, #1114, #797, #1032, #4784 ),
 .UNSPECIFIED., .F., .F.,
 ( 4, 2, 2, 2, 2, 2, 2, 2, 4 ),
 ( 0.000000000000000000, 0.0003914362731607599595, 0.0007828725463215199191, 0.001174308819482279987, 0.001565745092643039838, 0.001957181365803799689, 0.002348617638964559974, 0.002740053912125319825, 0.003131490185286079676 ),
 .UNSPECIFIED. ) ;
#3665=CARTESIAN_POINT ( 'NONE',  ( -2.668367453516892418, 5.373994336898001656, 24.49999999999999289 ) ) ;
#3666=VERTEX_POINT ( 'NONE', #6058 ) ;
#3668=CARTESIAN_POINT ( 'NONE',  ( -6.176542424588095770, -0.9554180641287001174, 11.49999999999998224 ) ) ;
#3674=CARTESIAN_POINT ( 'NONE',  ( 3.011899281037468068, 5.190111395030246655, 5.800222173838807116 ) ) ;
#3679=EDGE_LOOP ( 'NONE', ( #15291, #14330, #9380, #3082 ) ) ;
#3682=ORIENTED_EDGE ( 'NONE', *, *, #6146, .T. ) ;
#3687=CARTESIAN_POINT ( 'NONE',  ( 3.735808404765003754, -4.696639218303121588, 12.47398020122237661 ) ) ;
#3689=CARTESIAN_POINT ( 'NONE',  ( -4.196288036172415303, -4.288789315524868861, 12.00312048902375039 ) ) ;
#3690=CARTESIAN_POINT ( 'NONE',  ( -3.459447313391887047, 5.206669755180961090, 10.52599901976669194 ) ) ;
#3692=CARTESIAN_POINT ( 'NONE',  ( 6.768587589771821120E-14, 6.000000000000000888, 12.49999999999998401 ) ) ;
#3700=EDGE_LOOP ( 'NONE', ( #7036, #3819, #7579, #12667 ) ) ;
#3701=CARTESIAN_POINT ( 'NONE',  ( -5.330004929009583670, 2.755647751839406023, 11.76239891805594695 ) ) ;
#3702=CARTESIAN_POINT ( 'NONE',  ( 6.780834053290958173E-14, -6.000000000000000888, 10.49999999999998224 ) ) ;
#3704=CARTESIAN_POINT ( 'NONE',  ( 5.935543223013889147, -0.8771126767604601193, 24.49999999999999289 ) ) ;
#3707=FACE_OUTER_BOUND ( 'NONE', #8873, .T. ) ;
#3711=CARTESIAN_POINT ( 'NONE',  ( -0.1323408341374683050, -6.250000000000002665, 32.00000000000000711 ) ) ;
#3713=FACE_BOUND ( 'NONE', #10752, .T. ) ;
#3716=CARTESIAN_POINT ( 'NONE',  ( 5.725930890718397670, -2.506952462183888120, 25.29933148907577234 ) ) ;
#3725=CARTESIAN_POINT ( 'NONE',  ( 5.866817325727508248, -1.260653813891976061, 5.800222173838807116 ) ) ;
#3726=DIRECTION ( 'NONE',  ( 0.000000000000000000, 1.000000000000000000, 0.000000000000000000 ) ) ;
#3729=CARTESIAN_POINT ( 'NONE',  ( 5.486982057989271411, -2.429327048029698233, 25.29931806258174376 ) ) ;
#3731=B_SPLINE_CURVE_WITH_KNOTS ( 'NONE', 3,
 ( #7377, #8422, #2358, #8733, #4836, #1243, #5070, #13491, #13335, #11030, #9922, #7302, #1162, #7226, #10793, #11868, #6031, #3630 ),
 .UNSPECIFIED., .F., .F.,
 ( 4, 2, 2, 2, 2, 2, 2, 2, 4 ),
 ( 0.003131486019301992895, 0.003522824630466699601, 0.003914163241631405873, 0.004305501852796113013, 0.004696840463960820153, 0.005088179075125526425, 0.005479517686290233565, 0.005870856297454941572, 0.006262194908619648712 ),
 .UNSPECIFIED. ) ;
#3733=CARTESIAN_POINT ( 'NONE',  ( 5.843075991566589522, -1.368655265451022451, 31.87364704684421923 ) ) ;
#3734=CARTESIAN_POINT ( 'NONE',  ( -5.621278735166232110, 2.101423246382466026, 10.52591947216897594 ) ) ;
#3736=CARTESIAN_POINT ( 'NONE',  ( -5.375763363753467416, 2.665284979407501087, 30.49610204984016448 ) ) ;
#3737=VERTEX_POINT ( 'NONE', #8530 ) ;
#3738=ORIENTED_EDGE ( 'NONE', *, *, #5282, .T. ) ;
#3740=VERTEX_POINT ( 'NONE', #9794 ) ;
#3742=EDGE_LOOP ( 'NONE', ( #9098, #11954, #4252, #9782 ) ) ;
#3745=ORIENTED_EDGE ( 'NONE', *, *, #2981, .T. ) ;
#3746=CARTESIAN_POINT ( 'NONE',  ( 5.558508435838200867, 2.857531096718914920, 31.13234125634169658 ) ) ;
#3749=EDGE_CURVE ( 'NONE', #15704, #1426, #15680, .T. ) ;
#3752=CARTESIAN_POINT ( 'NONE',  ( 2.848235266351006434, 5.281699484015658363, 5.613977389430844234 ) ) ;
#3754=DIRECTION ( 'NONE',  ( -0.5877852522924685852, -0.8090169943749508930, 0.000000000000000000 ) ) ;
#3758=VECTOR ( 'NONE', #13065, 1000.000000000000000 ) ;
#3760=CARTESIAN_POINT ( 'NONE',  ( 5.903230462362963671, -1.077253041748834406, 30.38557478428061742 ) ) ;
#3763=CARTESIAN_POINT ( 'NONE',  ( -0.9737778612005471013, -5.920671847850519143, 4.737363758846508510 ) ) ;
#3764=CARTESIAN_POINT ( 'NONE',  ( -6.021167129161054454, -1.680051667990301922, 31.97359571723301741 ) ) ;
#3768=CARTESIAN_POINT ( 'NONE',  ( -5.570820891630826388, 2.833901239560284502, 5.262369734438755664 ) ) ;
#3776=ORIENTED_EDGE ( 'NONE', *, *, #12447, .T. ) ;
#3777=CARTESIAN_POINT ( 'NONE',  ( -4.143041610105339778, 4.340967609747004019, 5.613977389430842457 ) ) ;
#3785=CARTESIAN_POINT ( 'NONE',  ( -4.435347140101089103, 4.403429997944455110, 31.00000000000000000 ) ) ;
#3794=CARTESIAN_POINT ( 'NONE',  ( 0.5042987395407951823, 5.979983180450074265, 31.87329304179976219 ) ) ;
#3795=ORIENTED_EDGE ( 'NONE', *, *, #9036, .F. ) ;
#3802=B_SPLINE_CURVE_WITH_KNOTS ( 'NONE', 3,
 ( #5400, #13742, #2769, #452, #7776, #5324, #6444, #4116, #6364, #4032, #2609, #12623, #14862, #1720, #5161, #11277, #13815, #8987 ),
 .UNSPECIFIED., .F., .F.,
 ( 4, 2, 2, 2, 2, 2, 2, 2, 4 ),
 ( 0.000000000000000000, 0.0003914898357794965194, 0.0007829796715589930388, 0.001174469507338489612, 0.001565959343117986078, 0.001957449178897482760, 0.002348939014676979225, 0.002740428850456475690, 0.003131918686235972155 ),
 .UNSPECIFIED. ) ;
#3804=STYLED_ITEM ( 'NONE', ( #10469 ), #4039 ) ;
#3811=CARTESIAN_POINT ( 'NONE',  ( -0.2638277032948710410, -5.995407492418040718, 31.97332055281518848 ) ) ;
#3812=CARTESIAN_POINT ( 'NONE',  ( 5.782895619916176955, -1.604017620858013915, 31.97408052783100985 ) ) ;
#3813=CARTESIAN_POINT ( 'NONE',  ( -0.8730628416135957082, -6.188929913094981750, 17.49504929893117477 ) ) ;
#3815=LINE ( 'NONE', #13517, #14913 ) ;
#3816=CARTESIAN_POINT ( 'NONE',  ( 3.633127580202104134, 4.776802569231184847, 23.49992038825523011 ) ) ;
#3819=ORIENTED_EDGE ( 'NONE', *, *, #10559, .F. ) ;
#3822=ORIENTED_EDGE ( 'NONE', *, *, #2508, .F. ) ;
#3824=CARTESIAN_POINT ( 'NONE',  ( -6.081464507797611496, -1.446657058464287715, 12.37380055247394672 ) ) ;
#3825=DIRECTION ( 'NONE',  ( 1.000000000000000000, 0.000000000000000000, 0.000000000000000000 ) ) ;
#3828=CYLINDRICAL_SURFACE ( 'NONE', #13538, 1.000000000000000888 ) ;
#3830=CARTESIAN_POINT ( 'NONE',  ( 4.286401442266578599, -4.198423832313147308, 31.13236078583911137 ) ) ;
#3832=CARTESIAN_POINT ( 'NONE',  ( -5.615973259022341679, 2.743340227996126757, 30.49610786875030044 ) ) ;
#3838=CARTESIAN_POINT ( 'NONE',  ( 5.843318061569056532, -1.367618216965589717, 30.12696220972948424 ) ) ;
#3839=CARTESIAN_POINT ( 'NONE',  ( 3.566234721238087158, 5.134387337253796701, 4.000082581897114409 ) ) ;
#3840=CARTESIAN_POINT ( 'NONE',  ( 7.347881158177969135E-16, 6.250000000000000888, 4.000000000000004441 ) ) ;
#3841=CARTESIAN_POINT ( 'NONE',  ( -3.420311045507865355, -4.931422832349278806, 19.00007961174475213 ) ) ;
#3842=CARTESIAN_POINT ( 'NONE',  ( 0.6144377077730618364, 5.969178481556058458, 10.70033966857734775 ) ) ;
#3844=DIRECTION ( 'NONE',  ( 0.8090169943749506709, -0.5877852522924686962, 0.000000000000000000 ) ) ;
#3845=CARTESIAN_POINT ( 'NONE',  ( -4.435347140101121965, 4.403429997944421359, 11.36939309276498911 ) ) ;
#3846=CARTESIAN_POINT ( 'NONE',  ( 0.6152055445548323398, -5.969096820685134475, 25.29904968670267351 ) ) ;
#3851=EDGE_CURVE ( 'NONE', #15393, #11257, #6052, .T. ) ;
#3853=ORIENTED_EDGE ( 'NONE', *, *, #5899, .T. ) ;
#3855=CARTESIAN_POINT ( 'NONE',  ( -5.903057025253910517, 1.078199533779480745, 12.11561732698603855 ) ) ;
#3856=CARTESIAN_POINT ( 'NONE',  ( -5.570722351696290708, 2.834100162821917124, 30.73809786915987630 ) ) ;
#3858=CARTESIAN_POINT ( 'NONE',  ( 2.030576276931546336E-13, 6.000000000000000888, 25.49999999999999645 ) ) ;
#3861=CARTESIAN_POINT ( 'NONE',  ( 7.490007020835686369, -2.433650805992243260, 5.000000000000004441 ) ) ;
#3863=DIRECTION ( 'NONE',  ( -0.5877852522924685852, -0.8090169943749507819, 0.000000000000000000 ) ) ;
#3864=CARTESIAN_POINT ( 'NONE',  ( -0.9737725088282058739, -6.173885267451823644, 30.73735758726567013 ) ) ;
#3870=B_SPLINE_CURVE_WITH_KNOTS ( 'NONE', 3,
 ( #6112, #9842, #7375, #5947, #11978, #3468, #1159, #14613, #3628, #13489, #7143, #3550, #1313, #6028, #4991, #10949, #13412, #4914 ),
 .UNSPECIFIED., .F., .F.,
 ( 4, 2, 2, 2, 2, 2, 2, 2, 4 ),
 ( 0.003131486019301987257, 0.003522824630466694397, 0.003914163241631401537, 0.004305501852796108676, 0.004696840463960815816, 0.005088179075125522956, 0.005479517686290230095, 0.005870856297454937235, 0.006262194908619644375 ),
 .UNSPECIFIED. ) ;
#3873=CARTESIAN_POINT ( 'NONE',  ( -5.621278735166176155, -2.101423246382613463, 18.97408052783099563 ) ) ;
#3879=CARTESIAN_POINT ( 'NONE',  ( 2.930922878467467019, -5.520395124723577851, 17.49610786875028623 ) ) ;
#3881=CARTESIAN_POINT ( 'NONE',  ( -0.8730628416136632097, -6.188929913094972868, 10.99504929893116767 ) ) ;
#3886=CARTESIAN_POINT ( 'NONE',  ( -0.5030929395818956040, -6.230885867001155987, 17.12600319116547709 ) ) ;
#3887=CARTESIAN_POINT ( 'NONE',  ( -7.180990026460683850, -3.384707322287710873, 24.49999999999999289 ) ) ;
#3891=ORIENTED_EDGE ( 'NONE', *, *, #2375, .F. ) ;
#3892=DIRECTION ( 'NONE',  ( -0.9510565162951544194, 0.3090169943749447312, 0.000000000000000000 ) ) ;
#3898=CARTESIAN_POINT ( 'NONE',  ( 5.558508435838253270, 2.857531096718811892, 18.13234125634167526 ) ) ;
#3900=CYLINDRICAL_SURFACE ( 'NONE', #568, 1.000000000000000666 ) ;
#3903=CARTESIAN_POINT ( 'NONE',  ( -3.736532060718099402, 4.696070028785882755, 17.02622176056705783 ) ) ;
#3905=CARTESIAN_POINT ( 'NONE',  ( -6.176542424588072677, -0.9554180641288341214, 24.49999999999999289 ) ) ;
#3907=CARTESIAN_POINT ( 'NONE',  ( 5.558508435838262152, -2.857531096718793240, 11.36765874365828743 ) ) ;
#3909=ORIENTED_EDGE ( 'NONE', *, *, #9693, .F. ) ;
#3912=CARTESIAN_POINT ( 'NONE',  ( 5.935543223013863390, -0.8771126767606431951, 30.86938304467861727 ) ) ;
#3914=VERTEX_POINT ( 'NONE', #8757 ) ;
#3915=CARTESIAN_POINT ( 'NONE',  ( -1.000079958708137928, -5.916066267613700802, 5.131527388820333435 ) ) ;
#3916=CARTESIAN_POINT ( 'NONE',  ( -3.923477796648590754, -4.541042560386415516, 18.87303779027050155 ) ) ;
#3917=CARTESIAN_POINT ( 'NONE',  ( 4.069684453406231306, -4.744965295353614110, 23.62619944752604084 ) ) ;
#3921=CARTESIAN_POINT ( 'NONE',  ( -4.435347140101121965, 4.403429997944421359, 11.49999999999998224 ) ) ;
#3922=CARTESIAN_POINT ( 'NONE',  ( 0.9735856429314875271, -5.920699391844991943, 24.76285283906726065 ) ) ;
#3929=VERTEX_POINT ( 'NONE', #10819 ) ;
#3930=LINE ( 'NONE', #6424, #223 ) ;
#3932=DIRECTION ( 'NONE',  ( 0.5877852522924802425, -0.8090169943749422332, 0.000000000000000000 ) ) ;
#3933=CARTESIAN_POINT ( 'NONE',  ( 6.768587589771821120E-14, -6.250000000000000888, 12.49999999999998401 ) ) ;
#3934=CARTESIAN_POINT ( 'NONE',  ( 5.726049995854468833, 2.506679546901878552, 12.29954462468842991 ) ) ;
#3936=CARTESIAN_POINT ( 'NONE',  ( 4.435347140101010943, 4.403429997944536822, 5.132374107163055754 ) ) ;
#3938=CARTESIAN_POINT ( 'NONE',  ( 7.490007020835692586, -2.433650805992223720, 31.00000000000000000 ) ) ;
#3939=EDGE_CURVE ( 'NONE', #5534, #11257, #1186, .T. ) ;
#3940=DIRECTION ( 'NONE',  ( 0.8090169943749421222, 0.5877852522924802425, 0.000000000000000000 ) ) ;
#3943=EDGE_CURVE ( 'NONE', #15370, #7094, #13983, .T. ) ;
#3946=CARTESIAN_POINT ( 'NONE',  ( 5.770331821586490051, -2.404225004693387291, 25.37380055247395561 ) ) ;
#3947=B_SPLINE_CURVE_WITH_KNOTS ( 'NONE', 3,
 ( #105, #13544, #5123, #11316, #9976, #415, #7581, #5047, #5285, #14752, #12430, #2886, #1530, #6405, #11237, #339, #5201, #10054 ),
 .UNSPECIFIED., .F., .F.,
 ( 4, 2, 2, 2, 2, 2, 2, 2, 4 ),
 ( 0.003131923598876997471, 0.003523316383094315246, 0.003914709167311632154, 0.004306101951528949930, 0.004697494735746267705, 0.005088887519963585480, 0.005480280304180903256, 0.005871673088398220164, 0.006263065872615537939 ),
 .UNSPECIFIED. ) ;
#3950=CARTESIAN_POINT ( 'NONE',  ( -5.842945980534627104, -1.369128644669050043, 18.87378430870261781 ) ) ;
#3951=CIRCLE ( 'NONE', #15139, 6.250000000000000888 ) ;
#3954=CARTESIAN_POINT ( 'NONE',  ( -7.490007020835664164, -2.433650805992495503, 17.99999999999998934 ) ) ;
#3955=ADVANCED_FACE ( 'NONE', ( #12398 ), #7785, .F. ) ;
#3960=CARTESIAN_POINT ( 'NONE',  ( 4.195795028114952530, 4.289273350251397332, 17.49571079637979309 ) ) ;
#3964=CARTESIAN_POINT ( 'NONE',  ( -4.435347140101088215, 4.403429997944455998, 30.86939309276502641 ) ) ;
#3965=CYLINDRICAL_SURFACE ( 'NONE', #665, 1.000000000000000222 ) ;
#3966=CYLINDRICAL_SURFACE ( 'NONE', #7713, 1.000000000000000888 ) ;
#3967=ORIENTED_EDGE ( 'NONE', *, *, #13803, .F. ) ;
#3969=ORIENTED_EDGE ( 'NONE', *, *, #10127, .F. ) ;
#3970=CARTESIAN_POINT ( 'NONE',  ( -5.746996058422734421, 1.729015645942056478, 25.50007961174475923 ) ) ;
#3972=DIRECTION ( 'NONE',  ( 1.000000000000000000, 0.000000000000000000, 0.000000000000000000 ) ) ;
#3980=CARTESIAN_POINT ( 'NONE',  ( -7.490007020835684592, -2.433650805992431110, 11.49999999999998224 ) ) ;
#3981=CARTESIAN_POINT ( 'NONE',  ( 3.735808404765050827, -4.696639218303082508, 31.97398020122238549 ) ) ;
#3983=ADVANCED_FACE ( 'NONE', ( #15108 ), #1730, .F. ) ;
#3984=CARTESIAN_POINT ( 'NONE',  ( 5.649200442566201019, -2.675373855294060910, 10.88439807107078572 ) ) ;
#3985=CARTESIAN_POINT ( 'NONE',  ( -0.8738043859790617374, 6.188821459035881212, 31.50341560223747450 ) ) ;
#3989=EDGE_CURVE ( 'NONE', #4626, #9974, #616, .T. ) ;
#3990=VERTEX_POINT ( 'NONE', #8916 ) ;
#3995=CARTESIAN_POINT ( 'NONE',  ( 0.7988860301922214857, 6.199427171881336740, 4.384555805361944891 ) ) ;
#3996=B_SPLINE_CURVE_WITH_KNOTS ( 'NONE', 3,
 ( #5142, #359, #15007, #5225, #8806, #4013, #8728, #1549, #9839, #4097, #6343, #8967, #12367, #13635, #433, #10072, #11180, #11336 ),
 .UNSPECIFIED., .F., .F.,
 ( 4, 2, 2, 2, 2, 2, 2, 2, 4 ),
 ( 0.000000000000000000, 0.0003914357524127463472, 0.0007828715048254926943, 0.001174307257238239042, 0.001565743009650985389, 0.001957178762063731953, 0.002348614514476478083, 0.002740050266889224213, 0.003131486019301970777 ),
 .UNSPECIFIED. ) ;
#3997=CARTESIAN_POINT ( 'NONE',  ( 0.7993282387951309298, -5.947240459526506484, 31.61484358216957347 ) ) ;
#3999=CARTESIAN_POINT ( 'NONE',  ( -0.7993401192311065939, 6.199366368793671533, 18.61483246936565550 ) ) ;
#4000=CARTESIAN_POINT ( 'NONE',  ( 0.1323408341374927855, 6.250000000000000888, 19.00000000000000711 ) ) ;
#4002=SURFACE_STYLE_FILL_AREA ( #13711 ) ;
#4003=CARTESIAN_POINT ( 'NONE',  ( -3.255013540813682660, 5.336859797930809890, 10.62618035954927898 ) ) ;
#4012=EDGE_LOOP ( 'NONE', ( #13617, #3294, #10826, #11850 ) ) ;
#4013=CARTESIAN_POINT ( 'NONE',  ( -6.105925084677680914, 1.337450587213181441, 17.20066851092422411 ) ) ;
#4014=CARTESIAN_POINT ( 'NONE',  ( 3.883716939929109380, -4.898343590941151682, 10.52640428276697548 ) ) ;
#4019=CARTESIAN_POINT ( 'NONE',  ( 3.159612573729236651, 5.393342049074624001, 5.800265150176763029 ) ) ;
#4021=CARTESIAN_POINT ( 'NONE',  ( 2.782156709077406642, 5.316215864844050287, 4.496879510976234506 ) ) ;
#4025=FACE_BOUND ( 'NONE', #3019, .T. ) ;
#4028=CARTESIAN_POINT ( 'NONE',  ( -2.817313151351169775, -5.579000502529442684, 11.49999999999998224 ) ) ;
#4030=CARTESIAN_POINT ( 'NONE',  ( 5.531796221294920990, 2.326749136277109109, 23.62621569129737509 ) ) ;
#4032=CARTESIAN_POINT ( 'NONE',  ( -3.632151824461173462, 4.777505256984529325, 19.00004932073311181 ) ) ;
#4033=VECTOR ( 'NONE', #6400, 1000.000000000000114 ) ;
#4035=VERTEX_POINT ( 'NONE', #13901 ) ;
#4036=EDGE_CURVE ( 'NONE', #8231, #14335, #3012, .T. ) ;
#4037=CARTESIAN_POINT ( 'NONE',  ( -3.779082820360704087, -4.979770177899243144, 16.99995093123465750 ) ) ;
#4038=CARTESIAN_POINT ( 'NONE',  ( 5.935543223013860725, -0.8771126767606638452, 5.130649613488545313 ) ) ;
#4039=ADVANCED_BREP_SHAPE_REPRESENTATION ( '', ( #15531, #14201 ), #10667 ) ;
#4040=CARTESIAN_POINT ( 'NONE',  ( -5.935543223013861613, 0.8771126767606655106, 5.000000000000004441 ) ) ;
#4043=CARTESIAN_POINT ( 'NONE',  ( 5.935543223013889147, -0.8771126767604600083, 24.63064961348855775 ) ) ;
#4046=CARTESIAN_POINT ( 'NONE',  ( 4.005785023174528447, -4.467917056767334749, 5.799520541027148646 ) ) ;
#4047=CARTESIAN_POINT ( 'NONE',  ( 6.176542424588119751, -0.9554180641285445752, 5.130639327542137806 ) ) ;
#4048=CARTESIAN_POINT ( 'NONE',  ( 0.000000000000000000, 0.000000000000000000, 36.00000000000000711 ) ) ;
#4049=CARTESIAN_POINT ( 'NONE',  ( -5.409007216690642217, -2.598315788643811963, 10.88557478428061032 ) ) ;
#4053=DIRECTION ( 'NONE',  ( -0.3090169943749446202, -0.9510565162951544194, 0.000000000000000000 ) ) ;
#4056=EDGE_LOOP ( 'NONE', ( #15006, #4955 ) ) ;
#4058=CARTESIAN_POINT ( 'NONE',  ( 2.030576276931546336E-13, -6.250000000000000888, 24.49999999999999289 ) ) ;
#4061=CARTESIAN_POINT ( 'NONE',  ( 1.000079958708139261, 5.916066267613699026, 5.131527388820331659 ) ) ;
#4066=CARTESIAN_POINT ( 'NONE',  ( -2.817313151351291012, -5.579000502529380512, 24.49999999999999289 ) ) ;
#4071=CARTESIAN_POINT ( 'NONE',  ( 5.131373506000599605, 7.062729720844090231, 5.000000000000004441 ) ) ;
#4072=CARTESIAN_POINT ( 'NONE',  ( 1.353717517954364224E-13, -6.000000000000000888, 18.99999999999998934 ) ) ;
#4073=EDGE_LOOP ( 'NONE', ( #802, #3822 ) ) ;
#4074=EDGE_LOOP ( 'NONE', ( #13616, #6834, #4532, #2669 ) ) ;
#4079=CARTESIAN_POINT ( 'NONE',  ( 0.8730628416137207193, 6.188929913094963986, 4.495049298931171222 ) ) ;
#4081=CARTESIAN_POINT ( 'NONE',  ( 1.000049560716574026, -5.916071405810141570, 30.86967799011530644 ) ) ;
#4082=CARTESIAN_POINT ( 'NONE',  ( -5.375605342016534394, 2.665598297262232741, 5.503120489023787698 ) ) ;
#4086=CARTESIAN_POINT ( 'NONE',  ( -4.070051655338214225, 4.744673454622383879, 18.87367328635991726 ) ) ;
#4089=B_SPLINE_CURVE_WITH_KNOTS ( 'NONE', 3,
 ( #2693, #8751, #1411, #6369, #7545, #10020, #14867, #12551, #4201, #11127, #13583, #2932, #5249, #14791, #7471, #6524, #10095, #6285 ),
 .UNSPECIFIED., .F., .F.,
 ( 4, 2, 2, 2, 2, 2, 2, 2, 4 ),
 ( 0.000000000000000000, 0.0003914357524127506840, 0.0007828715048255013680, 0.001174307257238252052, 0.001565743009651002736, 0.001957178762063753637, 0.002348614514476504104, 0.002740050266889254571, 0.003131486019302005472 ),
 .UNSPECIFIED. ) ;
#4094=EDGE_LOOP ( 'NONE', ( #12733, #10032 ) ) ;
#4097=CARTESIAN_POINT ( 'NONE',  ( -5.903843691985208864, 2.055287728870709874, 16.99995093123465750 ) ) ;
#4098=CARTESIAN_POINT ( 'NONE',  ( -5.558508435838136919, 2.857531096719036601, 24.36936067245786930 ) ) ;
#4099=CARTESIAN_POINT ( 'NONE',  ( -0.9740856415300837012, 6.173834621338593287, 4.738526530555331462 ) ) ;
#4101=EDGE_CURVE ( 'NONE', #11546, #3364, #6527, .T. ) ;
#4103=ADVANCED_FACE ( 'NONE', ( #5335 ), #9374, .F. ) ;
#4104=CARTESIAN_POINT ( 'NONE',  ( 4.267936573529151012, -4.217499624512297984, 24.23770962164067200 ) ) ;
#4106=CARTESIAN_POINT ( 'NONE',  ( 2.668367453516629517, 5.373994336898132218, 5.000000000000004441 ) ) ;
#4108=CARTESIAN_POINT ( 'NONE',  ( 5.935543223013846514, 0.8771126767607477781, 5.000000000000004441 ) ) ;
#4116=CARTESIAN_POINT ( 'NONE',  ( -3.311384659207262882, 5.004923837169336309, 18.97358595436693207 ) ) ;
#4119=CARTESIAN_POINT ( 'NONE',  ( -3.567624405365327878, -5.133384272590721054, 17.00004921015705861 ) ) ;
#4125=DIRECTION ( 'NONE',  ( 0.000000000000000000, 1.000000000000000000, 0.000000000000000000 ) ) ;
#4126=CARTESIAN_POINT ( 'NONE',  ( 5.317509234264001350, -2.779225709350912954, 11.49999999999998224 ) ) ;
#4127=CARTESIAN_POINT ( 'NONE',  ( 7.490007020835706797, -2.433650805992179755, 11.49999999999998224 ) ) ;
#4129=CARTESIAN_POINT ( 'NONE',  ( -5.935543223013839409, -0.8771126767608162789, 11.36763921416086554 ) ) ;
#4130=EDGE_LOOP ( 'NONE', ( #11932, #1000, #3119, #8503 ) ) ;
#4132=ORIENTED_EDGE ( 'NONE', *, *, #7757, .F. ) ;
#4133=CARTESIAN_POINT ( 'NONE',  ( -5.935543223013831415, 0.8771126767608680153, 24.49999999999999289 ) ) ;
#4136=LINE ( 'NONE', #2869, #13682 ) ;
#4138=CARTESIAN_POINT ( 'NONE',  ( -3.312341048453360415, -5.004306261885527185, 5.973980201222397923 ) ) ;
#4140=CARTESIAN_POINT ( 'NONE',  ( -0.5043776560896817696, 6.230795654995842980, 25.37337476296002947 ) ) ;
#4143=CARTESIAN_POINT ( 'NONE',  ( -4.196288036172528990, 4.288789315524756951, 17.49687951097622474 ) ) ;
#4144=ADVANCED_FACE ( 'NONE', ( #7069 ), #12782, .F. ) ;
#4148=CARTESIAN_POINT ( 'NONE',  ( 3.421280866381083641, 4.930711975950953452, 12.50004932073310471 ) ) ;
#4149=ADVANCED_FACE ( 'NONE', ( #6840 ), #12944, .F. ) ;
#4150=VERTEX_POINT ( 'NONE', #10412 ) ;
#4151=ORIENTED_EDGE ( 'NONE', *, *, #10955, .F. ) ;
#4153=VERTEX_POINT ( 'NONE', #655 ) ;
#4154=CARTESIAN_POINT ( 'NONE',  ( 4.153440676704430956, -4.671190581744464332, 12.29954462468842813 ) ) ;
#4156=B_SPLINE_CURVE_WITH_KNOTS ( 'NONE', 3,
 ( #4350, #9285, #10319, #5476, #8169, #14121, #764, #1795, #3227, #9209, #11738, #8008, #12930, #12849, #5628, #10475, #9135, #12769 ),
 .UNSPECIFIED., .F., .F.,
 ( 4, 2, 2, 2, 2, 2, 2, 2, 4 ),
 ( 0.003131918686235975191, 0.003523310662250265460, 0.003914702638264555730, 0.004306094614278846433, 0.004697486590293136269, 0.005088878566307426972, 0.005480270542321717675, 0.005871662518336007511, 0.006263054494350298214 ),
 .UNSPECIFIED. ) ;
#4157=VERTEX_POINT ( 'NONE', #14250 ) ;
#4160=CARTESIAN_POINT ( 'NONE',  ( 0.7993401192313105419, -6.199366368793645776, 18.61483246936574432 ) ) ;
#4161=EDGE_CURVE ( 'NONE', #6307, #2787, #2430, .T. ) ;
#4162=CARTESIAN_POINT ( 'NONE',  ( -5.665308849928848645, 1.980336949702434790, 5.999920023562623328 ) ) ;
#4165=CARTESIAN_POINT ( 'NONE',  ( -4.322356511625788045, 7.650514973136498753, 31.00000000000000000 ) ) ;
#4171=CARTESIAN_POINT ( 'NONE',  ( 4.286401442266591921, -4.198423832313132209, 5.000000000000004441 ) ) ;
#4177=CARTESIAN_POINT ( 'NONE',  ( 0.6139731865240710684, -6.220476368274045598, 10.69975545601931799 ) ) ;
#4178=CYLINDRICAL_SURFACE ( 'NONE', #13943, 1.000000000000000888 ) ;
#4180=CARTESIAN_POINT ( 'NONE',  ( 3.922288969639700529, -4.542045818322596240, 23.62621569129737154 ) ) ;
#4181=EDGE_CURVE ( 'NONE', #12139, #2516, #8147, .T. ) ;
#4182=CARTESIAN_POINT ( 'NONE',  ( 6.176542424588121527, -0.9554180641285238140, 31.00000000000000000 ) ) ;
#4184=CARTESIAN_POINT ( 'NONE',  ( -3.420311045507770764, -4.931422832349343643, 32.00007961174477344 ) ) ;
#4185=CARTESIAN_POINT ( 'NONE',  ( -2.997451966578355886, -5.485105005466039074, 30.38482219624157565 ) ) ;
#4187=AXIS2_PLACEMENT_3D ( 'NONE', #5193, #6159, #255 ) ;
#4190=LINE ( 'NONE', #11737, #2459 ) ;
#4191=EDGE_CURVE ( 'NONE', #11875, #11314, #12308, .T. ) ;
#4192=CARTESIAN_POINT ( 'NONE',  ( -4.152999119457986055, -4.671604476854346544, 10.69973484982324052 ) ) ;
#4195=CARTESIAN_POINT ( 'NONE',  ( -5.329907877631296031, -2.755840666746375511, 18.26194324003145653 ) ) ;
#4196=EDGE_CURVE ( 'NONE', #14255, #11999, #8150, .T. ) ;
#4199=CARTESIAN_POINT ( 'NONE',  ( -4.344502777243583580, -4.493369211529213203, 17.49610786875029689 ) ) ;
#4201=CARTESIAN_POINT ( 'NONE',  ( 5.903596343266319657, -2.055998103990523518, 12.49995078984291830 ) ) ;
#4202=B_SPLINE_CURVE_WITH_KNOTS ( 'NONE', 3,
 ( #12109, #2490, #14329, #10840, #7348, #3521, #24, #4886, #4968, #3436, #12190, #7194, #11950, #1289, #6163, #9819, #1132, #10766 ),
 .UNSPECIFIED., .F., .F.,
 ( 4, 2, 2, 2, 2, 2, 2, 2, 4 ),
 ( 0.003131486019301987257, 0.003522824630466693530, 0.003914163241631398935, 0.004305501852796105207, 0.004696840463960811479, 0.005088179075125518619, 0.005479517686290224891, 0.005870856297454931164, 0.006262194908619638303 ),
 .UNSPECIFIED. ) ;
#4206=CARTESIAN_POINT ( 'NONE',  ( 7.180990026460741582, -3.384707322287397790, 5.000000000000004441 ) ) ;
#4207=CARTESIAN_POINT ( 'NONE',  ( -2.817313151351249711, 5.579000502529400940, 11.49999999999998224 ) ) ;
#4209=CARTESIAN_POINT ( 'NONE',  ( 5.858736126997154514, -2.179962889277010873, 5.973595717233013858 ) ) ;
#4211=CARTESIAN_POINT ( 'NONE',  ( -5.935543223013836744, -0.8771126767608161678, 11.49999999999998224 ) ) ;
#4212=EDGE_LOOP ( 'NONE', ( #12683, #13543 ) ) ;
#4215=CARTESIAN_POINT ( 'NONE',  ( -5.915641100987789613, -1.003868594704996342, 23.99571079637979665 ) ) ;
#4216=ORIENTED_EDGE ( 'NONE', *, *, #13485, .F. ) ;
#4217=LINE ( 'NONE', #13914, #10145 ) ;
#4218=DIRECTION ( 'NONE',  ( 0.000000000000000000, 0.000000000000000000, 1.000000000000000000 ) ) ;
#4220=CARTESIAN_POINT ( 'NONE',  ( -0.1323933160974262724, 6.000000000000003553, 18.99999999999998934 ) ) ;
#4221=CARTESIAN_POINT ( 'NONE',  ( -4.416678568553632722, -4.422441866694328816, 5.262369734438752999 ) ) ;
#4223=CARTESIAN_POINT ( 'NONE',  ( -6.081464507797627483, -1.446657058464217327, 5.873800552473966263 ) ) ;
#4224=DIRECTION ( 'NONE',  ( 0.000000000000000000, 1.000000000000000000, 0.000000000000000000 ) ) ;
#4225=DIRECTION ( 'NONE',  ( -0.3090169943749446202, -0.9510565162951544194, 0.000000000000000000 ) ) ;
#4227=CARTESIAN_POINT ( 'NONE',  ( 2.848235266350948702, 5.281699484015686785, 12.11397738943082736 ) ) ;
#4228=EDGE_CURVE ( 'NONE', #6465, #8099, #9659, .T. ) ;
#4233=CARTESIAN_POINT ( 'NONE',  ( 4.344265632482078310, -4.493596842504967270, 18.50425949503009448 ) ) ;
#4236=CARTESIAN_POINT ( 'NONE',  ( 5.931828553037993501, -0.9033193133617988257, 18.26194324003146008 ) ) ;
#4239=CARTESIAN_POINT ( 'NONE',  ( -5.903057025253926504, 1.078199533779401253, 5.615617326986045654 ) ) ;
#4240=CARTESIAN_POINT ( 'NONE',  ( 5.649200442566188585, -2.675373855294086667, 30.38439807107076973 ) ) ;
#4242=CARTESIAN_POINT ( 'NONE',  ( -5.131373506000823426, 7.062729720843950787, 17.99999999999998934 ) ) ;
#4243=CARTESIAN_POINT ( 'NONE',  ( 5.843318061569063637, 1.367618216965549749, 18.87303779027049444 ) ) ;
#4246=CARTESIAN_POINT ( 'NONE',  ( -5.620879908643960476, -2.102487719021914003, 4.026221760567070262 ) ) ;
#4249=ORIENTED_EDGE ( 'NONE', *, *, #6301, .T. ) ;
#4252=ORIENTED_EDGE ( 'NONE', *, *, #3989, .T. ) ;
#4253=CARTESIAN_POINT ( 'NONE',  ( -0.7993401192311344605, 6.199366368793667981, 12.11483246936570524 ) ) ;
#4260=CARTESIAN_POINT ( 'NONE',  ( 3.883716939929077849, 4.898343590941176551, 5.973595717233015634 ) ) ;
#4261=CARTESIAN_POINT ( 'NONE',  ( 2.817313151351065859, -5.579000502529494199, 17.99999999999998934 ) ) ;
#4269=FACE_BOUND ( 'NONE', #4073, .T. ) ;
#4270=CARTESIAN_POINT ( 'NONE',  ( -7.180990026460747799, -3.384707322287517695, 5.000000000000004441 ) ) ;
#4274=VECTOR ( 'NONE', #4529, 1000.000000000000114 ) ;
#4276=ORIENTED_EDGE ( 'NONE', *, *, #12836, .F. ) ;
#4278=VECTOR ( 'NONE', #462, 1000.000000000000000 ) ;
#4279=CARTESIAN_POINT ( 'NONE',  ( -0.5030929395820217254, -6.230885867001147105, 4.126003191165496631 ) ) ;
#4280=ADVANCED_FACE ( 'NONE', ( #1130 ), #10838, .F. ) ;
#4281=CARTESIAN_POINT ( 'NONE',  ( -5.931817299736832361, 0.9033986943603389275, 24.23770962164067200 ) ) ;
#4286=CIRCLE ( 'NONE', #14709, 6.000000000000000888 ) ;
#4287=CARTESIAN_POINT ( 'NONE',  ( 5.649200442566265856, -2.675373855293923686, 23.88439807107078039 ) ) ;
#4288=CARTESIAN_POINT ( 'NONE',  ( -5.570722351696298702, 2.834100162821898916, 4.738097869159890507 ) ) ;
#4289=CARTESIAN_POINT ( 'NONE',  ( -3.922672396097018233, -4.541739265057732844, 30.12635295315576656 ) ) ;
#4290=ORIENTED_EDGE ( 'NONE', *, *, #2340, .T. ) ;
#4294=DIRECTION ( 'NONE',  ( 0.8090169943749421222, 0.5877852522924802425, 0.000000000000000000 ) ) ;
#4299=CARTESIAN_POINT ( 'NONE',  ( 0.1323602877612205797, 6.000000000000001776, 6.000000000000007105 ) ) ;
#4302=CARTESIAN_POINT ( 'NONE',  ( 5.665707375537527568, -1.979196487016524175, 23.49992038825522300 ) ) ;
#4304=CARTESIAN_POINT ( 'NONE',  ( -6.155867707731109917, -1.081837891425901921, 5.504369696801525436 ) ) ;
#4306=CYLINDRICAL_SURFACE ( 'NONE', #6487, 1.000000000000000666 ) ;
#4307=CARTESIAN_POINT ( 'NONE',  ( 2.930922878467487003, 5.520395124723568081, 31.50389213124968890 ) ) ;
#4308=CARTESIAN_POINT ( 'NONE',  ( -0.6151877315909831667, 6.220340188096017187, 31.79906673469668732 ) ) ;
#4309=ORIENTED_EDGE ( 'NONE', *, *, #12116, .T. ) ;
#4313=ORIENTED_EDGE ( 'NONE', *, *, #9207, .F. ) ;
#4314=CARTESIAN_POINT ( 'NONE',  ( -5.858813228503623627, -2.179803269293346002, 10.52622717124729412 ) ) ;
#4316=ORIENTED_EDGE ( 'NONE', *, *, #2542, .F. ) ;
#4318=CARTESIAN_POINT ( 'NONE',  ( -5.931817299736849236, -0.9033986943602401176, 31.26229037835932090 ) ) ;
#4320=CARTESIAN_POINT ( 'NONE',  ( -2.817313151351109379, -5.579000502529471994, 5.000000000000004441 ) ) ;
#4324=CARTESIAN_POINT ( 'NONE',  ( 3.106366801611939010, 5.134708448381321233, 10.62696220972947181 ) ) ;
#4325=B_SPLINE_CURVE_WITH_KNOTS ( 'NONE', 3,
 ( #1838, #3194, #3042, #725, #10518, #12736, #6638, #12665, #5364, #15293, #9174, #2965, #4154, #3120, #8132, #15061, #1762, #11468 ),
 .UNSPECIFIED., .F., .F.,
 ( 4, 2, 2, 2, 2, 2, 2, 2, 4 ),
 ( 0.003131486019301968175, 0.003522824630466676616, 0.003914163241631385057, 0.004305501852796093064, 0.004696840463960801071, 0.005088179075125509945, 0.005479517686290218820, 0.005870856297454928562, 0.006262194908619637436 ),
 .UNSPECIFIED. ) ;
#4330=B_SPLINE_CURVE_WITH_KNOTS ( 'NONE', 3,
 ( #13494, #4997, #9849, #7307, #1167, #2361, #13181, #3557, #9698, #6120, #9357, #14535, #13421, #8510, #8587, #15657, #5954, #11111 ),
 .UNSPECIFIED., .F., .F.,
 ( 4, 2, 2, 2, 2, 2, 2, 2, 4 ),
 ( 0.003131486019301969476, 0.003522824630466678351, 0.003914163241631387659, 0.004305501852796096533, 0.004696840463960805408, 0.005088179075125515149, 0.005479517686290224024, 0.005870856297454932898, 0.006262194908619641773 ),
 .UNSPECIFIED. ) ;
#4332=EDGE_LOOP ( 'NONE', ( #10442, #4892, #5062, #9176 ) ) ;
#4335=CYLINDRICAL_SURFACE ( 'NONE', #8619, 1.000000000000000666 ) ;
#4336=DIRECTION ( 'NONE',  ( -0.3090169943749446202, -0.9510565162951544194, 0.000000000000000000 ) ) ;
#4337=CARTESIAN_POINT ( 'NONE',  ( -0.5044069930203394225, 5.979990686694992341, 5.873357432279042278 ) ) ;
#4338=ORIENTED_EDGE ( 'NONE', *, *, #364, .T. ) ;
#4340=CARTESIAN_POINT ( 'NONE',  ( -1.000082492230513820, -6.169467968613740361, 24.63152538105391187 ) ) ;
#4343=CARTESIAN_POINT ( 'NONE',  ( 3.106366801611989636, 5.134708448381291035, 4.126962209729496678 ) ) ;
#4344=CARTESIAN_POINT ( 'NONE',  ( -7.180990026460740694, -3.384707322287537679, 31.00000000000000000 ) ) ;
#4346=ADVANCED_FACE ( 'NONE', ( #2488 ), #7346, .F. ) ;
#4349=FACE_BOUND ( 'NONE', #13700, .T. ) ;
#4350=CARTESIAN_POINT ( 'NONE',  ( -5.317509234263906315, 2.779225709351095475, 17.99999999999998934 ) ) ;
#4354=CARTESIAN_POINT ( 'NONE',  ( 3.253823204785034839, -5.337590213880554657, 25.37305891554299464 ) ) ;
#4356=ORIENTED_EDGE ( 'NONE', *, *, #3349, .F. ) ;
#4358=B_SPLINE_CURVE_WITH_KNOTS ( 'NONE', 3,
 ( #13448, #4947, #5979, #8452, #9798, #14648, #1349, #14729, #6224, #3816, #13519, #2626, #7482, #12326, #7874, #2783, #13671, #6459 ),
 .UNSPECIFIED., .F., .F.,
 ( 4, 2, 2, 2, 2, 2, 2, 2, 4 ),
 ( 0.003131918686235980395, 0.003523310662250270665, 0.003914702638264560934, 0.004306094614278851637, 0.004697486590293141473, 0.005088878566307432176, 0.005480270542321721144, 0.005871662518336010980, 0.006263054494350299949 ),
 .UNSPECIFIED. ) ;
#4364=CARTESIAN_POINT ( 'NONE',  ( -5.783239563508415948, -1.602707436861142032, 5.973585954366939177 ) ) ;
#4366=CARTESIAN_POINT ( 'NONE',  ( 6.105747081304177648, -1.338335777572248420, 5.800265150176761253 ) ) ;
#4367=CARTESIAN_POINT ( 'NONE',  ( -5.903843691985250608, 2.055287728870591746, 3.999950931234677487 ) ) ;
#4368=VECTOR ( 'NONE', #6192, 1000.000000000000114 ) ;
#4369=DIRECTION ( 'NONE',  ( 0.8090169943749506709, -0.5877852522924689183, 0.000000000000000000 ) ) ;
#4370=ORIENTED_EDGE ( 'NONE', *, *, #11646, .F. ) ;
#4373=CARTESIAN_POINT ( 'NONE',  ( -4.435347140101057128, -4.403429997944487084, 11.49999999999998224 ) ) ;
#4377=ADVANCED_FACE ( 'NONE', ( #5040 ), #13612, .F. ) ;
#4378=AXIS2_PLACEMENT_3D ( 'NONE', #11612, #10505, #6935 ) ;
#4379=DIRECTION ( 'NONE',  ( 0.9510565162951499785, 0.3090169943749582204, 0.000000000000000000 ) ) ;
#4380=CARTESIAN_POINT ( 'NONE',  ( -2.782713018890655476, 5.315928322779151394, 31.50439760644212939 ) ) ;
#4381=CARTESIAN_POINT ( 'NONE',  ( 2.841163418881270886, 5.567120626447992215, 17.73763026556123634 ) ) ;
#4383=CARTESIAN_POINT ( 'NONE',  ( -2.931212650151567178, -5.520239928492866710, 5.504259495030093596 ) ) ;
#4384=EDGE_CURVE ( 'NONE', #7314, #1512, #11023, .T. ) ;
#4386=CARTESIAN_POINT ( 'NONE',  ( -6.155854678529475876, -1.081900940642102737, 4.495740504969913509 ) ) ;
#4389=CARTESIAN_POINT ( 'NONE',  ( -5.531209434046278517, -2.328189801702761130, 17.12696220972947714 ) ) ;
#4390=CARTESIAN_POINT ( 'NONE',  ( -0.8730424326979571159, -5.936362132114481049, 17.49500690218562582 ) ) ;
#4391=ORIENTED_EDGE ( 'NONE', *, *, #92, .F. ) ;
#4392=EDGE_CURVE ( 'NONE', #14489, #12984, #11077, .T. ) ;
#4394=ORIENTED_EDGE ( 'NONE', *, *, #7177, .T. ) ;
#4395=ORIENTED_EDGE ( 'NONE', *, *, #792, .T. ) ;
#4396=CARTESIAN_POINT ( 'NONE',  ( 3.311576095066486314, -5.004818610361370546, 25.47377823943293862 ) ) ;
#4401=CARTESIAN_POINT ( 'NONE',  ( 6.081836621194454118, 1.445163676684769749, 18.87305891554299464 ) ) ;
#4404=AXIS2_PLACEMENT_3D ( 'NONE', #11699, #3416, #9477 ) ;
#4412=ORIENTED_EDGE ( 'NONE', *, *, #6167, .F. ) ;
#4414=VECTOR ( 'NONE', #5011, 1000.000000000000000 ) ;
#4416=CARTESIAN_POINT ( 'NONE',  ( -0.6139731865239230757, 6.220476368274060697, 10.69975545601930556 ) ) ;
#4418=CARTESIAN_POINT ( 'NONE',  ( 5.558508435838283468, 2.857531096718750607, 24.49999999999999289 ) ) ;
#4421=DIRECTION ( 'NONE',  ( 0.000000000000000000, 1.000000000000000000, 0.000000000000000000 ) ) ;
#4423=DIRECTION ( 'NONE',  ( -0.5877852522924685852, -0.8090169943749508930, 0.000000000000000000 ) ) ;
#4427=CARTESIAN_POINT ( 'NONE',  ( 6.081836621194475434, -1.445163676684684484, 17.12694108445698760 ) ) ;
#4428=DIRECTION ( 'NONE',  ( 0.9510565162951499785, 0.3090169943749582204, 0.000000000000000000 ) ) ;
#4431=CARTESIAN_POINT ( 'NONE',  ( 4.290130679986473794, -4.545972905167823264, 25.11560192892922316 ) ) ;
#4434=CARTESIAN_POINT ( 'NONE',  ( -5.131373506000823426, 7.062729720843950787, 17.99999999999998934 ) ) ;
#4436=ADVANCED_FACE ( 'NONE', ( #11232 ), #12267, .F. ) ;
#4437=CARTESIAN_POINT ( 'NONE',  ( -5.935543223013858949, 0.8771126767606857166, 31.00000000000000000 ) ) ;
#4440=CARTESIAN_POINT ( 'NONE',  ( 6.081836621194470105, 1.445163676684702692, 25.37305891554299819 ) ) ;
#4446=CARTESIAN_POINT ( 'NONE',  ( 0.1306171417088810571, 6.000000000000000888, 30.00000000000000000 ) ) ;
#4447=VERTEX_POINT ( 'NONE', #5195 ) ;
#4449=CARTESIAN_POINT ( 'NONE',  ( -0.9740807849835485532, 5.920620690450699719, 11.23850119700668237 ) ) ;
#4450=EDGE_CURVE ( 'NONE', #15268, #12984, #4574, .T. ) ;
#4451=ORIENTED_EDGE ( 'NONE', *, *, #15351, .T. ) ;
#4452=CARTESIAN_POINT ( 'NONE',  ( -4.196038884587126816, -4.289036423669315923, 4.496102049840170700 ) ) ;
#4455=CARTESIAN_POINT ( 'NONE',  ( 3.158296126777706547, 5.394094919772162378, 17.20112161576661691 ) ) ;
#4457=CARTESIAN_POINT ( 'NONE',  ( 5.915755444410836006, -1.003187219519639628, 23.99687951097623184 ) ) ;
#4459=CARTESIAN_POINT ( 'NONE',  ( -6.020865209844600052, -1.681180471732124149, 4.025999019766706155 ) ) ;
#4461=AXIS2_PLACEMENT_3D ( 'NONE', #4242, #11634, #2973 ) ;
#4463=CARTESIAN_POINT ( 'NONE',  ( 4.286401442266577710, -4.198423832313146420, 31.00000000000000000 ) ) ;
#4464=CARTESIAN_POINT ( 'NONE',  ( 5.931793676715092722, 0.9035324301688769655, 11.76239891805594340 ) ) ;
#4465=ORIENTED_EDGE ( 'NONE', *, *, #1472, .F. ) ;
#4466=EDGE_CURVE ( 'NONE', #12035, #11999, #11260, .T. ) ;
#4470=CARTESIAN_POINT ( 'NONE',  ( 5.570760634536763511, 2.834026536768326832, 4.737747182782873878 ) ) ;
#4473=CARTESIAN_POINT ( 'NONE',  ( -5.915653884842702048, -1.003805156977462198, 31.50439760644212939 ) ) ;
#4478=B_SPLINE_CURVE_WITH_KNOTS ( 'NONE', 3,
 ( #7915, #903, #5464, #4577, #11800, #3295, #8158, #5617, #5696, #14111, #595, #830, #14036, #12993, #10387, #2019, #11650, #752 ),
 .UNSPECIFIED., .F., .F.,
 ( 4, 2, 2, 2, 2, 2, 2, 2, 4 ),
 ( 0.003131486019302003303, 0.003522824630466707407, 0.003914163241631411945, 0.004305501852796116483, 0.004696840463960820153, 0.005088179075125524690, 0.005479517686290229228, 0.005870856297454934633, 0.006262194908619640038 ),
 .UNSPECIFIED. ) ;
#4479=CARTESIAN_POINT ( 'NONE',  ( 5.131373506000546314, 7.062729720844130199, 11.49999999999998224 ) ) ;
#4481=CARTESIAN_POINT ( 'NONE',  ( 4.435347140101073116, -4.403429997944470209, 4.867625892836954904 ) ) ;
#4484=EDGE_CURVE ( 'NONE', #5826, #15044, #13204, .T. ) ;
#4485=CARTESIAN_POINT ( 'NONE',  ( 4.435347140100915020, 4.403429997944631857, 18.13237410716304865 ) ) ;
#4487=CARTESIAN_POINT ( 'NONE',  ( 2.668367453516707233, -5.373994336898093138, 5.000000000000004441 ) ) ;
#4489=CARTESIAN_POINT ( 'NONE',  ( -0.2622538972263960821, 6.245673238944477568, 12.47385994369196816 ) ) ;
#4491=CARTESIAN_POINT ( 'NONE',  ( 5.725930890718356814, 2.506952462183982266, 23.70066851092423832 ) ) ;
#4493=CARTESIAN_POINT ( 'NONE',  ( -5.783239563508403513, 1.602707436861190438, 17.02641404563305372 ) ) ;
#4495=FACE_BOUND ( 'NONE', #1430, .T. ) ;
#4498=CARTESIAN_POINT ( 'NONE',  ( -2.692693252389528169, -5.362085866495135633, 31.26382603205595601 ) ) ;
#4499=( LENGTH_UNIT ( ) NAMED_UNIT ( * ) SI_UNIT ( .MILLI., .METRE. ) );
#4500=CARTESIAN_POINT ( 'NONE',  ( 0.000000000000000000, 6.250000000000000888, 32.00000000000000000 ) ) ;
#4503=FACE_OUTER_BOUND ( 'NONE', #12060, .T. ) ;
#4504=CARTESIAN_POINT ( 'NONE',  ( 0.5042675786779833302, 6.230788509548835563, 25.37331068310455251 ) ) ;
#4511=CARTESIAN_POINT ( 'NONE',  ( -5.725684683139587783, 2.507514573674819669, 18.79887838423337598 ) ) ;
#4514=LINE ( 'NONE', #5486, #10877 ) ;
#4520=CARTESIAN_POINT ( 'NONE',  ( -5.842945980534661743, -1.369128644668902384, 5.873784308702619583 ) ) ;
#4522=FACE_BOUND ( 'NONE', #5283, .T. ) ;
#4525=VERTEX_POINT ( 'NONE', #6264 ) ;
#4527=AXIS2_PLACEMENT_3D ( 'NONE', #1741, #6536, #4053 ) ;
#4528=EDGE_CURVE ( 'NONE', #12751, #13870, #11181, .T. ) ;
#4529=DIRECTION ( 'NONE',  ( -0.9510565162951544194, 0.3090169943749447312, 0.000000000000000000 ) ) ;
#4532=ORIENTED_EDGE ( 'NONE', *, *, #13034, .T. ) ;
#4533=B_SPLINE_CURVE_WITH_KNOTS ( 'NONE', 3,
 ( #13076, #13319, #2421, #7289, #2506, #2176, #12125, #6095, #10700, #7362, #1300, #6177, #991, #5855, #11533, #11382, #9092, #3109 ),
 .UNSPECIFIED., .F., .F.,
 ( 4, 2, 2, 2, 2, 2, 2, 2, 4 ),
 ( 0.000000000000000000, 0.0003914904498596253886, 0.0007829808997192507771, 0.001174471349578876112, 0.001565961799438501554, 0.001957452249298126997, 0.002348942699157752223, 0.002740433149017377883, 0.003131923598877003109 ),
 .UNSPECIFIED. ) ;
#4534=CARTESIAN_POINT ( 'NONE',  ( -3.107688324358628407, -5.133887830459884505, 4.126215691297385746 ) ) ;
#4536=CARTESIAN_POINT ( 'NONE',  ( 5.317509234263996021, 2.779225709350927609, 17.86760611998364823 ) ) ;
#4539=CARTESIAN_POINT ( 'NONE',  ( -2.817313151351109379, -5.579000502529471994, 5.000000000000004441 ) ) ;
#4547=EDGE_LOOP ( 'NONE', ( #15309, #13295 ) ) ;
#4548=EDGE_CURVE ( 'NONE', #8273, #1022, #9605, .T. ) ;
#4556=ORIENTED_EDGE ( 'NONE', *, *, #2168, .T. ) ;
#4557=B_SPLINE_CURVE_WITH_KNOTS ( 'NONE', 3,
 ( #13773, #6401, #11233, #10355, #4308, #9170, #3985, #335, #5196, #1757, #6552, #2882, #12502, #7729, #1677, #10204, #9021, #12660 ),
 .UNSPECIFIED., .F., .F.,
 ( 4, 2, 2, 2, 2, 2, 2, 2, 4 ),
 ( 0.000000000000000000, 0.0003914362731607569780, 0.0007828725463215139560, 0.001174308819482270880, 0.001565745092643027912, 0.001957181365803784944, 0.002348617638964541759, 0.002740053912125299009, 0.003131490185286055824 ),
 .UNSPECIFIED. ) ;
#4558=CARTESIAN_POINT ( 'NONE',  ( 4.435347140100928343, -4.403429997944614982, 24.49999999999999289 ) ) ;
#4559=CARTESIAN_POINT ( 'NONE',  ( 2.996417732210394647, 5.485687819087000427, 25.11396179408070850 ) ) ;
#4562=CARTESIAN_POINT ( 'NONE',  ( -4.435347140101218777, 4.403429997944323659, 24.49999999999999289 ) ) ;
#4568=ORIENTED_EDGE ( 'NONE', *, *, #9396, .T. ) ;
#4569=CARTESIAN_POINT ( 'NONE',  ( -5.375605342016444688, 2.665598297262417482, 25.00312048902378237 ) ) ;
#4571=CARTESIAN_POINT ( 'NONE',  ( -5.648794263291700979, 2.676232015153707344, 25.11441947245483064 ) ) ;
#4574=B_SPLINE_CURVE_WITH_KNOTS ( 'NONE', 3,
 ( #6318, #6240, #11155, #257, #13694, #13539, #7500, #2804, #12501, #13464, #14746, #8782, #1600, #1367, #3832, #3856, #2590, #1628 ),
 .UNSPECIFIED., .F., .F.,
 ( 4, 2, 2, 2, 2, 2, 2, 2, 4 ),
 ( 0.000000000000000000, 0.0003914357524127485156, 0.0007828715048254970311, 0.001174307257238245547, 0.001565743009650994062, 0.001957178762063742361, 0.002348614514476491093, 0.002740050266889239826, 0.003131486019301988125 ),
 .UNSPECIFIED. ) ;
#4577=CARTESIAN_POINT ( 'NONE',  ( 2.930600586412910324, 5.520563544161783298, 10.99691356133952169 ) ) ;
#4578=CARTESIAN_POINT ( 'NONE',  ( 5.621197618055753686, -2.101623592078309510, 17.02601979877759319 ) ) ;
#4580=CARTESIAN_POINT ( 'NONE',  ( -3.883588957979267065, -4.898466244118923285, 18.97377282875267923 ) ) ;
#4582=CARTESIAN_POINT ( 'NONE',  ( -3.011385983131315225, -5.190390249166442871, 31.79952054102716374 ) ) ;
#4584=FACE_OUTER_BOUND ( 'NONE', #8867, .T. ) ;
#4585=ADVANCED_FACE ( 'NONE', ( #12450 ), #6426, .F. ) ;
#4588=CARTESIAN_POINT ( 'NONE',  ( -5.558508435838126260, -2.857531096719055697, 18.13063932754212004 ) ) ;
#4590=EDGE_CURVE ( 'NONE', #7332, #5826, #10384, .T. ) ;
#4592=CARTESIAN_POINT ( 'NONE',  ( -4.267838854167155027, 4.217593933790356964, 4.737601081944045056 ) ) ;
#4594=VERTEX_POINT ( 'NONE', #9271 ) ;
#4595=CARTESIAN_POINT ( 'NONE',  ( -5.903061651806585708, 2.057626436184840646, 18.99991741810287493 ) ) ;
#4600=CARTESIAN_POINT ( 'NONE',  ( 5.649200442566227665, 2.675373855294000514, 25.11560192892921606 ) ) ;
#4604=FACE_BOUND ( 'NONE', #9002, .T. ) ;
#4606=CARTESIAN_POINT ( 'NONE',  ( -4.286401442266531525, -4.198423832313195270, 5.000000000000004441 ) ) ;
#4611=ORIENTED_EDGE ( 'NONE', *, *, #9756, .F. ) ;
#4615=CARTESIAN_POINT ( 'NONE',  ( 5.317509234263995133, 2.779225709350928053, 17.99999999999998934 ) ) ;
#4617=CARTESIAN_POINT ( 'NONE',  ( 3.632753594129368047, -4.777047695050953280, 30.00004946353777768 ) ) ;
#4621=CARTESIAN_POINT ( 'NONE',  ( 0.9735954530125449091, -6.173909381473989377, 31.26281793585245694 ) ) ;
#4624=VERTEX_POINT ( 'NONE', #826 ) ;
#4625=VERTEX_POINT ( 'NONE', #11797 ) ;
#4626=VERTEX_POINT ( 'NONE', #3212 ) ;
#4628=CARTESIAN_POINT ( 'NONE',  ( 2.996920846510496172, 5.485395142346785491, 30.38558052754516225 ) ) ;
#4629=CARTESIAN_POINT ( 'NONE',  ( -4.196038884587224516, 4.289036423669218223, 12.00389795015984973 ) ) ;
#4633=CARTESIAN_POINT ( 'NONE',  ( 2.031800924177950305E-13, 6.000000000000000888, 23.49999999999999289 ) ) ;
#4637=ADVANCED_FACE ( 'NONE', ( #7912 ), #10614, .F. ) ;
#4641=DIRECTION ( 'NONE',  ( -0.5877852522924685852, -0.8090169943749507819, 0.000000000000000000 ) ) ;
#4643=B_SPLINE_CURVE_WITH_KNOTS ( 'NONE', 3,
 ( #2633, #11064, #7563, #322, #1588, #1510, #11143, #10037, #7487, #6385, #1275, #6466, #13367, #9730, #12332, #163, #5026, #14568 ),
 .UNSPECIFIED., .F., .F.,
 ( 4, 2, 2, 2, 2, 2, 2, 2, 4 ),
 ( 0.000000000000000000, 0.0003914898357794973326, 0.0007829796715589946651, 0.001174469507338491998, 0.001565959343117989330, 0.001957449178897486663, 0.002348939014676983995, 0.002740428850456481328, 0.003131918686235978661 ),
 .UNSPECIFIED. ) ;
#4647=CARTESIAN_POINT ( 'NONE',  ( 2.668367453516705901, -5.373994336898094915, 4.869350386511452911 ) ) ;
#4648=VERTEX_POINT ( 'NONE', #9193 ) ;
#4649=EDGE_LOOP ( 'NONE', ( #1506, #1330 ) ) ;
#4650=CARTESIAN_POINT ( 'NONE',  ( 0.2637975869347874425, 6.245592211692893692, 31.97332839949191552 ) ) ;
#4652=CARTESIAN_POINT ( 'NONE',  ( 3.922288969639753375, -4.542045818322549167, 17.12621569129736798 ) ) ;
#4653=CARTESIAN_POINT ( 'NONE',  ( 0.9735954530125295880, -6.173909381473990265, 5.262817935852433848 ) ) ;
#4655=CARTESIAN_POINT ( 'NONE',  ( -6.020865209844618704, 1.681180471732060422, 31.97400098023329917 ) ) ;
#4656=EDGE_CURVE ( 'NONE', #8072, #8675, #3062, .T. ) ;
#4657=CARTESIAN_POINT ( 'NONE',  ( 6.123233995736766282E-16, -6.250000000000000888, 6.000000000000005329 ) ) ;
#4658=B_SPLINE_CURVE_WITH_KNOTS ( 'NONE', 3,
 ( #8574, #11440, #9076, #3240, #5567, #15109, #4520, #4364, #10413, #7786, #10564, #11752, #13825, #778, #11516, #9149, #6682, #3013 ),
 .UNSPECIFIED., .F., .F.,
 ( 4, 2, 2, 2, 2, 2, 2, 2, 4 ),
 ( 0.000000000000000000, 0.0003914898357794940800, 0.0007829796715589883768, 0.001174469507338482457, 0.001565959343117977187, 0.001957449178897471484, 0.002348939014676964913, 0.002740428850456459210, 0.003131918686235953507 ),
 .UNSPECIFIED. ) ;
#4659=CARTESIAN_POINT ( 'NONE',  ( -0.9740012993918163442, -6.173846968979670891, 24.76164920628438182 ) ) ;
#4661=CARTESIAN_POINT ( 'NONE',  ( -5.725684683139530051, -2.507514573674952452, 23.70112161576660625 ) ) ;
#4662=CARTESIAN_POINT ( 'NONE',  ( -3.781065399486090328, -4.978303713186380541, 25.49991741810288204 ) ) ;
#4666=CARTESIAN_POINT ( 'NONE',  ( -5.903843691985178666, -2.055287728870804909, 19.00004906876531408 ) ) ;
#4668=VERTEX_POINT ( 'NONE', #9124 ) ;
#4669=CARTESIAN_POINT ( 'NONE',  ( -5.486741141153783197, 2.429871531109751182, 12.29888242247938202 ) ) ;
#4671=CARTESIAN_POINT ( 'NONE',  ( -2.817313151351169775, -5.579000502529442684, 11.49999999999998224 ) ) ;
#4672=ORIENTED_EDGE ( 'NONE', *, *, #8274, .F. ) ;
#4676=CARTESIAN_POINT ( 'NONE',  ( 6.250000000000000888, 7.654042494670958593E-16, 36.00000000000000711 ) ) ;
#4685=FACE_BOUND ( 'NONE', #751, .T. ) ;
#4687=CARTESIAN_POINT ( 'NONE',  ( 1.000079958708160355, 5.916066267613696361, 31.13152738882034143 ) ) ;
#4692=CARTESIAN_POINT ( 'NONE',  ( -4.154121946520892728, -4.670585111242955278, 12.29887838423337953 ) ) ;
#4695=CARTESIAN_POINT ( 'NONE',  ( -3.922672396097006242, -4.541739265057743502, 4.126352953155773662 ) ) ;
#4696=FACE_OUTER_BOUND ( 'NONE', #12094, .T. ) ;
#4697=CARTESIAN_POINT ( 'NONE',  ( -2.849269941562008857, 5.281123252784022171, 31.61519382448851090 ) ) ;
#4698=CARTESIAN_POINT ( 'NONE',  ( 0.1306070469494091113, 6.249999999999999112, 10.49999999999998401 ) ) ;
#4700=CARTESIAN_POINT ( 'NONE',  ( 3.107278289587086739, 5.134157760522114700, 18.87364704684421923 ) ) ;
#4702=CARTESIAN_POINT ( 'NONE',  ( -6.142844459177239536, -1.156093792145200361, 4.384398071070797265 ) ) ;
#4705=CARTESIAN_POINT ( 'NONE',  ( -5.558508435838199091, 2.857531096718913588, 11.36936067245786397 ) ) ;
#4708=EDGE_LOOP ( 'NONE', ( #6912, #13048 ) ) ;
#4709=EDGE_LOOP ( 'NONE', ( #5435, #4132 ) ) ;
#4710=ORIENTED_EDGE ( 'NONE', *, *, #4181, .T. ) ;
#4712=EDGE_LOOP ( 'NONE', ( #8669, #10210, #264, #4313 ) ) ;
#4714=CARTESIAN_POINT ( 'NONE',  ( -5.666074146197994210, -1.978051345703167208, 32.00004932073311892 ) ) ;
#4716=CARTESIAN_POINT ( 'NONE',  ( 5.558508435838199979, 2.857531096718914476, 31.00000000000000000 ) ) ;
#4723=CARTESIAN_POINT ( 'NONE',  ( 3.254737477228057951, -5.337033878705167211, 30.12632671364006143 ) ) ;
#4728=B_SPLINE_CURVE_WITH_KNOTS ( 'NONE', 3,
 ( #1299, #9907, #13476, #6176, #2578, #190, #6415, #14761, #349, #8718, #5213, #6333, #7824, #6721, #5448, #9111, #10142, #13861 ),
 .UNSPECIFIED., .F., .F.,
 ( 4, 2, 2, 2, 2, 2, 2, 2, 4 ),
 ( 0.000000000000000000, 0.0003914898357794969531, 0.0007829796715589939062, 0.001174469507338490913, 0.001565959343117987812, 0.001957449178897484928, 0.002348939014676981827, 0.002740428850456478726, 0.003131918686235975625 ),
 .UNSPECIFIED. ) ;
#4729=DIRECTION ( 'NONE',  ( -0.9510565162951544194, 0.3090169943749447312, 0.000000000000000000 ) ) ;
#4730=VERTEX_POINT ( 'NONE', #5537 ) ;
#4731=ORIENTED_EDGE ( 'NONE', *, *, #11819, .T. ) ;
#4733=CARTESIAN_POINT ( 'NONE',  ( -5.903061651806561727, 2.057626436184907703, 25.49991741810288559 ) ) ;
#4734=CARTESIAN_POINT ( 'NONE',  ( -4.070051655338184915, -4.744673454622407860, 23.62632671364005432 ) ) ;
#4735=CARTESIAN_POINT ( 'NONE',  ( 0.6139731865239909103, -6.220476368274053591, 4.199755456019331312 ) ) ;
#4736=CARTESIAN_POINT ( 'NONE',  ( -5.984595133899166974, -1.806709459528702988, 31.99995078984293428 ) ) ;
#4737=CARTESIAN_POINT ( 'NONE',  ( -0.9737725088282169761, -6.173885267451821868, 4.737357587265639935 ) ) ;
#4740=CARTESIAN_POINT ( 'NONE',  ( 5.620786884546272510, 2.102685372472933967, 30.02641404563307148 ) ) ;
#4745=CARTESIAN_POINT ( 'NONE',  ( -5.859221468178921199, -2.178708437343302329, 18.97408542334169823 ) ) ;
#4746=ADVANCED_FACE ( 'NONE', ( #6890 ), #11723, .F. ) ;
#4747=CARTESIAN_POINT ( 'NONE',  ( 5.330189595673613390, 2.755293208590291254, 31.26382603205596311 ) ) ;
#4749=CARTESIAN_POINT ( 'NONE',  ( -2.692693252389590786, 5.362085866495107211, 4.736173967944048435 ) ) ;
#4750=CARTESIAN_POINT ( 'NONE',  ( -0.9739805876847252852, -5.920636045238177658, 11.76171386814421105 ) ) ;
#4752=ORIENTED_EDGE ( 'NONE', *, *, #4839, .T. ) ;
#4753=CARTESIAN_POINT ( 'NONE',  ( 0.6144377077731991710, 5.969178481556046023, 23.70033966857736019 ) ) ;
#4755=CARTESIAN_POINT ( 'NONE',  ( -3.011385983131415145, 5.190390249166383363, 10.70047945897284158 ) ) ;
#4760=CARTESIAN_POINT ( 'NONE',  ( -3.779082820360676109, 4.979770177899266237, 6.000049068765331839 ) ) ;
#4765=CARTESIAN_POINT ( 'NONE',  ( 5.558508435838253270, 2.857531096718811892, 17.99999999999998934 ) ) ;
#4766=ORIENTED_EDGE ( 'NONE', *, *, #7650, .F. ) ;
#4770=CARTESIAN_POINT ( 'NONE',  ( 5.935543223013876712, 0.8771126767605440522, 24.49999999999999289 ) ) ;
#4773=EDGE_CURVE ( 'NONE', #9142, #11546, #13971, .T. ) ;
#4774=B_SPLINE_CURVE_WITH_KNOTS ( 'NONE', 3,
 ( #8825, #15023, #7540, #1644, #14940, #10168, #6595, #300, #10090, #6281, #7698, #6520, #11354, #10015, #5084, #225, #11430, #1485 ),
 .UNSPECIFIED., .F., .F.,
 ( 4, 2, 2, 2, 2, 2, 2, 2, 4 ),
 ( 0.000000000000000000, 0.0003914357524127488408, 0.0007828715048254976817, 0.001174307257238246631, 0.001565743009650995363, 0.001957178762063744096, 0.002348614514476493262, 0.002740050266889241994, 0.003131486019301990727 ),
 .UNSPECIFIED. ) ;
#4776=CARTESIAN_POINT ( 'NONE',  ( 5.725930890718322175, -2.506952462184060426, 31.79933148907577234 ) ) ;
#4779=CARTESIAN_POINT ( 'NONE',  ( 4.195842658231382138, 4.289229542213252699, 18.50439760644211518 ) ) ;
#4780=CARTESIAN_POINT ( 'NONE',  ( 6.176542424588115310, 0.9554180641285648923, 11.49999999999998224 ) ) ;
#4782=CARTESIAN_POINT ( 'NONE',  ( 5.931828553037973961, -0.9033193133619132897, 31.26194324003147429 ) ) ;
#4784=CARTESIAN_POINT ( 'NONE',  ( 2.094888799673178700E-14, -6.250000000000000888, 30.00000000000000000 ) ) ;
#4785=CARTESIAN_POINT ( 'NONE',  ( -5.648559266344529206, 2.676764518775933244, 10.88603820591927374 ) ) ;
#4786=CARTESIAN_POINT ( 'NONE',  ( 5.375913338529092478, 2.664979843780434621, 12.00428920362018737 ) ) ;
#4787=VECTOR ( 'NONE', #2547, 1000.000000000000114 ) ;
#4792=ORIENTED_EDGE ( 'NONE', *, *, #11, .F. ) ;
#4796=AXIS2_PLACEMENT_3D ( 'NONE', #854, #15419, #6761 ) ;
#4797=CARTESIAN_POINT ( 'NONE',  ( -5.570722351696229424, -2.834100162822036140, 11.76190213084010416 ) ) ;
#4806=VERTEX_POINT ( 'NONE', #12412 ) ;
#4808=ORIENTED_EDGE ( 'NONE', *, *, #13918, .F. ) ;
#4814=CARTESIAN_POINT ( 'NONE',  ( 0.8002720181890988771, -6.199262377003406321, 4.386062624655575171 ) ) ;
#4815=CARTESIAN_POINT ( 'NONE',  ( -5.769755079862325609, 2.405651898698959901, 31.87305891554300530 ) ) ;
#4816=B_SPLINE_CURVE_WITH_KNOTS ( 'NONE', 3,
 ( #4418, #6891, #8156, #9126, #10538, #4491, #9272, #13955, #3064, #11568, #14109, #6735, #663, #10385, #15236, #9345, #12118, #10849 ),
 .UNSPECIFIED., .F., .F.,
 ( 4, 2, 2, 2, 2, 2, 2, 2, 4 ),
 ( 0.000000000000000000, 0.0003914357524127467266, 0.0007828715048254934533, 0.001174307257238240126, 0.001565743009650986907, 0.001957178762063733687, 0.002348614514476480251, 0.002740050266889227249, 0.003131486019301973813 ),
 .UNSPECIFIED. ) ;
#4822=CARTESIAN_POINT ( 'NONE',  ( -7.490007020835699691, -2.433650805992386701, 31.00000000000000000 ) ) ;
#4826=CARTESIAN_POINT ( 'NONE',  ( 4.286401442266518202, 4.198423832313208592, 31.00000000000000000 ) ) ;
#4830=CARTESIAN_POINT ( 'NONE',  ( -0.2624013748572519011, -5.995472630654522739, 10.52628559691080845 ) ) ;
#4832=EDGE_LOOP ( 'NONE', ( #14397, #8805, #12177, #14063 ) ) ;
#4834=FACE_OUTER_BOUND ( 'NONE', #7038, .T. ) ;
#4835=ORIENTED_EDGE ( 'NONE', *, *, #6051, .F. ) ;
#4836=CARTESIAN_POINT ( 'NONE',  ( 2.996920846510343406, 5.485395142346868980, 23.88558052754514804 ) ) ;
#4839=EDGE_CURVE ( 'NONE', #8675, #5801, #8468, .T. ) ;
#4842=CARTESIAN_POINT ( 'NONE',  ( -0.2637975869347698454, -6.245592211692896356, 31.97332839949191552 ) ) ;
#4848=DIRECTION ( 'NONE',  ( 0.000000000000000000, 1.000000000000000000, 0.000000000000000000 ) ) ;
#4853=LINE ( 'NONE', #6045, #14693 ) ;
#4854=ORIENTED_EDGE ( 'NONE', *, *, #11938, .F. ) ;
#4856=B_SPLINE_CURVE_WITH_KNOTS ( 'NONE', 3,
 ( #8714, #9980, #2575, #7432, #1534, #2815, #3916, #1376, #12511, #3841, #6250, #1451, #5129, #266, #5050, #14831, #1611, #12588 ),
 .UNSPECIFIED., .F., .F.,
 ( 4, 2, 2, 2, 2, 2, 2, 2, 4 ),
 ( 0.003131918686235974757, 0.003523310662250265027, 0.003914702638264554863, 0.004306094614278844698, 0.004697486590293135401, 0.005088878566307425237, 0.005480270542321715940, 0.005871662518336005776, 0.006263054494350295612 ),
 .UNSPECIFIED. ) ;
#4857=CARTESIAN_POINT ( 'NONE',  ( 5.665824935993609479, -1.978765057080921208, 5.999950536462232087 ) ) ;
#4860=CARTESIAN_POINT ( 'NONE',  ( 6.768587589771821120E-14, -6.250000000000000888, 12.49999999999998401 ) ) ;
#4861=CARTESIAN_POINT ( 'NONE',  ( 4.286401442266437378, 4.198423832313292081, 17.99999999999998934 ) ) ;
#4865=CARTESIAN_POINT ( 'NONE',  ( 1.353717517954364224E-13, -6.250000000000000888, 18.99999999999998934 ) ) ;
#4866=CARTESIAN_POINT ( 'NONE',  ( 5.931828553037959750, 0.9033193133620174287, 4.738056759968539922 ) ) ;
#4867=CARTESIAN_POINT ( 'NONE',  ( -5.746837578676019298, 1.729433780394205700, 30.00004946353777413 ) ) ;
#4868=ORIENTED_EDGE ( 'NONE', *, *, #1127, .F. ) ;
#4871=B_SPLINE_CURVE_WITH_KNOTS ( 'NONE', 3,
 ( #3702, #7373, #4830, #1311, #2187, #10789, #9840, #1002, #6109, #9686, #4750, #14525, #14356, #8331, #13169, #3625, #2432, #1238 ),
 .UNSPECIFIED., .F., .F.,
 ( 4, 2, 2, 2, 2, 2, 2, 2, 4 ),
 ( 0.003131923598876997904, 0.003523316383094314812, 0.003914709167311631287, 0.004306101951528948195, 0.004697494735746265103, 0.005088887519963581144, 0.005480280304180898052, 0.005871673088398214960, 0.006263065872615531868 ),
 .UNSPECIFIED. ) ;
#4874=AXIS2_PLACEMENT_3D ( 'NONE', #7605, #2835, #2988 ) ;
#4881=CARTESIAN_POINT ( 'NONE',  ( 4.195842658231482503, 4.289229542213157664, 5.504397606442132052 ) ) ;
#4883=ADVANCED_FACE ( 'NONE', ( #7281 ), #6088, .F. ) ;
#4884=CARTESIAN_POINT ( 'NONE',  ( 4.153663429050823197, -4.670992970568335068, 30.20066851092421700 ) ) ;
#4886=CARTESIAN_POINT ( 'NONE',  ( 6.021135683317679899, 1.680226122398283950, 5.973772828752684561 ) ) ;
#4887=ORIENTED_EDGE ( 'NONE', *, *, #8312, .F. ) ;
#4890=EDGE_LOOP ( 'NONE', ( #12376, #935 ) ) ;
#4891=ORIENTED_EDGE ( 'NONE', *, *, #2586, .T. ) ;
#4892=ORIENTED_EDGE ( 'NONE', *, *, #4101, .T. ) ;
#4893=CARTESIAN_POINT ( 'NONE',  ( 0.9740012993920327267, 6.173846968979637140, 31.26164920628441024 ) ) ;
#4895=CARTESIAN_POINT ( 'NONE',  ( 0.5043776560897352823, -6.230795654995838539, 5.873374762960125395 ) ) ;
#4897=B_SPLINE_CURVE_WITH_KNOTS ( 'NONE', 3,
 ( #7971, #3270, #5438, #1994, #7814, #13851, #6712, #10285, #7895, #11624, #6868, #10208, #12812, #10440, #4233, #9101, #9026, #10360 ),
 .UNSPECIFIED., .F., .F.,
 ( 4, 2, 2, 2, 2, 2, 2, 2, 4 ),
 ( 0.003131486019301974247, 0.003522824630466683121, 0.003914163241631391996, 0.004305501852796101737, 0.004696840463960810612, 0.005088179075125519486, 0.005479517686290229228, 0.005870856297454939837, 0.006262194908619649579 ),
 .UNSPECIFIED. ) ;
#4899=CARTESIAN_POINT ( 'NONE',  ( -3.011385983131359190, -5.190390249166418002, 12.29952054102714598 ) ) ;
#4900=AXIS2_PLACEMENT_3D ( 'NONE', #3938, #14697, #5073 ) ;
#4901=CARTESIAN_POINT ( 'NONE',  ( -5.903061651806636334, 2.057626436184698537, 5.999917418102894473 ) ) ;
#4902=CARTESIAN_POINT ( 'NONE',  ( 2.817313151351065859, -5.579000502529494199, 17.99999999999998934 ) ) ;
#4903=DIRECTION ( 'NONE',  ( 0.000000000000000000, 0.000000000000000000, -1.000000000000000000 ) ) ;
#4907=CARTESIAN_POINT ( 'NONE',  ( 5.409274167810647072, 2.597759609440661421, 10.88480617551147667 ) ) ;
#4912=CARTESIAN_POINT ( 'NONE',  ( 0.2622916576877225014, -5.995491482261829042, 12.47384942646812078 ) ) ;
#4914=CARTESIAN_POINT ( 'NONE',  ( 4.435347140101058905, -4.403429997944484420, 31.00000000000000000 ) ) ;
#4916=CARTESIAN_POINT ( 'NONE',  ( -4.006441409774768481, 4.467329318258185467, 10.70111757752057002 ) ) ;
#4919=CARTESIAN_POINT ( 'NONE',  ( 2.031800923730693940E-13, -6.250000000000000888, 23.49999999999999289 ) ) ;
#4920=AXIS2_PLACEMENT_3D ( 'NONE', #12576, #4224, #10124 ) ;
#4921=CARTESIAN_POINT ( 'NONE',  ( -0.1306070469493167963, -6.250000000000002665, 30.00000000000000000 ) ) ;
#4923=FACE_BOUND ( 'NONE', #2983, .T. ) ;
#4926=CARTESIAN_POINT ( 'NONE',  ( 5.558508435838323436, -2.857531096718671559, 24.63237410716305931 ) ) ;
#4930=CARTESIAN_POINT ( 'NONE',  ( -7.490007020835699691, -2.433650805992386701, 31.00000000000000000 ) ) ;
#4931=CARTESIAN_POINT ( 'NONE',  ( 3.780072143464197065, 4.979057943639763728, 29.99991780678444186 ) ) ;
#4934=ADVANCED_FACE ( 'NONE', ( #9751 ), #1744, .F. ) ;
#4936=CARTESIAN_POINT ( 'NONE',  ( 5.531796221294873028, -2.326749136277222796, 5.873784308702619583 ) ) ;
#4939=CARTESIAN_POINT ( 'NONE',  ( -0.7988860301921629770, -6.199427171881343845, 10.88455580536193601 ) ) ;
#4940=CARTESIAN_POINT ( 'NONE',  ( 3.312524433819871827, -5.004191858253940417, 30.02591947216899371 ) ) ;
#4942=CARTESIAN_POINT ( 'NONE',  ( 7.799024015210631156, -1.482594289697088730, 5.000000000000004441 ) ) ;
#4944=CARTESIAN_POINT ( 'NONE',  ( 5.746619684944286099, -1.730157667110801212, 32.00004932073311892 ) ) ;
#4945=CARTESIAN_POINT ( 'NONE',  ( -5.666074146198012862, 1.978051345703121244, 10.49995067926686332 ) ) ;
#4946=CARTESIAN_POINT ( 'NONE',  ( 5.903347812666339678, 1.076697810262650323, 4.386022610569179747 ) ) ;
#4947=CARTESIAN_POINT ( 'NONE',  ( 2.668367453516445664, 5.373994336898223700, 24.36938304467862082 ) ) ;
#4948=EDGE_CURVE ( 'NONE', #15526, #5163, #11221, .T. ) ;
#4949=ORIENTED_EDGE ( 'NONE', *, *, #13803, .T. ) ;
#4954=CARTESIAN_POINT ( 'NONE',  ( -4.286401442266607020, 4.198423832313117110, 31.00000000000000000 ) ) ;
#4955=ORIENTED_EDGE ( 'NONE', *, *, #5899, .F. ) ;
#4958=CARTESIAN_POINT ( 'NONE',  ( -6.155867707731093930, -1.081837891425983189, 12.00436969680152899 ) ) ;
#4962=CARTESIAN_POINT ( 'NONE',  ( -5.409007216690699948, 2.598315788643695612, 31.61442521571937547 ) ) ;
#4963=CARTESIAN_POINT ( 'NONE',  ( 4.286401442266577710, -4.198423832313146420, 31.00000000000000000 ) ) ;
#4966=CARTESIAN_POINT ( 'NONE',  ( 2.996417732210637563, -5.485687819086870753, 30.38603820591928084 ) ) ;
#4968=CARTESIAN_POINT ( 'NONE',  ( 5.985119669071089277, 1.805077827356658116, 5.999917418102894473 ) ) ;
#4971=EDGE_LOOP ( 'NONE', ( #3659, #4338, #6283, #11005 ) ) ;
#4974=CARTESIAN_POINT ( 'NONE',  ( 0.6151877315909851651, -6.220340188096018075, 5.799066734696703307 ) ) ;
#4976=CARTESIAN_POINT ( 'NONE',  ( 4.005785023174466275, -4.467917056767390704, 12.29952054102713532 ) ) ;
#4977=CARTESIAN_POINT ( 'NONE',  ( 4.416779112813571828, -4.422345839825880809, 24.23774718278286855 ) ) ;
#4978=DIRECTION ( 'NONE',  ( 0.000000000000000000, 1.000000000000000000, 0.000000000000000000 ) ) ;
#4979=CARTESIAN_POINT ( 'NONE',  ( -3.781065399486036149, 4.978303713186424062, 10.50008258189709132 ) ) ;
#4987=ORIENTED_EDGE ( 'NONE', *, *, #8342, .T. ) ;
#4988=CARTESIAN_POINT ( 'NONE',  ( -5.931734679891446760, 0.9039278060244116952, 11.76382603205595956 ) ) ;
#4989=FACE_OUTER_BOUND ( 'NONE', #10106, .T. ) ;
#4991=CARTESIAN_POINT ( 'NONE',  ( 4.344265632482167128, -4.493596842504882005, 31.50425949503009448 ) ) ;
#4993=ADVANCED_FACE ( 'NONE', ( #554 ), #397, .F. ) ;
#4994=CARTESIAN_POINT ( 'NONE',  ( 7.180990026460783326, -3.384707322287269893, 17.99999999999998934 ) ) ;
#4996=CARTESIAN_POINT ( 'NONE',  ( -3.159082487394956118, 5.393634094348230157, 23.70045537531157365 ) ) ;
#4997=CARTESIAN_POINT ( 'NONE',  ( -5.558508435838198203, 2.857531096718914032, 11.63060690723495760 ) ) ;
#4999=FACE_BOUND ( 'NONE', #13681, .T. ) ;
#5006=CARTESIAN_POINT ( 'NONE',  ( -2.997753866155795421, -5.484939622623858924, 12.11560192892921251 ) ) ;
#5008=VERTEX_POINT ( 'NONE', #10191 ) ;
#5011=DIRECTION ( 'NONE',  ( 0.5877852522924802425, -0.8090169943749422332, 0.000000000000000000 ) ) ;
#5012=VECTOR ( 'NONE', #2121, 1000.000000000000114 ) ;
#5015=CARTESIAN_POINT ( 'NONE',  ( 3.633127580202159201, 4.776802569231145768, 16.99992038825522656 ) ) ;
#5017=CARTESIAN_POINT ( 'NONE',  ( -0.8738118504725461699, -5.936246475285035018, 31.50357242174242600 ) ) ;
#5018=CARTESIAN_POINT ( 'NONE',  ( 5.915699123067170717, -1.003533581835479582, 31.50389795015983552 ) ) ;
#5019=CARTESIAN_POINT ( 'NONE',  ( -3.567258970015989128, 5.133675764669665575, 29.99991780678443121 ) ) ;
#5020=CARTESIAN_POINT ( 'NONE',  ( -5.931817299736859894, 0.9033986943601567399, 30.73770962164068621 ) ) ;
#5023=EDGE_LOOP ( 'NONE', ( #1993, #9158 ) ) ;
#5025=EDGE_LOOP ( 'NONE', ( #13522, #5572 ) ) ;
#5026=CARTESIAN_POINT ( 'NONE',  ( -5.317509234263835260, -2.779225709351231366, 24.63064961348855775 ) ) ;
#5031=CYLINDRICAL_SURFACE ( 'NONE', #15305, 1.000000000000000666 ) ;
#5034=VECTOR ( 'NONE', #4125, 1000.000000000000000 ) ;
#5035=CARTESIAN_POINT ( 'NONE',  ( -5.317509234263962270, 2.779225709350992890, 31.13061695532139339 ) ) ;
#5036=ADVANCED_FACE ( 'NONE', ( #8117 ), #1978, .F. ) ;
#5038=CARTESIAN_POINT ( 'NONE',  ( 2.668367453516629517, 5.373994336898132218, 5.000000000000004441 ) ) ;
#5040=FACE_OUTER_BOUND ( 'NONE', #2809, .T. ) ;
#5042=EDGE_CURVE ( 'NONE', #5984, #9644, #14323, .T. ) ;
#5045=ADVANCED_FACE ( 'NONE', ( #10574 ), #2131, .F. ) ;
#5046=ORIENTED_EDGE ( 'NONE', *, *, #3851, .F. ) ;
#5047=CARTESIAN_POINT ( 'NONE',  ( 0.9737778612006920964, 5.920671847850494274, 17.73736375884652716 ) ) ;
#5048=CARTESIAN_POINT ( 'NONE',  ( 2.841163418881393454, 5.567120626447931819, 4.737630265561252330 ) ) ;
#5049=CARTESIAN_POINT ( 'NONE',  ( -6.081509788407712058, -1.446521464462831918, 17.12618035954928075 ) ) ;
#5050=CARTESIAN_POINT ( 'NONE',  ( -2.782769401326246062, -5.315896561274812804, 18.50428920362019269 ) ) ;
#5052=CARTESIAN_POINT ( 'NONE',  ( -0.5042675786777256475, -6.230788509548854215, 25.37331068310447080 ) ) ;
#5053=CARTESIAN_POINT ( 'NONE',  ( -3.883588957979273726, 4.898466244118916180, 10.52622717124729412 ) ) ;
#5054=CARTESIAN_POINT ( 'NONE',  ( -2.817313151351311884, 5.579000502529370742, 17.99999999999998934 ) ) ;
#5059=AXIS2_PLACEMENT_3D ( 'NONE', #5117, #11311, #6477 ) ;
#5062=ORIENTED_EDGE ( 'NONE', *, *, #10429, .F. ) ;
#5063=DIRECTION ( 'NONE',  ( 0.9510565162951499785, 0.3090169943749582204, 0.000000000000000000 ) ) ;
#5065=CARTESIAN_POINT ( 'NONE',  ( 3.779681992289830372, -4.979315417303873836, 10.50004921015705150 ) ) ;
#5066=AXIS2_PLACEMENT_3D ( 'NONE', #7954, #9008, #15042 ) ;
#5067=CARTESIAN_POINT ( 'NONE',  ( -3.011385983131546595, 5.190390249166308756, 23.70047945897283270 ) ) ;
#5068=FACE_OUTER_BOUND ( 'NONE', #10463, .T. ) ;
#5070=CARTESIAN_POINT ( 'NONE',  ( 3.253823204784968226, 5.337590213880594625, 23.62694108445698760 ) ) ;
#5073=DIRECTION ( 'NONE',  ( -0.3090169943749446202, -0.9510565162951544194, 0.000000000000000000 ) ) ;
#5080=CARTESIAN_POINT ( 'NONE',  ( -3.779082820360647244, -4.979770177899287553, 10.49995093123465395 ) ) ;
#5082=CARTESIAN_POINT ( 'NONE',  ( 6.123233995736766282E-16, -6.250000000000000888, 6.000000000000004441 ) ) ;
#5084=CARTESIAN_POINT ( 'NONE',  ( 6.155912734541153952, -1.081577393120774166, 18.50389213124969956 ) ) ;
#5086=EDGE_LOOP ( 'NONE', ( #1056, #5326, #9418, #11292 ) ) ;
#5087=CARTESIAN_POINT ( 'NONE',  ( -4.005361199355111701, -4.468319061418669413, 23.69977782616122397 ) ) ;
#5088=MECHANICAL_DESIGN_GEOMETRIC_PRESENTATION_REPRESENTATION('',(#3804),#10931);
#5091=B_SPLINE_CURVE_WITH_KNOTS ( 'NONE', 3,
 ( #14011, #13931, #11703, #11543, #11394, #643, #5514, #4396, #9250, #14084, #8052, #12890, #5670, #1334, #10671, #11848, #13434, #10968 ),
 .UNSPECIFIED., .F., .F.,
 ( 4, 2, 2, 2, 2, 2, 2, 2, 4 ),
 ( 0.003131918686235979962, 0.003523310662250269364, 0.003914702638264559199, 0.004306094614278848168, 0.004697486590293138004, 0.005088878566307427839, 0.005480270542321717675, 0.005871662518336009245, 0.006263054494350299081 ),
 .UNSPECIFIED. ) ;
#5093=CARTESIAN_POINT ( 'NONE',  ( -0.6144300524833031796, -6.220417338033058741, 10.70033372175932662 ) ) ;
#5096=CARTESIAN_POINT ( 'NONE',  ( 2.094888798833199608E-14, -6.000000000000000888, 30.00000000000000000 ) ) ;
#5097=CARTESIAN_POINT ( 'NONE',  ( 4.141923667210722471, -4.342011609040392628, 5.615617326986045654 ) ) ;
#5098=CARTESIAN_POINT ( 'NONE',  ( -1.000082492230581765, -6.169467968613729703, 18.13152538105390832 ) ) ;
#5099=CARTESIAN_POINT ( 'NONE',  ( -5.931817299736839466, -0.9033986943602941855, 11.76229037835932800 ) ) ;
#5100=LINE ( 'NONE', #7407, #14564 ) ;
#5107=ORIENTED_EDGE ( 'NONE', *, *, #10989, .F. ) ;
#5109=CARTESIAN_POINT ( 'NONE',  ( 5.726049995854488373, 2.506679546901831035, 18.79954462468841925 ) ) ;
#5113=B_SPLINE_CURVE_WITH_KNOTS ( 'NONE', 3,
 ( #8876, #12589, #14908, #1922, #2816, #3999, #10214, #6564, #576, #647, #7665, #1767, #11472, #12513, #420, #13937, #2893, #10139 ),
 .UNSPECIFIED., .F., .F.,
 ( 4, 2, 2, 2, 2, 2, 2, 2, 4 ),
 ( 0.000000000000000000, 0.0003914362731607440218, 0.0007828725463214880435, 0.001174308819482232065, 0.001565745092642976087, 0.001957181365803720326, 0.002348617638964464131, 0.002740053912125207936, 0.003131490185285952174 ),
 .UNSPECIFIED. ) ;
#5115=CARTESIAN_POINT ( 'NONE',  ( 4.142173849413761211, 4.341773579105392855, 5.615193824488510010 ) ) ;
#5117=CARTESIAN_POINT ( 'NONE',  ( -7.490007020835664164, -2.433650805992495503, 17.99999999999998934 ) ) ;
#5119=ORIENTED_EDGE ( 'NONE', *, *, #9140, .F. ) ;
#5121=VERTEX_POINT ( 'NONE', #13033 ) ;
#5123=CARTESIAN_POINT ( 'NONE',  ( 0.2624013748574551275, 5.995472630654512969, 17.02628559691081733 ) ) ;
#5125=ADVANCED_FACE ( 'NONE', ( #9384 ), #11606, .F. ) ;
#5127=CARTESIAN_POINT ( 'NONE',  ( 0.5042675786779255986, 6.230788509548840004, 5.873310683104476126 ) ) ;
#5129=CARTESIAN_POINT ( 'NONE',  ( -3.011385983131411592, -5.190390249166387804, 18.79952054102714598 ) ) ;
#5130=CARTESIAN_POINT ( 'NONE',  ( 2.817313151351004130, -5.579000502529524397, 24.49999999999999289 ) ) ;
#5133=CARTESIAN_POINT ( 'NONE',  ( -2.817313151351250156, 5.579000502529400940, 11.36765874365829099 ) ) ;
#5134=CARTESIAN_POINT ( 'NONE',  ( -3.458467055437393078, 5.207305717053763772, 18.97359571723300320 ) ) ;
#5135=PRODUCT_CONTEXT ( 'NONE', #12368, 'mechanical' ) ;
#5141=ORIENTED_EDGE ( 'NONE', *, *, #6602, .T. ) ;
#5142=CARTESIAN_POINT ( 'NONE',  ( -6.176542424588100211, 0.9554180641286806885, 17.99999999999998934 ) ) ;
#5145=CARTESIAN_POINT ( 'NONE',  ( 0.7993401192312425962, -6.199366368793653770, 12.11483246936573721 ) ) ;
#5150=CARTESIAN_POINT ( 'NONE',  ( -2.997753866155991265, 5.484939622623749678, 23.88439807107078039 ) ) ;
#5152=CARTESIAN_POINT ( 'NONE',  ( 5.747343991580163625, 1.727858744772343247, 5.999920023562623328 ) ) ;
#5158=CARTESIAN_POINT ( 'NONE',  ( -3.255128505894268276, -5.336774832660745815, 10.62619944752603018 ) ) ;
#5161=CARTESIAN_POINT ( 'NONE',  ( -4.196038884587275142, 4.289036423669169373, 18.50389795015985328 ) ) ;
#5163=VERTEX_POINT ( 'NONE', #12871 ) ;
#5164=LINE ( 'NONE', #6677, #7 ) ;
#5165=CARTESIAN_POINT ( 'NONE',  ( 5.935543223013858949, -0.8771126767606638452, 5.000000000000004441 ) ) ;
#5166=EDGE_CURVE ( 'NONE', #8072, #11236, #305, .T. ) ;
#5167=CARTESIAN_POINT ( 'NONE',  ( -5.317509234263969375, 2.779225709350973350, 5.000000000000004441 ) ) ;
#5169=CARTESIAN_POINT ( 'NONE',  ( 4.005785023174365023, 4.467917056767481299, 17.20047945897285047 ) ) ;
#5172=ADVANCED_FACE ( 'NONE', ( #7241 ), #145, .F. ) ;
#5175=CARTESIAN_POINT ( 'NONE',  ( -5.935543223013836744, -0.8771126767608161678, 11.49999999999998224 ) ) ;
#5176=CYLINDRICAL_SURFACE ( 'NONE', #14841, 1.000000000000000888 ) ;
#5177=EDGE_LOOP ( 'NONE', ( #8765, #4731, #548, #8293 ) ) ;
#5180=CARTESIAN_POINT ( 'NONE',  ( -5.842988226680536634, 1.369004370660818370, 25.37380682714709579 ) ) ;
#5183=CARTESIAN_POINT ( 'NONE',  ( -2.849269941562166952, 5.281123252783936906, 25.11519382448850379 ) ) ;
#5184=ORIENTED_EDGE ( 'NONE', *, *, #15661, .T. ) ;
#5186=CARTESIAN_POINT ( 'NONE',  ( -3.459447313391850631, 5.206669755180985071, 4.025999019766706155 ) ) ;
#5193=CARTESIAN_POINT ( 'NONE',  ( -5.131373506000769247, 7.062729720843990755, 11.49999999999998224 ) ) ;
#5195=CARTESIAN_POINT ( 'NONE',  ( 2.668367453516629517, 5.373994336898132218, 5.000000000000004441 ) ) ;
#5196=CARTESIAN_POINT ( 'NONE',  ( -0.9999505860953201708, 6.169489349035809589, 31.13105903165810773 ) ) ;
#5198=B_SPLINE_CURVE_WITH_KNOTS ( 'NONE', 3,
 ( #2802, #14819, #2645, #4881, #5115, #13462, #12421, #9815, #10997, #97, #12264, #7497, #3674, #3752, #11230, #332, #174, #5038 ),
 .UNSPECIFIED., .F., .F.,
 ( 4, 2, 2, 2, 2, 2, 2, 2, 4 ),
 ( 0.000000000000000000, 0.0003914898357794947847, 0.0007829796715589895694, 0.001174469507338484191, 0.001565959343117978055, 0.001957449178897471918, 0.002348939014676965781, 0.002740428850456459644, 0.003131918686235953941 ),
 .UNSPECIFIED. ) ;
#5200=ORIENTED_EDGE ( 'NONE', *, *, #2307, .F. ) ;
#5201=CARTESIAN_POINT ( 'NONE',  ( 0.1323602877613519191, 6.000000000000000000, 18.99999999999998579 ) ) ;
#5202=CARTESIAN_POINT ( 'NONE',  ( 4.344265632482118278, 4.493596842504927302, 4.495740504969913509 ) ) ;
#5203=ORIENTED_EDGE ( 'NONE', *, *, #5922, .F. ) ;
#5204=CARTESIAN_POINT ( 'NONE',  ( -6.176542424588101987, -0.9554180641286524889, 31.00000000000000000 ) ) ;
#5206=CARTESIAN_POINT ( 'NONE',  ( 0.6139908388541118756, -5.969238533166610239, 30.19977627912011542 ) ) ;
#5207=VECTOR ( 'NONE', #14931, 1000.000000000000114 ) ;
#5208=EDGE_CURVE ( 'NONE', #4525, #7295, #7163, .T. ) ;
#5209=CARTESIAN_POINT ( 'NONE',  ( -4.152999119458018029, 4.671604476854316346, 31.80026515017674882 ) ) ;
#5210=CARTESIAN_POINT ( 'NONE',  ( 0.9737725088283790686, 6.173885267451797887, 17.73735758726570566 ) ) ;
#5213=CARTESIAN_POINT ( 'NONE',  ( 5.782895619916185836, -1.604017620857976167, 12.47408052783098853 ) ) ;
#5215=CARTESIAN_POINT ( 'NONE',  ( -4.344502777243645752, 4.493369211529153695, 18.50389213124969956 ) ) ;
#5225=CARTESIAN_POINT ( 'NONE',  ( -6.155867707731101035, 1.081837891425948550, 17.49563030319846746 ) ) ;
#5227=CARTESIAN_POINT ( 'NONE',  ( -0.8738043859790733947, 6.188821459035875883, 5.503415602237494042 ) ) ;
#5228=CARTESIAN_POINT ( 'NONE',  ( 6.172651332693083859, 0.9815532474594386159, 30.73809786915987630 ) ) ;
#5231=CARTESIAN_POINT ( 'NONE',  ( -3.567258970015910080, -5.133675764669719754, 32.00008219321556169 ) ) ;
#5233=CARTESIAN_POINT ( 'NONE',  ( 4.267558728637196097, 4.217879122113799895, 4.736173967944048435 ) ) ;
#5235=CARTESIAN_POINT ( 'NONE',  ( 7.180990026460762010, -3.384707322287334286, 11.49999999999998224 ) ) ;
#5237=FACE_BOUND ( 'NONE', #6967, .T. ) ;
#5241=CARTESIAN_POINT ( 'NONE',  ( 6.172651332693125603, -0.9815532474591706080, 24.76190213084012726 ) ) ;
#5244=CARTESIAN_POINT ( 'NONE',  ( 5.940390500375443139, 6.474944468551700361, 17.99999999999998934 ) ) ;
#5248=CARTESIAN_POINT ( 'NONE',  ( -3.158825713737554164, -5.393784879207130345, 17.20066851092422411 ) ) ;
#5249=CARTESIAN_POINT ( 'NONE',  ( 6.105747081304188306, -1.338335777572190466, 12.30026515017674882 ) ) ;
#5251=DIRECTION ( 'NONE',  ( -0.5877852522924685852, -0.8090169943749507819, 0.000000000000000000 ) ) ;
#5252=CARTESIAN_POINT ( 'NONE',  ( 2.668367453516444776, 5.373994336898222812, 24.49999999999999289 ) ) ;
#5255=CARTESIAN_POINT ( 'NONE',  ( 2.782156709077490131, -5.316215864844006767, 5.503120489023789474 ) ) ;
#5256=CARTESIAN_POINT ( 'NONE',  ( -3.634089073485446963, 4.776071126502678510, 30.00007997643739088 ) ) ;
#5261=ADVANCED_FACE ( 'NONE', ( #12312 ), #1410, .F. ) ;
#5262=ORIENTED_EDGE ( 'NONE', *, *, #12407, .F. ) ;
#5270=CARTESIAN_POINT ( 'NONE',  ( -0.8736516769105580060, 5.936271176698252106, 17.49606771578676145 ) ) ;
#5278=DIRECTION ( 'NONE',  ( 0.000000000000000000, 0.000000000000000000, 1.000000000000000000 ) ) ;
#5279=CARTESIAN_POINT ( 'NONE',  ( 3.922288969639730727, 4.542045818322569595, 12.37378430870260715 ) ) ;
#5282=EDGE_CURVE ( 'NONE', #13328, #8099, #14748, .T. ) ;
#5283=EDGE_LOOP ( 'NONE', ( #14465, #14145 ) ) ;
#5284=ORIENTED_EDGE ( 'NONE', *, *, #474, .F. ) ;
#5285=CARTESIAN_POINT ( 'NONE',  ( 0.9999196734184028212, 5.916093360767494147, 17.86725955955069622 ) ) ;
#5287=ORIENTED_EDGE ( 'NONE', *, *, #1564, .F. ) ;
#5288=ORIENTED_EDGE ( 'NONE', *, *, #1535, .F. ) ;
#5289=CARTESIAN_POINT ( 'NONE',  ( -5.615811513734942473, -2.743665920700590011, 17.49691356133953590 ) ) ;
#5290=CARTESIAN_POINT ( 'NONE',  ( 0.8738043859791964074, -6.188821459035860784, 18.50341560223750648 ) ) ;
#5292=CARTESIAN_POINT ( 'NONE',  ( -4.435347140101089103, 4.403429997944455110, 31.00000000000000000 ) ) ;
#5293=CARTESIAN_POINT ( 'NONE',  ( 5.616116467183648098, -2.743044348085566408, 30.49574050496988775 ) ) ;
#5296=CARTESIAN_POINT ( 'NONE',  ( 2.030576276931546336E-13, -6.250000000000000888, 25.49999999999999645 ) ) ;
#5301=VECTOR ( 'NONE', #62, 1000.000000000000114 ) ;
#5302=VERTEX_POINT ( 'NONE', #13745 ) ;
#5306=ORIENTED_EDGE ( 'NONE', *, *, #586, .F. ) ;
#5307=DIRECTION ( 'NONE',  ( 0.000000000000000000, 0.000000000000000000, 1.000000000000000000 ) ) ;
#5308=CARTESIAN_POINT ( 'NONE',  ( -5.770167736194656172, 2.404664418229267575, 23.62632671364006853 ) ) ;
#5309=CARTESIAN_POINT ( 'NONE',  ( 4.435347140100977192, -4.403429997944567020, 17.99999999999998934 ) ) ;
#5310=CARTESIAN_POINT ( 'NONE',  ( 6.081836621194437242, 1.445163676684838361, 12.37305891554298931 ) ) ;
#5313=FACE_BOUND ( 'NONE', #9154, .T. ) ;
#5316=CARTESIAN_POINT ( 'NONE',  ( -3.779082820360620598, -4.979770177899308869, 29.99995093123466816 ) ) ;
#5319=CARTESIAN_POINT ( 'NONE',  ( -2.817313151351206635, 5.579000502529421368, 31.00000000000000000 ) ) ;
#5320=CARTESIAN_POINT ( 'NONE',  ( 4.435347140100959429, 4.403429997944583008, 11.63237410716304332 ) ) ;
#5324=CARTESIAN_POINT ( 'NONE',  ( -3.011139120916648260, 5.190534000030265105, 18.79931806258173665 ) ) ;
#5326=ORIENTED_EDGE ( 'NONE', *, *, #5914, .T. ) ;
#5327=CARTESIAN_POINT ( 'NONE',  ( -4.070051655338138730, -4.744673454622449604, 17.12632671364005787 ) ) ;
#5329=EDGE_CURVE ( 'NONE', #1423, #6465, #10934, .T. ) ;
#5331=EDGE_CURVE ( 'NONE', #7351, #2035, #5164, .T. ) ;
#5332=CARTESIAN_POINT ( 'NONE',  ( -5.746837578676025515, 1.729433780394186382, 4.000049463537776795 ) ) ;
#5335=FACE_OUTER_BOUND ( 'NONE', #6714, .T. ) ;
#5337=CARTESIAN_POINT ( 'NONE',  ( 5.616089948629725548, -2.743103014345551482, 5.504369696801525436 ) ) ;
#5344=VERTEX_POINT ( 'NONE', #12470 ) ;
#5347=VECTOR ( 'NONE', #13873, 1000.000000000000114 ) ;
#5349=CARTESIAN_POINT ( 'NONE',  ( -3.736532060717933756, -4.696070028786013317, 5.973778239432933290 ) ) ;
#5353=CARTESIAN_POINT ( 'NONE',  ( -5.726307184802639227, -2.506131700382496330, 5.800265150176761253 ) ) ;
#5354=CARTESIAN_POINT ( 'NONE',  ( -2.849573632035372839, 5.280958870664546723, 17.38438267301393481 ) ) ;
#5359=CARTESIAN_POINT ( 'NONE',  ( 4.195842658231422995, 4.289229542213213620, 12.00439760644213294 ) ) ;
#5363=EDGE_CURVE ( 'NONE', #12662, #8844, #3007, .T. ) ;
#5364=CARTESIAN_POINT ( 'NONE',  ( 3.566234721238094707, -5.134387337253790484, 12.49991741810287138 ) ) ;
#5365=CARTESIAN_POINT ( 'NONE',  ( 5.984377695197210301, 1.807429553002331879, 3.999950931234676599 ) ) ;
#5369=CARTESIAN_POINT ( 'NONE',  ( -5.531209434046362894, 2.328189801702562178, 5.873037790270514868 ) ) ;
#5374=CARTESIAN_POINT ( 'NONE',  ( 4.286401442266485340, 4.198423832313245008, 11.36763921416086554 ) ) ;
#5382=CARTESIAN_POINT ( 'NONE',  ( -3.255013540813745720, 5.336859797930771698, 17.12618035954928075 ) ) ;
#5383=B_SPLINE_CURVE_WITH_KNOTS ( 'NONE', 3,
 ( #11958, #10932, #8314, #9505, #14340, #1064, #7202, #15714, #13070, #5847, #1141, #9584, #14427, #6171, #3445, #12043, #3531, #1220 ),
 .UNSPECIFIED., .F., .F.,
 ( 4, 2, 2, 2, 2, 2, 2, 2, 4 ),
 ( 0.003131918686235977359, 0.003523310662250266762, 0.003914702638264556597, 0.004306094614278846433, 0.004697486590293137136, 0.005088878566307427839, 0.005480270542321717675, 0.005871662518336009245, 0.006263054494350299081 ),
 .UNSPECIFIED. ) ;
#5384=CARTESIAN_POINT ( 'NONE',  ( 3.459597053047867465, -5.206576120509730288, 10.52591457665827157 ) ) ;
#5385=CARTESIAN_POINT ( 'NONE',  ( 7.347881158177969135E-16, 6.250000000000000888, 4.000000000000004441 ) ) ;
#5386=CARTESIAN_POINT ( 'NONE',  ( 5.558508435838221295, 2.857531096718872288, 11.63234125634166105 ) ) ;
#5388=CARTESIAN_POINT ( 'NONE',  ( 3.779681992289804615, 4.979315417303895153, 5.999950789842940502 ) ) ;
#5389=CARTESIAN_POINT ( 'NONE',  ( -4.416678568553731310, -4.422441866694230228, 18.26236973443872813 ) ) ;
#5391=CARTESIAN_POINT ( 'NONE',  ( -4.006441409774673446, -4.467329318258270732, 31.79888242247941221 ) ) ;
#5392=FACE_OUTER_BOUND ( 'NONE', #7719, .T. ) ;
#5395=FACE_BOUND ( 'NONE', #27, .T. ) ;
#5396=CARTESIAN_POINT ( 'NONE',  ( -3.158825713737495544, -5.393784879207164096, 10.70066851092422411 ) ) ;
#5400=CARTESIAN_POINT ( 'NONE',  ( -2.668367453516831134, 5.373994336898032742, 17.99999999999998934 ) ) ;
#5402=ORIENTED_EDGE ( 'NONE', *, *, #2616, .F. ) ;
#5403=CARTESIAN_POINT ( 'NONE',  ( -3.255128505894326008, -5.336774832660711176, 17.12619944752603729 ) ) ;
#5404=CARTESIAN_POINT ( 'NONE',  ( 5.931793676715114927, -0.9035324301687286397, 17.73760108194402108 ) ) ;
#5409=DIRECTION ( 'NONE',  ( 0.5877852522924802425, -0.8090169943749422332, 0.000000000000000000 ) ) ;
#5410=CARTESIAN_POINT ( 'NONE',  ( 2.094888807778566729E-14, 6.000000000000000888, 30.00000000000000000 ) ) ;
#5411=CARTESIAN_POINT ( 'NONE',  ( 4.195795028115118619, -4.289273350251234795, 5.504289203620184701 ) ) ;
#5412=CARTESIAN_POINT ( 'NONE',  ( -4.196288036172437508, 4.288789315524846657, 30.49687951097621763 ) ) ;
#5413=DIRECTION ( 'NONE',  ( 0.8090169943749506709, -0.5877852522924689183, 0.000000000000000000 ) ) ;
#5419=CARTESIAN_POINT ( 'NONE',  ( -5.375605342016400279, -2.665598297262502303, 23.99687951097623184 ) ) ;
#5422=FACE_OUTER_BOUND ( 'NONE', #8693, .T. ) ;
#5423=DIRECTION ( 'NONE',  ( 0.000000000000000000, 1.000000000000000000, 0.000000000000000000 ) ) ;
#5426=CARTESIAN_POINT ( 'NONE',  ( -0.9735856429311440241, 5.920699391845048787, 18.26285283906727486 ) ) ;
#5427=CARTESIAN_POINT ( 'NONE',  ( -0.9999505860951506397, 6.169489349035837122, 24.63105903165801180 ) ) ;
#5434=ADVANCED_FACE ( 'NONE', ( #3316 ), #13094, .F. ) ;
#5435=ORIENTED_EDGE ( 'NONE', *, *, #11555, .F. ) ;
#5437=ORIENTED_EDGE ( 'NONE', *, *, #2729, .F. ) ;
#5438=CARTESIAN_POINT ( 'NONE',  ( 2.841163418881348601, -5.567120626447951359, 18.26236973443873524 ) ) ;
#5440=EDGE_CURVE ( 'NONE', #14829, #8273, #1958, .T. ) ;
#5445=CARTESIAN_POINT ( 'NONE',  ( -5.782947755040686033, 1.603807858343911930, 5.973980201222398811 ) ) ;
#5448=CARTESIAN_POINT ( 'NONE',  ( 5.915699123067175158, -1.003533581835451383, 12.00389795015984973 ) ) ;
#5449=ADVANCED_FACE ( 'NONE', ( #7062 ), #5790, .F. ) ;
#5450=CARTESIAN_POINT ( 'NONE',  ( 4.195795028115012926, 4.289273350251342265, 10.99571079637980908 ) ) ;
#5455=EDGE_LOOP ( 'NONE', ( #1211, #4792 ) ) ;
#5457=ADVANCED_FACE ( 'NONE', ( #13978 ), #10405, .F. ) ;
#5459=CARTESIAN_POINT ( 'NONE',  ( -0.9735954530124610873, 6.173909381474003588, 11.76281793585240898 ) ) ;
#5461=CARTESIAN_POINT ( 'NONE',  ( 4.195842658231450528, -4.289229542213186086, 17.49560239355786706 ) ) ;
#5464=CARTESIAN_POINT ( 'NONE',  ( 2.841163418881336167, 5.567120626447958465, 11.23763026556121680 ) ) ;
#5466=CARTESIAN_POINT ( 'NONE',  ( -4.290821322214338096, -4.545321419741590319, 31.61441947245485196 ) ) ;
#5468=B_SPLINE_CURVE_WITH_KNOTS ( 'NONE', 3,
 ( #7492, #14739, #7722, #4140, #8775, #13606, #8121, #14227, #5427, #5735, #1984, #10579, #12877, #7802, #6857, #793, #13998, #11693 ),
 .UNSPECIFIED., .F., .F.,
 ( 4, 2, 2, 2, 2, 2, 2, 2, 4 ),
 ( 0.000000000000000000, 0.0003914362731607349145, 0.0007828725463214698289, 0.001174308819482204743, 0.001565745092642939658, 0.001957181365803674356, 0.002348617638964409487, 0.002740053912125144618, 0.003131490185285879316 ),
 .UNSPECIFIED. ) ;
#5470=CARTESIAN_POINT ( 'NONE',  ( -4.142620314836317874, -4.341347824677564304, 31.61442521571936837 ) ) ;
#5475=CYLINDRICAL_SURFACE ( 'NONE', #3217, 1.000000000000000888 ) ;
#5476=CARTESIAN_POINT ( 'NONE',  ( -5.375605342016473998, 2.665598297262353533, 18.50312048902377526 ) ) ;
#5483=CARTESIAN_POINT ( 'NONE',  ( -3.011139120916564327, -5.190534000030312178, 17.20068193741824558 ) ) ;
#5486=CARTESIAN_POINT ( 'NONE',  ( -7.799024015210657801, -1.482594289697236389, 31.00000000000000000 ) ) ;
#5488=CARTESIAN_POINT ( 'NONE',  ( 2.030576276931546336E-13, -6.250000000000000888, 25.49999999999999645 ) ) ;
#5489=CARTESIAN_POINT ( 'NONE',  ( -0.1306497350717108763, 6.000000000000002665, 30.00000000000000711 ) ) ;
#5491=CARTESIAN_POINT ( 'NONE',  ( 6.106056299406789734, -1.336851112280482035, 23.70112161576661336 ) ) ;
#5492=CARTESIAN_POINT ( 'NONE',  ( -5.317509234263969375, 2.779225709350973350, 5.000000000000004441 ) ) ;
#5494=ORIENTED_EDGE ( 'NONE', *, *, #9992, .T. ) ;
#5496=CARTESIAN_POINT ( 'NONE',  ( -0.9999502950801375523, 5.916088184763895086, 11.63108149190012064 ) ) ;
#5499=CYLINDRICAL_SURFACE ( 'NONE', #5066, 1.000000000000000888 ) ;
#5501=CARTESIAN_POINT ( 'NONE',  ( -5.866923913994636308, -1.260079467906572770, 30.20047945897284336 ) ) ;
#5502=CARTESIAN_POINT ( 'NONE',  ( -0.5044069930201934282, 5.979990686695005664, 18.87335743227902896 ) ) ;
#5503=( NAMED_UNIT ( * ) PLANE_ANGLE_UNIT ( ) SI_UNIT ( $, .RADIAN. ) );
#5504=CARTESIAN_POINT ( 'NONE',  ( -3.781065399485917133, -4.978303713186513768, 5.999917418102895361 ) ) ;
#5508=DIRECTION ( 'NONE',  ( -0.9510565162951545304, 0.3090169943749447867, 0.000000000000000000 ) ) ;
#5509=CARTESIAN_POINT ( 'NONE',  ( -5.665308849928776702, -1.980336949702643512, 17.00007997643737312 ) ) ;
#5512=ORIENTED_EDGE ( 'NONE', *, *, #5166, .T. ) ;
#5514=CARTESIAN_POINT ( 'NONE',  ( 3.106366801611900819, -5.134708448381346102, 25.37303779027051576 ) ) ;
#5515=DIRECTION ( 'NONE',  ( -0.9510565162951544194, 0.3090169943749447312, 0.000000000000000000 ) ) ;
#5516=VERTEX_POINT ( 'NONE', #15414 ) ;
#5520=CARTESIAN_POINT ( 'NONE',  ( -2.931156713028478134, 5.520271803279214851, 31.50436969680152899 ) ) ;
#5524=EDGE_CURVE ( 'NONE', #8289, #6892, #9619, .T. ) ;
#5525=CARTESIAN_POINT ( 'NONE',  ( -5.131373506000731055, 7.062729720844018289, 31.00000000000000000 ) ) ;
#5533=B_SPLINE_CURVE_WITH_KNOTS ( 'NONE', 3,
 ( #14440, #13009, #10631, #8250, #8414, #3621, #9766, #8328, #14522, #7055, #12055, #3543, #9683, #6104, #15567, #4747, #5785, #2347 ),
 .UNSPECIFIED., .F., .F.,
 ( 4, 2, 2, 2, 2, 2, 2, 2, 4 ),
 ( 0.003131918686235970421, 0.003523310662250261124, 0.003914702638264551393, 0.004306094614278842096, 0.004697486590293132799, 0.005088878566307422635, 0.005480270542321714206, 0.005871662518336004041, 0.006263054494350294744 ),
 .UNSPECIFIED. ) ;
#5534=VERTEX_POINT ( 'NONE', #3469 ) ;
#5535=LINE ( 'NONE', #14337, #8364 ) ;
#5537=CARTESIAN_POINT ( 'NONE',  ( 2.094888806938587637E-14, 6.250000000000000888, 30.00000000000000000 ) ) ;
#5538=CARTESIAN_POINT ( 'NONE',  ( -0.2622916576876674899, 5.995491482261829042, 5.973849426468138546 ) ) ;
#5540=DIRECTION ( 'NONE',  ( 0.9510565162951499785, 0.3090169943749582204, 0.000000000000000000 ) ) ;
#5544=CARTESIAN_POINT ( 'NONE',  ( -4.322356511625788045, 7.650514973136498753, 31.00000000000000000 ) ) ;
#5551=DIRECTION ( 'NONE',  ( 0.000000000000000000, 0.000000000000000000, -1.000000000000000000 ) ) ;
#5552=CARTESIAN_POINT ( 'NONE',  ( 0.8730628416139659675, 6.188929913094928459, 23.99504929893123517 ) ) ;
#5555=CARTESIAN_POINT ( 'NONE',  ( -4.416837305303647376, 4.422286678978860408, 24.76190213084012726 ) ) ;
#5557=FACE_OUTER_BOUND ( 'NONE', #13867, .T. ) ;
#5559=ADVANCED_FACE ( 'NONE', ( #1241 ), #14449, .F. ) ;
#5561=CARTESIAN_POINT ( 'NONE',  ( -5.866984344570817633, 1.259800266528702917, 23.70068193741825269 ) ) ;
#5563=CARTESIAN_POINT ( 'NONE',  ( 5.317509234263979145, -2.779225709350955142, 31.00000000000000000 ) ) ;
#5567=CARTESIAN_POINT ( 'NONE',  ( -5.903119516422476565, -1.077859910107483943, 5.615193824488508234 ) ) ;
#5569=DIRECTION ( 'NONE',  ( -0.3090169943749447867, -0.9510565162951544194, 0.000000000000000000 ) ) ;
#5572=ORIENTED_EDGE ( 'NONE', *, *, #6976, .T. ) ;
#5574=CARTESIAN_POINT ( 'NONE',  ( -0.6152055445545627776, 5.969096820685162896, 12.29904968670266108 ) ) ;
#5575=VERTEX_POINT ( 'NONE', #7376 ) ;
#5576=DIRECTION ( 'NONE',  ( -0.3090169943749579429, 0.9510565162951502005, 0.000000000000000000 ) ) ;
#5577=CARTESIAN_POINT ( 'NONE',  ( 5.131373506000584506, 7.062729720844102665, 31.00000000000000000 ) ) ;
#5578=B_SPLINE_CURVE_WITH_KNOTS ( 'NONE', 3,
 ( #12987, #2985, #12914, #1936, #2015, #6810, #513, #7836, #6656, #11645, #6888, #5382, #6733, #825, #7911, #15080, #1781, #11487 ),
 .UNSPECIFIED., .F., .F.,
 ( 4, 2, 2, 2, 2, 2, 2, 2, 4 ),
 ( 0.003131486019301991160, 0.003522824630466697866, 0.003914163241631405006, 0.004305501852796111278, 0.004696840463960818418, 0.005088179075125525558, 0.005479517686290231830, 0.005870856297454938102, 0.006262194908619645242 ),
 .UNSPECIFIED. ) ;
#5579=CARTESIAN_POINT ( 'NONE',  ( -5.375605342016489097, -2.665598297262326444, 30.49687951097621053 ) ) ;
#5580=FACE_OUTER_BOUND ( 'NONE', #11484, .T. ) ;
#5581=CARTESIAN_POINT ( 'NONE',  ( 5.935543223013866942, 0.8771126767606117758, 17.99999999999998934 ) ) ;
#5583=CARTESIAN_POINT ( 'NONE',  ( -3.159082487394711869, -5.393634094348371377, 5.799544624688432570 ) ) ;
#5585=CARTESIAN_POINT ( 'NONE',  ( 4.005998022989988527, -4.467726698309236077, 10.70068193741824913 ) ) ;
#5587=CYLINDRICAL_SURFACE ( 'NONE', #6745, 1.000000000000000888 ) ;
#5589=CARTESIAN_POINT ( 'NONE',  ( -4.286401442266546624, -4.198423832313178394, 31.00000000000000000 ) ) ;
#5593=ORIENTED_EDGE ( 'NONE', *, *, #677, .F. ) ;
#5594=CARTESIAN_POINT ( 'NONE',  ( -6.081509788407728045, -1.446521464462759976, 10.62618035954927898 ) ) ;
#5597=CARTESIAN_POINT ( 'NONE',  ( 5.317509234264033324, -2.779225709350851670, 18.13239388001634467 ) ) ;
#5599=CARTESIAN_POINT ( 'NONE',  ( -0.6152055445544284407, 5.969096820685177995, 25.29904968670266996 ) ) ;
#5600=CARTESIAN_POINT ( 'NONE',  ( -3.567624405365222628, -5.133384272590791220, 4.000049210157070156 ) ) ;
#5603=DIRECTION ( 'NONE',  ( 0.8090169943749506709, -0.5877852522924686962, 0.000000000000000000 ) ) ;
#5606=CARTESIAN_POINT ( 'NONE',  ( -5.903057025253906964, -1.078199533779497177, 4.384382673013948128 ) ) ;
#5609=VERTEX_POINT ( 'NONE', #7225 ) ;
#5613=CARTESIAN_POINT ( 'NONE',  ( -0.2619041840694215084, 6.245686665308503471, 10.52605849433793672 ) ) ;
#5617=CARTESIAN_POINT ( 'NONE',  ( 3.458623254138665448, 5.207221900902852418, 10.52622717124729945 ) ) ;
#5619=FACE_BOUND ( 'NONE', #10787, .T. ) ;
#5620=CARTESIAN_POINT ( 'NONE',  ( 4.069684453406282820, -4.744965295353568813, 17.12619944752603729 ) ) ;
#5625=ADVANCED_FACE ( 'NONE', ( #4834 ), #14614, .F. ) ;
#5627=FACE_BOUND ( 'NONE', #10514, .T. ) ;
#5628=CARTESIAN_POINT ( 'NONE',  ( -5.915641100987815371, 1.003868594704848238, 18.50428920362019269 ) ) ;
#5631=B_SPLINE_CURVE_WITH_KNOTS ( 'NONE', 3,
 ( #2620, #7476, #12320, #1415, #7549, #3729, #1342, #9869, #6452, #2698, #151, #8607, #12474, #11131, #14870, #6373, #4043, #2545 ),
 .UNSPECIFIED., .F., .F.,
 ( 4, 2, 2, 2, 2, 2, 2, 2, 4 ),
 ( 0.000000000000000000, 0.0003914898357794973868, 0.0007829796715589947735, 0.001174469507338492215, 0.001565959343117989547, 0.001957449178897487096, 0.002348939014676984429, 0.002740428850456481762, 0.003131918686235979094 ),
 .UNSPECIFIED. ) ;
#5633=CARTESIAN_POINT ( 'NONE',  ( -4.152999119458150368, 4.671604476854199106, 25.30026515017674171 ) ) ;
#5634=CARTESIAN_POINT ( 'NONE',  ( -0.9739805876845880617, -5.920636045238200751, 24.76171386814422704 ) ) ;
#5636=CARTESIAN_POINT ( 'NONE',  ( -5.558508435838166228, 2.857531096718976649, 17.99999999999998934 ) ) ;
#5638=DIRECTION ( 'NONE',  ( 0.5877852522924802425, -0.8090169943749422332, 0.000000000000000000 ) ) ;
#5640=CARTESIAN_POINT ( 'NONE',  ( 2.082642335314403343E-14, 6.000000000000000888, 32.00000000000000000 ) ) ;
#5644=VECTOR ( 'NONE', #4379, 1000.000000000000114 ) ;
#5646=ORIENTED_EDGE ( 'NONE', *, *, #9307, .F. ) ;
#5648=CARTESIAN_POINT ( 'NONE',  ( 7.180990026460803755, -3.384707322287205944, 24.49999999999999289 ) ) ;
#5649=ORIENTED_EDGE ( 'NONE', *, *, #11273, .F. ) ;
#5651=DIRECTION ( 'NONE',  ( -0.5877852522924685852, -0.8090169943749508930, 0.000000000000000000 ) ) ;
#5655=B_SPLINE_CURVE_WITH_KNOTS ( 'NONE', 3,
 ( #1266, #1345, #14558, #13445, #8686, #3654, #10979, #7402, #12245, #11055, #154, #14873, #15032, #12477, #12399, #6293, #7707, #4126 ),
 .UNSPECIFIED., .F., .F.,
 ( 4, 2, 2, 2, 2, 2, 2, 2, 4 ),
 ( 0.003131918686235975625, 0.003523310662250265894, 0.003914702638264555730, 0.004306094614278846433, 0.004697486590293136269, 0.005088878566307426105, 0.005480270542321715940, 0.005871662518336005776, 0.006263054494350296479 ),
 .UNSPECIFIED. ) ;
#5656=ADVANCED_FACE ( 'NONE', ( #13801 ), #2754, .F. ) ;
#5657=CARTESIAN_POINT ( 'NONE',  ( 5.903347812666365435, 1.076697810262510213, 17.38602261056917087 ) ) ;
#5659=DIRECTION ( 'NONE',  ( 0.000000000000000000, 1.000000000000000000, 0.000000000000000000 ) ) ;
#5661=DIRECTION ( 'NONE',  ( 0.000000000000000000, 0.000000000000000000, 1.000000000000000000 ) ) ;
#5664=CARTESIAN_POINT ( 'NONE',  ( 4.435347140100995844, 4.403429997944549257, 31.00000000000000000 ) ) ;
#5665=CARTESIAN_POINT ( 'NONE',  ( 5.935543223013857173, 0.8771126767606810537, 11.63061695532135609 ) ) ;
#5667=AXIS2_PLACEMENT_3D ( 'NONE', #5856, #4423, #9590 ) ;
#5668=ORIENTED_EDGE ( 'NONE', *, *, #9950, .F. ) ;
#5670=CARTESIAN_POINT ( 'NONE',  ( 4.005785023174367687, -4.467917056767481299, 25.29952054102715309 ) ) ;
#5671=FACE_OUTER_BOUND ( 'NONE', #10985, .T. ) ;
#5673=CARTESIAN_POINT ( 'NONE',  ( 5.866817325727538446, -1.260653813891827291, 18.80022217383877958 ) ) ;
#5675=CARTESIAN_POINT ( 'NONE',  ( 7.347880794884119736E-16, -6.250000000000000888, 4.000000000000004441 ) ) ;
#5680=CYLINDRICAL_SURFACE ( 'NONE', #7694, 0.9999999999999998890 ) ;
#5683=CARTESIAN_POINT ( 'NONE',  ( -7.180990026460705167, -3.384707322287646480, 17.99999999999998934 ) ) ;
#5690=CARTESIAN_POINT ( 'NONE',  ( 2.841163418881473834, -5.567120626447887410, 5.262369734438755664 ) ) ;
#5691=ADVANCED_FACE ( 'NONE', ( #1705 ), #6581, .F. ) ;
#5692=CARTESIAN_POINT ( 'NONE',  ( 7.490007020835706797, -2.433650805992179755, 11.49999999999998224 ) ) ;
#5694=CARTESIAN_POINT ( 'NONE',  ( -0.6139908388541001072, 5.969238533166612015, 4.199776279120134070 ) ) ;
#5696=CARTESIAN_POINT ( 'NONE',  ( 3.566234721238037864, 5.134387337253831340, 10.50008258189709132 ) ) ;
#5697=FACE_BOUND ( 'NONE', #498, .T. ) ;
#5705=FACE_BOUND ( 'NONE', #7483, .T. ) ;
#5706=LINE ( 'NONE', #10550, #6209 ) ;
#5710=CYLINDRICAL_SURFACE ( 'NONE', #7077, 1.000000000000000888 ) ;
#5711=DIRECTION ( 'NONE',  ( 0.8090169943749506709, -0.5877852522924689183, 0.000000000000000000 ) ) ;
#5713=CARTESIAN_POINT ( 'NONE',  ( -5.858813228503629844, 2.179803269293333123, 18.97377282875267213 ) ) ;
#5714=ORIENTED_EDGE ( 'NONE', *, *, #3943, .T. ) ;
#5715=VECTOR ( 'NONE', #7872, 1000.000000000000114 ) ;
#5718=ADVANCED_FACE ( 'NONE', ( #9127 ), #15238, .F. ) ;
#5721=CARTESIAN_POINT ( 'NONE',  ( -0.6152055445546077417, 5.969096820685158455, 31.79904968670268417 ) ) ;
#5722=EDGE_CURVE ( 'NONE', #6460, #5344, #6815, .T. ) ;
#5724=FACE_BOUND ( 'NONE', #2244, .T. ) ;
#5725=CARTESIAN_POINT ( 'NONE',  ( -5.615973259022345232, 2.743340227996120539, 4.496107868750329750 ) ) ;
#5726=DIRECTION ( 'NONE',  ( -1.000000000000000000, 0.000000000000000000, 0.000000000000000000 ) ) ;
#5729=CARTESIAN_POINT ( 'NONE',  ( 4.195795028115036018, 4.289273350251318284, 30.49571079637980020 ) ) ;
#5732=CARTESIAN_POINT ( 'NONE',  ( -2.668367453516726773, 5.373994336898084256, 31.13239388001635177 ) ) ;
#5733=CARTESIAN_POINT ( 'NONE',  ( 2.996920846510391812, 5.485395142346844111, 17.38558052754515160 ) ) ;
#5735=CARTESIAN_POINT ( 'NONE',  ( -1.000049271338272705, 6.169473353325585663, 24.36969612704542243 ) ) ;
#5737=CARTESIAN_POINT ( 'NONE',  ( 3.312524433819828307, -5.004191858253970615, 10.52591947216897772 ) ) ;
#5740=CIRCLE ( 'NONE', #131, 6.250000000000000888 ) ;
#5742=CARTESIAN_POINT ( 'NONE',  ( -5.486741141153726353, -2.429871531109881300, 17.20111757752057002 ) ) ;
#5743=EDGE_CURVE ( 'NONE', #12482, #12866, #4478, .T. ) ;
#5744=FACE_OUTER_BOUND ( 'NONE', #4074, .T. ) ;
#5746=VERTEX_POINT ( 'NONE', #5772 ) ;
#5748=CARTESIAN_POINT ( 'NONE',  ( 2.817313151351090728, 5.579000502529481764, 30.86939309276503351 ) ) ;
#5749=CARTESIAN_POINT ( 'NONE',  ( -3.632151824461123724, 4.777505256984569293, 12.50004932073310471 ) ) ;
#5750=ORIENTED_EDGE ( 'NONE', *, *, #8030, .F. ) ;
#5752=CARTESIAN_POINT ( 'NONE',  ( 0.5039079366032432894, -5.980031194523151683, 4.126370681098135762 ) ) ;
#5753=CARTESIAN_POINT ( 'NONE',  ( -2.841041022017302797, -5.567186575787308023, 4.737747182782873878 ) ) ;
#5760=B_SPLINE_CURVE_WITH_KNOTS ( 'NONE', 3,
 ( #8759, #14874, #2549, #3886, #12171, #6294, #3813, #312, #2384, #5098, #79, #10905, #12324, #9949, #14801, #14646, #9723, #4865 ),
 .UNSPECIFIED., .F., .F.,
 ( 4, 2, 2, 2, 2, 2, 2, 2, 4 ),
 ( 0.003131490185286092253, 0.003522829482338693183, 0.003914168779391293679, 0.004305508076443895042, 0.004696847373496496406, 0.005088186670549096902, 0.005479525967601697398, 0.005870865264654297894, 0.006262204561706899257 ),
 .UNSPECIFIED. ) ;
#5766=CARTESIAN_POINT ( 'NONE',  ( 2.848235266351075268, -5.281699484015620172, 4.386022610569179747 ) ) ;
#5767=EDGE_LOOP ( 'NONE', ( #1742, #11702 ) ) ;
#5769=DIRECTION ( 'NONE',  ( -0.3090169943749446202, -0.9510565162951544194, 0.000000000000000000 ) ) ;
#5772=CARTESIAN_POINT ( 'NONE',  ( -5.935543223013841185, 0.8771126767608004027, 17.99999999999998934 ) ) ;
#5773=CARTESIAN_POINT ( 'NONE',  ( 3.312524433819643122, 5.004191858254092296, 25.47408052783099919 ) ) ;
#5774=FACE_BOUND ( 'NONE', #14628, .T. ) ;
#5775=CARTESIAN_POINT ( 'NONE',  ( -2.997753866155852265, -5.484939622623827837, 18.61560192892920895 ) ) ;
#5778=CYLINDRICAL_SURFACE ( 'NONE', #11786, 0.9999999999999998890 ) ;
#5782=B_SPLINE_CURVE_WITH_KNOTS ( 'NONE', 3,
 ( #5664, #7966, #14004, #637, #10511, #15366, #14157, #3260, #2066, #3036, #10354, #3112, #7014, #6939, #4307, #7889, #874, #954 ),
 .UNSPECIFIED., .F., .F.,
 ( 4, 2, 2, 2, 2, 2, 2, 2, 4 ),
 ( 0.000000000000000000, 0.0003914357524127466182, 0.0007828715048254932364, 0.001174307257238239909, 0.001565743009650987557, 0.001957178762063734988, 0.002348614514476482420, 0.002740050266889230285, 0.003131486019301977716 ),
 .UNSPECIFIED. ) ;
#5783=CARTESIAN_POINT ( 'NONE',  ( 3.922288969639774248, 4.542045818322530515, 31.87378430870261425 ) ) ;
#5785=CARTESIAN_POINT ( 'NONE',  ( 5.317509234263941842, 2.779225709351030638, 31.13236078583911493 ) ) ;
#5787=CARTESIAN_POINT ( 'NONE',  ( 5.935543223013856284, 0.8771126767606806096, 11.49999999999998224 ) ) ;
#5789=ORIENTED_EDGE ( 'NONE', *, *, #3262, .F. ) ;
#5790=CYLINDRICAL_SURFACE ( 'NONE', #7406, 1.000000000000000666 ) ;
#5794=CARTESIAN_POINT ( 'NONE',  ( 5.770288754215171956, 2.404361317819856403, 25.37381964045071214 ) ) ;
#5798=FACE_BOUND ( 'NONE', #7414, .T. ) ;
#5800=CARTESIAN_POINT ( 'NONE',  ( 0.000000000000000000, 0.000000000000000000, 36.00000000000000711 ) ) ;
#5801=VERTEX_POINT ( 'NONE', #10464 ) ;
#5810=CARTESIAN_POINT ( 'NONE',  ( -2.668367453516725885, 5.373994336898083368, 31.00000000000000000 ) ) ;
#5811=EDGE_CURVE ( 'NONE', #5746, #3666, #9981, .T. ) ;
#5815=CARTESIAN_POINT ( 'NONE',  ( 2.668367453516584664, -5.373994336898154422, 18.13061695532137918 ) ) ;
#5817=AXIS2_PLACEMENT_3D ( 'NONE', #15552, #30, #6386 ) ;
#5818=CARTESIAN_POINT ( 'NONE',  ( -6.081509788407743144, -1.446521464462711570, 4.126180359549291410 ) ) ;
#5822=CARTESIAN_POINT ( 'NONE',  ( 5.747343991580187605, 1.727858744772266419, 12.49992002356259668 ) ) ;
#5824=EDGE_LOOP ( 'NONE', ( #6885, #5141, #9172, #6692 ) ) ;
#5826=VERTEX_POINT ( 'NONE', #9585 ) ;
#5829=ORIENTED_EDGE ( 'NONE', *, *, #494, .F. ) ;
#5831=CARTESIAN_POINT ( 'NONE',  ( -0.2619456584319997949, 5.995505046955622142, 23.52607193928647433 ) ) ;
#5832=CARTESIAN_POINT ( 'NONE',  ( 4.435347140100866170, 4.403429997944680707, 24.63237410716306286 ) ) ;
#5835=CARTESIAN_POINT ( 'NONE',  ( 5.317509234263995133, 2.779225709350928053, 17.99999999999998934 ) ) ;
#5841=ORIENTED_EDGE ( 'NONE', *, *, #6538, .T. ) ;
#5843=ORIENTED_EDGE ( 'NONE', *, *, #8342, .F. ) ;
#5844=EDGE_LOOP ( 'NONE', ( #11525, #10112 ) ) ;
#5845=CARTESIAN_POINT ( 'NONE',  ( -5.858813228503639614, -2.179803269293304258, 30.02622717124732077 ) ) ;
#5846=CARTESIAN_POINT ( 'NONE',  ( -4.344502777243634206, -4.493369211529165241, 23.99610786875030755 ) ) ;
#5847=CARTESIAN_POINT ( 'NONE',  ( -3.420311045507915981, -4.931422832349241503, 25.50007961174475923 ) ) ;
#5850=CARTESIAN_POINT ( 'NONE',  ( -6.172639027853117355, -0.9816353142771756524, 31.26225281721713145 ) ) ;
#5852=CARTESIAN_POINT ( 'NONE',  ( -0.7995524673975737961, -6.199337389817267230, 5.614536794524584984 ) ) ;
#5853=CARTESIAN_POINT ( 'NONE',  ( -0.8730628416135229886, -6.188929913094992408, 23.99504929893116056 ) ) ;
#5854=CARTESIAN_POINT ( 'NONE',  ( -2.817313151351230172, -5.579000502529412486, 17.99999999999998934 ) ) ;
#5855=CARTESIAN_POINT ( 'NONE',  ( 0.6139908388542412165, -5.969238533166598693, 17.19977627912011542 ) ) ;
#5856=CARTESIAN_POINT ( 'NONE',  ( 5.131373506000599605, 7.062729720844090231, 5.000000000000004441 ) ) ;
#5860=CARTESIAN_POINT ( 'NONE',  ( -5.984595133899131447, -1.806709459528820227, 18.99995078984292007 ) ) ;
#5862=EDGE_LOOP ( 'NONE', ( #3795, #9580 ) ) ;
#5863=CARTESIAN_POINT ( 'NONE',  ( -5.375605342016499755, 2.665598297262299354, 12.00312048902375217 ) ) ;
#5864=CARTESIAN_POINT ( 'NONE',  ( 6.780834053290958173E-14, -6.000000000000000888, 10.49999999999998224 ) ) ;
#5865=CARTESIAN_POINT ( 'NONE',  ( -0.2624013748571158433, -5.995472630654528956, 23.52628559691083154 ) ) ;
#5871=B_SPLINE_CURVE_WITH_KNOTS ( 'NONE', 3,
 ( #11435, #536, #5404, #10252, #15104, #6010, #7205, #9069, #11962, #6756, #4578, #1880, #13979, #10619, #8405, #7044, #15180, #2256 ),
 .UNSPECIFIED., .F., .F.,
 ( 4, 2, 2, 2, 2, 2, 2, 2, 4 ),
 ( 0.003131918686235972589, 0.003523310662250263292, 0.003914702638264553995, 0.004306094614278844698, 0.004697486590293136269, 0.005088878566307426105, 0.005480270542321717675, 0.005871662518336008378, 0.006263054494350299081 ),
 .UNSPECIFIED. ) ;
#5876=FACE_OUTER_BOUND ( 'NONE', #8990, .T. ) ;
#5879=FACE_OUTER_BOUND ( 'NONE', #7219, .T. ) ;
#5885=CARTESIAN_POINT ( 'NONE',  ( 5.329945432499665792, 2.755769831645062506, 24.23770962164067200 ) ) ;
#5888=CARTESIAN_POINT ( 'NONE',  ( 0.2622538972266198476, -6.245673238944467798, 25.47385994369200191 ) ) ;
#5892=CARTESIAN_POINT ( 'NONE',  ( 4.141923667210617666, -4.342011609040492104, 18.61561732698604743 ) ) ;
#5896=CARTESIAN_POINT ( 'NONE',  ( -5.935543223013851843, 0.8771126767607326791, 11.36760611998364823 ) ) ;
#5898=CARTESIAN_POINT ( 'NONE',  ( -0.2638277032947476952, -5.995407492418047823, 18.97332055281517427 ) ) ;
#5899=EDGE_CURVE ( 'NONE', #7142, #7332, #9410, .T. ) ;
#5901=ORIENTED_EDGE ( 'NONE', *, *, #9837, .T. ) ;
#5906=ORIENTED_EDGE ( 'NONE', *, *, #2821, .T. ) ;
#5909=CARTESIAN_POINT ( 'NONE',  ( 6.155973317223301322, 1.081218830693648103, 18.50308643866044633 ) ) ;
#5910=CARTESIAN_POINT ( 'NONE',  ( -4.322356511625880415, 7.650514973136431252, 17.99999999999998934 ) ) ;
#5913=CARTESIAN_POINT ( 'NONE',  ( 5.726049995854467944, -2.506679546901878552, 4.200455375311575423 ) ) ;
#5914=EDGE_CURVE ( 'NONE', #3929, #11668, #7124, .T. ) ;
#5917=CARTESIAN_POINT ( 'NONE',  ( 3.779681992289859682, -4.979315417303849856, 30.00004921015706216 ) ) ;
#5921=ORIENTED_EDGE ( 'NONE', *, *, #5922, .T. ) ;
#5922=EDGE_CURVE ( 'NONE', #15454, #12751, #7136, .T. ) ;
#5924=ORIENTED_EDGE ( 'NONE', *, *, #7856, .F. ) ;
#5925=VERTEX_POINT ( 'NONE', #6008 ) ;
#5926=CARTESIAN_POINT ( 'NONE',  ( -5.615811513734994875, -2.743665920700480765, 30.49691356133953590 ) ) ;
#5927=CARTESIAN_POINT ( 'NONE',  ( 2.848235266350942929, -5.281699484015692114, 17.38602261056917797 ) ) ;
#5928=CARTESIAN_POINT ( 'NONE',  ( 0.9999505860953422642, -6.169489349035806924, 5.131059031658107727 ) ) ;
#5929=CARTESIAN_POINT ( 'NONE',  ( 3.311576095066596892, -5.004818610361295939, 12.47377823943291730 ) ) ;
#5930=CARTESIAN_POINT ( 'NONE',  ( -1.000082492230715436, -6.169467968613708386, 5.131525381053921642 ) ) ;
#5931=DIRECTION ( 'NONE',  ( 0.5877852522924802425, -0.8090169943749422332, 0.000000000000000000 ) ) ;
#5932=CARTESIAN_POINT ( 'NONE',  ( -2.931212650151701293, -5.520239928492797432, 18.50425949503010514 ) ) ;
#5933=CARTESIAN_POINT ( 'NONE',  ( -6.105861027178912437, -1.337741388557158073, 23.70045537531158075 ) ) ;
#5938=CARTESIAN_POINT ( 'NONE',  ( 2.848235266350975792, 5.281699484015673463, 31.61397738943082203 ) ) ;
#5939=EDGE_CURVE ( 'NONE', #12984, #15268, #15672, .T. ) ;
#5940=EDGE_CURVE ( 'NONE', #9955, #7970, #11297, .T. ) ;
#5942=VERTEX_POINT ( 'NONE', #7741 ) ;
#5944=CARTESIAN_POINT ( 'NONE',  ( 0.8737888311110715289, -5.936248257219499003, 12.00344185141215192 ) ) ;
#5947=CARTESIAN_POINT ( 'NONE',  ( 2.930600586413029784, -5.520563544161715797, 31.50308643866046054 ) ) ;
#5949=CARTESIAN_POINT ( 'NONE',  ( -4.435347140101025154, -4.403429997944519947, 31.13060690723500201 ) ) ;
#5950=VECTOR ( 'NONE', #621, 1000.000000000000114 ) ;
#5954=CARTESIAN_POINT ( 'NONE',  ( -6.176542424588111757, 0.9554180641286129649, 11.63234125634166105 ) ) ;
#5956=CARTESIAN_POINT ( 'NONE',  ( -3.255128505894301583, 5.336774832660725387, 5.873800552473966263 ) ) ;
#5958=CARTESIAN_POINT ( 'NONE',  ( -2.668367453516726329, 5.373994336898084256, 30.86763921416088863 ) ) ;
#5960=CARTESIAN_POINT ( 'NONE',  ( 6.105747081304190083, 1.338335777572186469, 17.19973484982324763 ) ) ;
#5961=VERTEX_POINT ( 'NONE', #7510 ) ;
#5965=CARTESIAN_POINT ( 'NONE',  ( 5.931828553037990837, 0.9033193133618145909, 24.23805675996852926 ) ) ;
#5966=ORIENTED_EDGE ( 'NONE', *, *, #5329, .F. ) ;
#5969=CARTESIAN_POINT ( 'NONE',  ( 0.8736772044962008987, -6.188841968496030965, 23.99611573292810718 ) ) ;
#5973=CARTESIAN_POINT ( 'NONE',  ( 2.692143549875461783, -5.362363179736447272, 30.73805675996853637 ) ) ;
#5975=CARTESIAN_POINT ( 'NONE',  ( -0.9739805876847694721, -5.920636045238170553, 31.26171386814423414 ) ) ;
#5979=CARTESIAN_POINT ( 'NONE',  ( 2.692335458626711642, 5.362264153667302580, 24.23760108194402108 ) ) ;
#5981=EDGE_CURVE ( 'NONE', #6465, #1423, #4856, .T. ) ;
#5982=VERTEX_POINT ( 'NONE', #11166 ) ;
#5984=VERTEX_POINT ( 'NONE', #11086 ) ;
#5985=FACE_OUTER_BOUND ( 'NONE', #12647, .T. ) ;
#5995=CARTESIAN_POINT ( 'NONE',  ( 4.069684453406374303, -4.744965295353490653, 4.126199447526043507 ) ) ;
#5997=CARTESIAN_POINT ( 'NONE',  ( 6.768587589771821120E-14, -6.250000000000000888, 12.49999999999998401 ) ) ;
#6001=VERTEX_POINT ( 'NONE', #6486 ) ;
#6002=VERTEX_POINT ( 'NONE', #8794 ) ;
#6004=EDGE_CURVE ( 'NONE', #11257, #15393, #1233, .T. ) ;
#6008=CARTESIAN_POINT ( 'NONE',  ( 6.176542424588105540, 0.9554180641286316167, 5.000000000000004441 ) ) ;
#6010=CARTESIAN_POINT ( 'NONE',  ( 5.867109477881265356, -1.259218163100813026, 17.20111757752057713 ) ) ;
#6011=CARTESIAN_POINT ( 'NONE',  ( -4.006441409774713414, -4.467329318258233428, 12.29888242247937669 ) ) ;
#6020=CARTESIAN_POINT ( 'NONE',  ( 5.558508435838291462, -2.857531096718732844, 17.86765874365829276 ) ) ;
#6025=CARTESIAN_POINT ( 'NONE',  ( 0.9740807849836848886, -5.920620690450679291, 11.23850119700669126 ) ) ;
#6028=CARTESIAN_POINT ( 'NONE',  ( 4.290130679986615903, -4.545972905167685596, 31.61560192892919829 ) ) ;
#6030=ORIENTED_EDGE ( 'NONE', *, *, #9396, .F. ) ;
#6031=CARTESIAN_POINT ( 'NONE',  ( 4.435347140100866170, 4.403429997944678931, 24.36765874365828921 ) ) ;
#6035=DIRECTION ( 'NONE',  ( 0.9510565162951499785, 0.3090169943749582204, 0.000000000000000000 ) ) ;
#6042=VERTEX_POINT ( 'NONE', #4676 ) ;
#6045=CARTESIAN_POINT ( 'NONE',  ( -5.940390500375658078, 6.474944468551550258, 5.000000000000004441 ) ) ;
#6047=ORIENTED_EDGE ( 'NONE', *, *, #13102, .F. ) ;
#6048=CARTESIAN_POINT ( 'NONE',  ( -3.011139120916623391, -5.190534000030277539, 23.70068193741825624 ) ) ;
#6049=VECTOR ( 'NONE', #8913, 1000.000000000000114 ) ;
#6050=CARTESIAN_POINT ( 'NONE',  ( 5.317509234263970264, -2.779225709350972906, 5.000000000000004441 ) ) ;
#6051=EDGE_CURVE ( 'NONE', #13870, #9028, #1837, .T. ) ;
#6052=B_SPLINE_CURVE_WITH_KNOTS ( 'NONE', 3,
 ( #5096, #6140, #7327, #12244, #6219, #14479, #10977, #76, #11054, #153, #5975, #5017, #2382, #1111, #9871, #3811, #8684, #3576 ),
 .UNSPECIFIED., .F., .F.,
 ( 4, 2, 2, 2, 2, 2, 2, 2, 4 ),
 ( 0.003131923598876997471, 0.003523316383094313945, 0.003914709167311630419, 0.004306101951528946460, 0.004697494735746262501, 0.005088887519963579409, 0.005480280304180895450, 0.005871673088398211490, 0.006263065872615528398 ),
 .UNSPECIFIED. ) ;
#6054=CARTESIAN_POINT ( 'NONE',  ( 0.000000000000000000, 6.250000000000000888, 12.49999999999998401 ) ) ;
#6055=CARTESIAN_POINT ( 'NONE',  ( -0.7995524673974949703, -6.199337389817277000, 12.11453679452457521 ) ) ;
#6056=CARTESIAN_POINT ( 'NONE',  ( 3.922288969639678768, 4.542045818322613115, 18.87378430870261781 ) ) ;
#6058=CARTESIAN_POINT ( 'NONE',  ( -5.317509234263906315, 2.779225709351095475, 17.99999999999998934 ) ) ;
#6059=CARTESIAN_POINT ( 'NONE',  ( 5.486982057989192363, -2.429327048029870539, 31.79931806258174376 ) ) ;
#6061=CARTESIAN_POINT ( 'NONE',  ( -4.290821322214410038, 4.545321419741521929, 30.38558052754516225 ) ) ;
#6062=CARTESIAN_POINT ( 'NONE',  ( -6.105925084677696013, 1.337450587213117048, 10.70066851092422233 ) ) ;
#6064=AXIS2_PLACEMENT_3D ( 'NONE', #10256, #5409, #6606 ) ;
#6068=CARTESIAN_POINT ( 'NONE',  ( -4.143041610105385963, 4.340967609746959610, 12.11397738943082913 ) ) ;
#6072=CARTESIAN_POINT ( 'NONE',  ( 0.5031281619707679287, 5.980084330432668516, 4.126022727445257665 ) ) ;
#6073=CARTESIAN_POINT ( 'NONE',  ( 5.903472034603481688, 2.056448723545244217, 32.00008219321556879 ) ) ;
#6078=DIRECTION ( 'NONE',  ( 0.8090169943749421222, 0.5877852522924802425, 0.000000000000000000 ) ) ;
#6083=ORIENTED_EDGE ( 'NONE', *, *, #9594, .F. ) ;
#6084=CARTESIAN_POINT ( 'NONE',  ( 5.131373506000437068, 7.062729720844210135, 24.49999999999999289 ) ) ;
#6087=CARTESIAN_POINT ( 'NONE',  ( -6.176542424588090441, 0.9554180641287481901, 24.63234125634168237 ) ) ;
#6088=CYLINDRICAL_SURFACE ( 'NONE', #5817, 1.000000000000000888 ) ;
#6089=CARTESIAN_POINT ( 'NONE',  ( 0.8738043859790753931, -6.188821459035878547, 5.503415602237494042 ) ) ;
#6090=CARTESIAN_POINT ( 'NONE',  ( -5.648559266344512331, -2.676764518775965218, 31.61396179408071916 ) ) ;
#6093=CARTESIAN_POINT ( 'NONE',  ( -0.7995524673973605223, -6.199337389817293875, 25.11453679452459298 ) ) ;
#6094=CARTESIAN_POINT ( 'NONE',  ( -2.841519077896212497, 5.566940434249979752, 11.23620383159194347 ) ) ;
#6095=CARTESIAN_POINT ( 'NONE',  ( 0.9735856429314211358, -5.920699391845005266, 18.26285283906725709 ) ) ;
#6098=B_SPLINE_CURVE_WITH_KNOTS ( 'NONE', 3,
 ( #2394, #12099, #1198, #6072, #9733, #14571, #3030, #1514, #6390, #4061, #1669, #9012, #8931, #7568, #12650, #14890, #4299, #7645 ),
 .UNSPECIFIED., .F., .F.,
 ( 4, 2, 2, 2, 2, 2, 2, 2, 4 ),
 ( 0.003131923598876998338, 0.003523316383094315246, 0.003914709167311632154, 0.004306101951528949062, 0.004697494735746265970, 0.005088887519963582878, 0.005480280304180900654, 0.005871673088398217562, 0.006263065872615534470 ),
 .UNSPECIFIED. ) ;
#6101=CARTESIAN_POINT ( 'NONE',  ( 5.329945432499600955, 2.755769831645193957, 11.23770962164069154 ) ) ;
#6102=B_SPLINE_CURVE_WITH_KNOTS ( 'NONE', 3,
 ( #8746, #1406, #2927, #530, #8907, #376, #3950, #10248, #2687, #13504, #3873, #13653, #15099, #7622, #12466, #4195, #1568, #7466 ),
 .UNSPECIFIED., .F., .F.,
 ( 4, 2, 2, 2, 2, 2, 2, 2, 4 ),
 ( 0.000000000000000000, 0.0003914898357794970615, 0.0007829796715589941230, 0.001174469507338491130, 0.001565959343117988246, 0.001957449178897485362, 0.002348939014676982261, 0.002740428850456479593, 0.003131918686235976492 ),
 .UNSPECIFIED. ) ;
#6103=EDGE_CURVE ( 'NONE', #13656, #10812, #9161, .T. ) ;
#6104=CARTESIAN_POINT ( 'NONE',  ( 5.409423237178992316, 2.597448116731069234, 31.61561732698606164 ) ) ;
#6106=EDGE_LOOP ( 'NONE', ( #6613, #14584, #6945, #11934 ) ) ;
#6109=CARTESIAN_POINT ( 'NONE',  ( -0.9999196734182004276, -5.916093360767527010, 11.36725955955069622 ) ) ;
#6110=EDGE_CURVE ( 'NONE', #9644, #5984, #10193, .T. ) ;
#6111=CARTESIAN_POINT ( 'NONE',  ( 5.317509234264027107, 2.779225709350867213, 24.49999999999999289 ) ) ;
#6112=CARTESIAN_POINT ( 'NONE',  ( 2.817313151351169331, -5.579000502529441796, 31.00000000000000000 ) ) ;
#6114=CARTESIAN_POINT ( 'NONE',  ( -3.923477796648607185, 4.541042560386401306, 10.62696220972946826 ) ) ;
#6120=CARTESIAN_POINT ( 'NONE',  ( -5.984759433607008461, 1.806271833852296282, 12.50008219321554925 ) ) ;
#6127=CARTESIAN_POINT ( 'NONE',  ( 2.082642335314403343E-14, 6.000000000000000888, 32.00000000000000000 ) ) ;
#6131=CARTESIAN_POINT ( 'NONE',  ( -3.159082487394789585, -5.393634094348327856, 12.29954462468842458 ) ) ;
#6132=EDGE_LOOP ( 'NONE', ( #7813, #9728 ) ) ;
#6139=CARTESIAN_POINT ( 'NONE',  ( 3.011899281037514697, -5.190111395030220010, 30.19977782616120621 ) ) ;
#6140=CARTESIAN_POINT ( 'NONE',  ( -0.1306171417088389242, -6.000000000000001776, 30.00000000000000000 ) ) ;
#6141=CARTESIAN_POINT ( 'NONE',  ( 5.317509234263979145, -2.779225709350955142, 31.00000000000000000 ) ) ;
#6143=CARTESIAN_POINT ( 'NONE',  ( 5.317509234263932072, 2.779225709351047957, 5.000000000000004441 ) ) ;
#6145=ORIENTED_EDGE ( 'NONE', *, *, #1759, .F. ) ;
#6146=EDGE_CURVE ( 'NONE', #1465, #14884, #14450, .T. ) ;
#6147=ORIENTED_EDGE ( 'NONE', *, *, #11241, .F. ) ;
#6148=ORIENTED_EDGE ( 'NONE', *, *, #9503, .F. ) ;
#6149=CARTESIAN_POINT ( 'NONE',  ( -4.286401442266736694, 4.198423832312983883, 24.63064961348855775 ) ) ;
#6157=CARTESIAN_POINT ( 'NONE',  ( -5.935543223013858949, 0.8771126767606857166, 31.00000000000000000 ) ) ;
#6159=DIRECTION ( 'NONE',  ( 0.5877852522924802425, -0.8090169943749422332, 0.000000000000000000 ) ) ;
#6161=CARTESIAN_POINT ( 'NONE',  ( 3.883716939929134693, -4.898343590941131254, 30.02640428276698970 ) ) ;
#6163=CARTESIAN_POINT ( 'NONE',  ( 5.616116467183593919, 2.743044348085676987, 5.504259495030093596 ) ) ;
#6167=EDGE_CURVE ( 'NONE', #15370, #4806, #3731, .T. ) ;
#6168=ORIENTED_EDGE ( 'NONE', *, *, #5940, .F. ) ;
#6169=CARTESIAN_POINT ( 'NONE',  ( -5.570820891630755334, -2.833901239560420837, 11.23763026556121858 ) ) ;
#6171=CARTESIAN_POINT ( 'NONE',  ( -2.849573632035356852, -5.280958870664559157, 25.11561732698605098 ) ) ;
#6172=CARTESIAN_POINT ( 'NONE',  ( 2.782156709077431067, -5.316215864844039629, 12.00312048902376993 ) ) ;
#6174=CARTESIAN_POINT ( 'NONE',  ( 4.153663429050693523, -4.670992970568449643, 23.70066851092423832 ) ) ;
#6175=CARTESIAN_POINT ( 'NONE',  ( -4.286401442266580375, -4.198423832313147308, 11.63061695532136852 ) ) ;
#6176=CARTESIAN_POINT ( 'NONE',  ( 5.375886393124412521, -2.665038680141230909, 12.00439760644213294 ) ) ;
#6177=CARTESIAN_POINT ( 'NONE',  ( 0.8736516769108282343, -5.936271176698213914, 17.49606771578676856 ) ) ;
#6182=CARTESIAN_POINT ( 'NONE',  ( 5.935543223013858061, 0.8771126767606804986, 11.36935038651144581 ) ) ;
#6184=AXIS2_PLACEMENT_3D ( 'NONE', #10468, #992, #8321 ) ;
#6185=ORIENTED_EDGE ( 'NONE', *, *, #7306, .T. ) ;
#6186=CARTESIAN_POINT ( 'NONE',  ( -3.312341048453451009, 5.004306261885466789, 4.026019798777604741 ) ) ;
#6188=CARTESIAN_POINT ( 'NONE',  ( 6.768587589771821120E-14, -6.000000000000000888, 12.49999999999998401 ) ) ;
#6190=CARTESIAN_POINT ( 'NONE',  ( 2.031800924177950305E-13, 6.000000000000000888, 23.49999999999999289 ) ) ;
#6192=DIRECTION ( 'NONE',  ( -0.9510565162951544194, 0.3090169943749447312, 0.000000000000000000 ) ) ;
#6193=EDGE_CURVE ( 'NONE', #12811, #2830, #13589, .T. ) ;
#6195=CARTESIAN_POINT ( 'NONE',  ( 5.330189595673641811, -2.755293208590234411, 4.736173967944048435 ) ) ;
#6199=CARTESIAN_POINT ( 'NONE',  ( 0.000000000000000000, 0.000000000000000000, 53.67766952966368876 ) ) ;
#6202=CARTESIAN_POINT ( 'NONE',  ( 6.172651332693102511, 0.9815532474593232637, 17.73809786915987274 ) ) ;
#6206=CARTESIAN_POINT ( 'NONE',  ( 5.620786884546339124, 2.102685372472758552, 23.52641404563304661 ) ) ;
#6207=CARTESIAN_POINT ( 'NONE',  ( 3.253823204785117440, 5.337590213880504919, 30.12694108445699825 ) ) ;
#6209=VECTOR ( 'NONE', #2108, 1000.000000000000000 ) ;
#6211=EDGE_CURVE ( 'NONE', #11236, #5801, #9773, .T. ) ;
#6212=CARTESIAN_POINT ( 'NONE',  ( 0.8002720181892983842, -6.199262377003380564, 23.88606262465556185 ) ) ;
#6213=ADVANCED_FACE ( 'NONE', ( #3707 ), #8584, .F. ) ;
#6219=CARTESIAN_POINT ( 'NONE',  ( -0.6144377077729746839, -5.969178481556069116, 30.20033966857736729 ) ) ;
#6222=CARTESIAN_POINT ( 'NONE',  ( -5.783239563508424830, 1.602707436861116497, 10.52641404563305194 ) ) ;
#6223=CARTESIAN_POINT ( 'NONE',  ( -6.081464507797636365, 1.446657058464182022, 10.62619944752603018 ) ) ;
#6224=CARTESIAN_POINT ( 'NONE',  ( 3.419318284370060912, 4.932111238568271716, 23.50007997643737312 ) ) ;
#6226=EDGE_LOOP ( 'NONE', ( #11301, #9563, #3057, #3446 ) ) ;
#6228=EDGE_LOOP ( 'NONE', ( #11720, #10867, #14671, #13989 ) ) ;
#6229=DIRECTION ( 'NONE',  ( 0.000000000000000000, 0.000000000000000000, 1.000000000000000000 ) ) ;
#6237=CARTESIAN_POINT ( 'NONE',  ( -5.620879908643987122, 2.102487719021844281, 31.97377823943293151 ) ) ;
#6238=CARTESIAN_POINT ( 'NONE',  ( 4.141923667210698490, -4.342011609040415721, 31.61561732698606875 ) ) ;
#6240=CARTESIAN_POINT ( 'NONE',  ( -6.176542424588117086, 0.9554180641285661135, 30.86762589283693359 ) ) ;
#6242=ORIENTED_EDGE ( 'NONE', *, *, #4228, .F. ) ;
#6243=ORIENTED_EDGE ( 'NONE', *, *, #7106, .T. ) ;
#6246=CARTESIAN_POINT ( 'NONE',  ( -7.490007020835642848, -2.433650805992559896, 24.49999999999999289 ) ) ;
#6249=CARTESIAN_POINT ( 'NONE',  ( -0.8738118504725720381, -5.936246475285030577, 5.503572421742426890 ) ) ;
#6250=CARTESIAN_POINT ( 'NONE',  ( -3.312341048453484316, -5.004306261885444584, 18.97398020122238904 ) ) ;
#6251=CARTESIAN_POINT ( 'NONE',  ( 0.7988914244718910984, 5.947301735519275212, 10.88456289168616742 ) ) ;
#6253=EDGE_CURVE ( 'NONE', #10136, #7716, #13259, .T. ) ;
#6254=FACE_OUTER_BOUND ( 'NONE', #8131, .T. ) ;
#6255=CARTESIAN_POINT ( 'NONE',  ( -6.021167129161060672, -1.680051667990286601, 5.973595717233013858 ) ) ;
#6256=CARTESIAN_POINT ( 'NONE',  ( 0.5039079366034465712, -5.980031194523134808, 23.62637068109812333 ) ) ;
#6264=CARTESIAN_POINT ( 'NONE',  ( 6.780834054130108014E-14, -6.250000000000000888, 10.49999999999998224 ) ) ;
#6265=CARTESIAN_POINT ( 'NONE',  ( 5.843318061569079624, 1.367618216965494238, 25.37303779027051576 ) ) ;
#6266=CARTESIAN_POINT ( 'NONE',  ( 5.770288754215121330, 2.404361317819969646, 12.37381964045070504 ) ) ;
#6270=CARTESIAN_POINT ( 'NONE',  ( 4.435347140101010055, 4.403429997944536822, 5.000000000000004441 ) ) ;
#6278=VERTEX_POINT ( 'NONE', #8660 ) ;
#6281=CARTESIAN_POINT ( 'NONE',  ( 5.984377695197274249, -1.807429553002113609, 19.00004906876531408 ) ) ;
#6283=ORIENTED_EDGE ( 'NONE', *, *, #11, .T. ) ;
#6284=CARTESIAN_POINT ( 'NONE',  ( -3.107688324358802490, -5.133887830459779700, 23.62621569129737864 ) ) ;
#6285=CARTESIAN_POINT ( 'NONE',  ( 6.176542424588128632, -0.9554180641284775177, 11.49999999999998224 ) ) ;
#6287=AXIS2_PLACEMENT_3D ( 'NONE', #1169, #10883, #3475 ) ;
#6288=CARTESIAN_POINT ( 'NONE',  ( 0.6144300524834573896, 6.220417338033042753, 10.70033372175934439 ) ) ;
#6293=CARTESIAN_POINT ( 'NONE',  ( 5.330189595673669345, -2.755293208590180232, 11.23617396794405288 ) ) ;
#6294=CARTESIAN_POINT ( 'NONE',  ( -0.7988860301920965856, -6.199427171881353615, 17.38455580536194489 ) ) ;
#6296=CARTESIAN_POINT ( 'NONE',  ( -5.317509234263959605, 2.779225709350992002, 31.00000000000000000 ) ) ;
#6301=EDGE_CURVE ( 'NONE', #1760, #5982, #15688, .T. ) ;
#6305=CARTESIAN_POINT ( 'NONE',  ( -4.196038884587333762, 4.289036423669111642, 25.00389795015983552 ) ) ;
#6307=VERTEX_POINT ( 'NONE', #6583 ) ;
#6315=CARTESIAN_POINT ( 'NONE',  ( -5.486741141153809842, 2.429871531109698335, 31.79888242247943353 ) ) ;
#6318=CARTESIAN_POINT ( 'NONE',  ( -6.176542424588117974, 0.9554180641285661135, 31.00000000000000000 ) ) ;
#6321=ORIENTED_EDGE ( 'NONE', *, *, #11273, .T. ) ;
#6322=EDGE_LOOP ( 'NONE', ( #5906, #7118, #7811, #3388 ) ) ;
#6324=CYLINDRICAL_SURFACE ( 'NONE', #13337, 1.000000000000000888 ) ;
#6325=CARTESIAN_POINT ( 'NONE',  ( 2.930600586412970276, 5.520563544161749547, 4.496913561339538568 ) ) ;
#6326=EDGE_LOOP ( 'NONE', ( #4611, #8516, #5494, #8336 ) ) ;
#6327=CARTESIAN_POINT ( 'NONE',  ( 0.6144300524833581356, 6.220417338033051635, 4.200333721759339944 ) ) ;
#6329=CARTESIAN_POINT ( 'NONE',  ( 0.8002720181892442053, -6.199262377003387670, 17.38606262465557606 ) ) ;
#6330=CARTESIAN_POINT ( 'NONE',  ( 3.568242062701445949, -5.132954954975562423, 23.49995093123466461 ) ) ;
#6333=CARTESIAN_POINT ( 'NONE',  ( 5.843075991566598404, -1.368655265450984704, 12.37364704684421035 ) ) ;
#6334=CARTESIAN_POINT ( 'NONE',  ( -3.158825713737648755, 5.393784879207071725, 18.79933148907576168 ) ) ;
#6341=EDGE_CURVE ( 'NONE', #13293, #4150, #11898, .T. ) ;
#6343=CARTESIAN_POINT ( 'NONE',  ( -5.859221468178952286, 2.178708437343215731, 17.02591457665827690 ) ) ;
#6344=B_SPLINE_CURVE_WITH_KNOTS ( 'NONE', 3,
 ( #8154, #9046, #4489, #10382, #10305, #4253, #14184, #5459, #11722, #3290, #747, #2091, #10460, #4416, #1860, #5613, #15233, #9269 ),
 .UNSPECIFIED., .F., .F.,
 ( 4, 2, 2, 2, 2, 2, 2, 2, 4 ),
 ( 0.000000000000000000, 0.0003914362731607522075, 0.0007828725463215044150, 0.001174308819482256568, 0.001565745092643008830, 0.001957181365803761092, 0.002348617638964513137, 0.002740053912125265615, 0.003131490185286017660 ),
 .UNSPECIFIED. ) ;
#6345=CARTESIAN_POINT ( 'NONE',  ( 3.254737477228021536, -5.337033878705195633, 10.62632671364005432 ) ) ;
#6347=CARTESIAN_POINT ( 'NONE',  ( -4.006441409774867957, 4.467329318258094872, 23.70111757752058068 ) ) ;
#6348=CARTESIAN_POINT ( 'NONE',  ( 0.8730424326982959560, 5.936362132114433976, 23.99500690218563648 ) ) ;
#6349=AXIS2_PLACEMENT_3D ( 'NONE', #15513, #3405, #8197 ) ;
#6351=EDGE_CURVE ( 'NONE', #7562, #7176, #15321, .T. ) ;
#6352=CARTESIAN_POINT ( 'NONE',  ( -2.817313151351126255, -5.579000502529464889, 31.13234125634170368 ) ) ;
#6354=CARTESIAN_POINT ( 'NONE',  ( -3.781065399486156497, 4.978303713186331692, 23.50008258189710020 ) ) ;
#6355=CARTESIAN_POINT ( 'NONE',  ( 5.843318061569033439, 1.367618216965686972, 5.873037790270514868 ) ) ;
#6360=CARTESIAN_POINT ( 'NONE',  ( 3.159612573729187357, 5.393342049074656863, 12.30026515017674882 ) ) ;
#6361=AXIS2_PLACEMENT_3D ( 'NONE', #5692, #10537, #6657 ) ;
#6364=CARTESIAN_POINT ( 'NONE',  ( -3.420659742068490328, 4.931142898501661875, 18.99995053646221521 ) ) ;
#6366=ORIENTED_EDGE ( 'NONE', *, *, #2340, .F. ) ;
#6367=CARTESIAN_POINT ( 'NONE',  ( -4.435347140101107755, -4.403429997944436458, 17.99999999999998934 ) ) ;
#6369=CARTESIAN_POINT ( 'NONE',  ( 5.616089948629760187, -2.743103014345478652, 12.00436969680152721 ) ) ;
#6371=CARTESIAN_POINT ( 'NONE',  ( -5.666074146198027961, 1.978051345703067065, 3.999950679266886855 ) ) ;
#6372=CARTESIAN_POINT ( 'NONE',  ( -0.2637975869347151114, -6.245592211692898132, 12.47332839949189598 ) ) ;
#6373=CARTESIAN_POINT ( 'NONE',  ( 5.931828553038004159, -0.9033193133617308801, 24.76194324003146008 ) ) ;
#6375=DIRECTION ( 'NONE',  ( -0.5877852522924685852, -0.8090169943749508930, 0.000000000000000000 ) ) ;
#6378=CARTESIAN_POINT ( 'NONE',  ( -5.783239563508395520, -1.602707436861224632, 12.47358595436692319 ) ) ;
#6380=EDGE_LOOP ( 'NONE', ( #3441, #10748, #2372, #10459 ) ) ;
#6385=CARTESIAN_POINT ( 'NONE',  ( -5.666074146197935590, -1.978051345703340180, 25.50004932073311892 ) ) ;
#6386=DIRECTION ( 'NONE',  ( 0.000000000000000000, 0.000000000000000000, 1.000000000000000000 ) ) ;
#6387=ORIENTED_EDGE ( 'NONE', *, *, #78, .F. ) ;
#6388=B_SPLINE_CURVE_WITH_KNOTS ( 'NONE', 3,
 ( #14638, #14716, #5888, #12001, #69, #7164, #1024, #1106, #3647, #10813, #9865, #5969, #6212, #2541, #14473, #2294, #1337, #11048 ),
 .UNSPECIFIED., .F., .F.,
 ( 4, 2, 2, 2, 2, 2, 2, 2, 4 ),
 ( 0.000000000000000000, 0.0003914362731607616401, 0.0007828725463215232801, 0.001174308819482284974, 0.001565745092643046560, 0.001957181365803808363, 0.002348617638964569949, 0.002740053912125331535, 0.003131490185286093120 ),
 .UNSPECIFIED. ) ;
#6390=CARTESIAN_POINT ( 'NONE',  ( 0.9999196734182647095, 5.916093360767514575, 4.867259559550685566 ) ) ;
#6394=ADVANCED_FACE ( 'NONE', ( #13640, #5313, #2756, #7607, #15482, #5619, #15399, #7997, #11802, #9275, #2174, #5697, #4495, #15558, #5774, #12759, #14037, #667, #6894, #906, #11570, #9349, #12920, #15320, #15239, #3145 ), #10541, .T. ) ;
#6399=EDGE_CURVE ( 'NONE', #14733, #15393, #2020, .T. ) ;
#6400=DIRECTION ( 'NONE',  ( -0.9510565162951544194, 0.3090169943749447312, 0.000000000000000000 ) ) ;
#6401=CARTESIAN_POINT ( 'NONE',  ( -0.1323736289504332531, 6.250000000000000888, 32.00000000000000000 ) ) ;
#6402=VERTEX_POINT ( 'NONE', #6816 ) ;
#6404=ORIENTED_EDGE ( 'NONE', *, *, #6211, .F. ) ;
#6405=CARTESIAN_POINT ( 'NONE',  ( 0.6156307853270768238, 5.969051238897241873, 18.79870573410680379 ) ) ;
#6408=CARTESIAN_POINT ( 'NONE',  ( 0.7995524673975749064, 6.199337389817269006, 5.614536794524586760 ) ) ;
#6411=CARTESIAN_POINT ( 'NONE',  ( -5.131373506000731055, 7.062729720844018289, 31.00000000000000000 ) ) ;
#6412=CARTESIAN_POINT ( 'NONE',  ( 5.558508435838239059, -2.857531096718835872, 30.86765874365832119 ) ) ;
#6415=CARTESIAN_POINT ( 'NONE',  ( 5.531796221294904115, -2.326749136277146857, 12.37378430870260537 ) ) ;
#6416=CARTESIAN_POINT ( 'NONE',  ( 3.010624175977925532, 5.190832888732251682, 10.70111757752057002 ) ) ;
#6423=ORIENTED_EDGE ( 'NONE', *, *, #2829, .F. ) ;
#6424=CARTESIAN_POINT ( 'NONE',  ( -7.799024015210657801, -1.482594289697236389, 31.00000000000000000 ) ) ;
#6425=B_SPLINE_CURVE_WITH_KNOTS ( 'NONE', 3,
 ( #9687, #13562, #12529, #1783, #8730, #6347, #11182, #14847, #9999, #281, #1629, #2833, #5067, #7838, #9048, #11103, #13799, #8808 ),
 .UNSPECIFIED., .F., .F.,
 ( 4, 2, 2, 2, 2, 2, 2, 2, 4 ),
 ( 0.003131918686235977793, 0.003523310662250268063, 0.003914702638264558332, 0.004306094614278849035, 0.004697486590293138004, 0.005088878566307427839, 0.005480270542321717675, 0.005871662518336007511, 0.006263054494350296479 ),
 .UNSPECIFIED. ) ;
#6426=CYLINDRICAL_SURFACE ( 'NONE', #13713, 1.000000000000000666 ) ;
#6428=CARTESIAN_POINT ( 'NONE',  ( 0.7995298244856630099, 5.947211616899221731, 25.11456014619858124 ) ) ;
#6431=B_SPLINE_CURVE_WITH_KNOTS ( 'NONE', 3,
 ( #3921, #3845, #13627, #2505, #2820, #14599, #14912, #5053, #4979, #12517, #3690, #4003, #270, #8881, #11170, #6094, #5133, #14835 ),
 .UNSPECIFIED., .F., .F.,
 ( 4, 2, 2, 2, 2, 2, 2, 2, 4 ),
 ( 0.003131486019302005472, 0.003522824630466710009, 0.003914163241631414547, 0.004305501852796118217, 0.004696840463960822755, 0.005088179075125527293, 0.005479517686290230963, 0.005870856297454935500, 0.006262194908619640038 ),
 .UNSPECIFIED. ) ;
#6434=CARTESIAN_POINT ( 'NONE',  ( -4.154121946521065922, 4.670585111242799847, 23.70112161576661336 ) ) ;
#6444=CARTESIAN_POINT ( 'NONE',  ( -3.107688324358827803, 5.133887830459763713, 18.87378430870261781 ) ) ;
#6452=CARTESIAN_POINT ( 'NONE',  ( 5.665824935993679645, -1.978765057080718481, 25.49995053646222232 ) ) ;
#6457=DIRECTION ( 'NONE',  ( -0.5877852522924685852, -0.8090169943749507819, 0.000000000000000000 ) ) ;
#6459=CARTESIAN_POINT ( 'NONE',  ( 4.286401442266388528, 4.198423832313340043, 24.49999999999999289 ) ) ;
#6460=VERTEX_POINT ( 'NONE', #3066 ) ;
#6462=VECTOR ( 'NONE', #4428, 1000.000000000000114 ) ;
#6463=ORIENTED_EDGE ( 'NONE', *, *, #9693, .T. ) ;
#6464=CARTESIAN_POINT ( 'NONE',  ( -5.935543223013818981, -0.8771126767609508379, 24.36763921416088863 ) ) ;
#6465=VERTEX_POINT ( 'NONE', #2099 ) ;
#6466=CARTESIAN_POINT ( 'NONE',  ( -5.531623157106079880, -2.327208526676637579, 25.37364704684422634 ) ) ;
#6470=CARTESIAN_POINT ( 'NONE',  ( -0.9740807849834816068, 5.920620690450712154, 17.73850119700669126 ) ) ;
#6472=CARTESIAN_POINT ( 'NONE',  ( -7.490007020835642848, -2.433650805992559896, 24.49999999999999289 ) ) ;
#6475=CARTESIAN_POINT ( 'NONE',  ( 3.010624175978041883, -5.190832888732185957, 31.79888242247942642 ) ) ;
#6477=DIRECTION ( 'NONE',  ( -0.3090169943749584425, 0.9510565162951498674, 0.000000000000000000 ) ) ;
#6478=CARTESIAN_POINT ( 'NONE',  ( 4.286401442266483564, 4.198423832313243231, 11.63239388001634289 ) ) ;
#6480=ORIENTED_EDGE ( 'NONE', *, *, #12636, .F. ) ;
#6482=CARTESIAN_POINT ( 'NONE',  ( 5.867109477881242263, -1.259218163100928267, 30.20111757752059489 ) ) ;
#6485=CARTESIAN_POINT ( 'NONE',  ( 0.9999171162589708395, 6.169494774098548184, 4.867223203306743073 ) ) ;
#6486=CARTESIAN_POINT ( 'NONE',  ( 6.176542424588140179, -0.9554180641284089059, 17.99999999999998934 ) ) ;
#6487=AXIS2_PLACEMENT_3D ( 'NONE', #1755, #636, #4225 ) ;
#6489=CARTESIAN_POINT ( 'NONE',  ( 5.985119669071122139, -1.805077827356540432, 30.00008258189710730 ) ) ;
#6491=SURFACE_STYLE_USAGE ( .BOTH. , #2739 ) ;
#6498=EDGE_CURVE ( 'NONE', #5516, #11747, #9510, .T. ) ;
#6500=B_SPLINE_CURVE_WITH_KNOTS ( 'NONE', 3,
 ( #2053, #10498, #13030, #13108, #5574, #8195, #12791, #14065, #5496, #9463, #4449, #12952, #12869, #10340, #10571, #3099, #8271, #11602 ),
 .UNSPECIFIED., .F., .F.,
 ( 4, 2, 2, 2, 2, 2, 2, 2, 4 ),
 ( 0.000000000000000000, 0.0003914904498596246296, 0.0007829808997192490424, 0.001174471349578873293, 0.001565961799438497868, 0.001957452249298122227, 0.002348942699157746585, 0.002740433149017371811, 0.003131923598876996170 ),
 .UNSPECIFIED. ) ;
#6501=ORIENTED_EDGE ( 'NONE', *, *, #939, .T. ) ;
#6503=CARTESIAN_POINT ( 'NONE',  ( -2.849269941561985764, 5.281123252784034605, 5.615193824488510010 ) ) ;
#6505=CARTESIAN_POINT ( 'NONE',  ( 0.8736772044960799954, -6.188841968496048729, 10.99611573292812672 ) ) ;
#6508=CARTESIAN_POINT ( 'NONE',  ( 3.568242062701532546, 5.132954954975506467, 6.000049068765333615 ) ) ;
#6510=CARTESIAN_POINT ( 'NONE',  ( 3.419318284370227445, 4.932111238568157141, 4.000079976437387330 ) ) ;
#6517=CARTESIAN_POINT ( 'NONE',  ( -4.435347140101057128, -4.403429997944488861, 11.36936067245786219 ) ) ;
#6520=CARTESIAN_POINT ( 'NONE',  ( 6.081590040723110491, -1.446205118472867923, 18.87367328635991726 ) ) ;
#6522=VERTEX_POINT ( 'NONE', #14263 ) ;
#6523=DIRECTION ( 'NONE',  ( -0.3090169943749584425, 0.9510565162951498674, 0.000000000000000000 ) ) ;
#6524=CARTESIAN_POINT ( 'NONE',  ( 6.172651332693103399, -0.9815532474593076095, 11.76190213084010239 ) ) ;
#6525=CARTESIAN_POINT ( 'NONE',  ( -5.915653884842720700, 1.003805156977363833, 4.495602393557862619 ) ) ;
#6527=LINE ( 'NONE', #11362, #4278 ) ;
#6529=CARTESIAN_POINT ( 'NONE',  ( 3.106366801612069573, -5.134708448381242185, 5.873037790270517533 ) ) ;
#6530=CARTESIAN_POINT ( 'NONE',  ( 6.081836621194488757, -1.445163676684627641, 23.62694108445698760 ) ) ;
#6532=CARTESIAN_POINT ( 'NONE',  ( -5.531209434046302498, -2.328189801702702511, 10.62696220972947003 ) ) ;
#6533=EDGE_LOOP ( 'NONE', ( #12075, #1428 ) ) ;
#6536=DIRECTION ( 'NONE',  ( -0.9510565162951545304, 0.3090169943749447867, 0.000000000000000000 ) ) ;
#6537=ORIENTED_EDGE ( 'NONE', *, *, #8094, .T. ) ;
#6538=EDGE_CURVE ( 'NONE', #10984, #8231, #10750, .T. ) ;
#6545=CARTESIAN_POINT ( 'NONE',  ( -0.9999502950800709389, 5.916088184763905744, 18.13108149190012597 ) ) ;
#6550=LINE ( 'NONE', #11309, #12064 ) ;
#6552=CARTESIAN_POINT ( 'NONE',  ( -0.9740856415300650495, 6.173834621338596840, 30.73852653055532613 ) ) ;
#6553=EDGE_LOOP ( 'NONE', ( #12113, #11059 ) ) ;
#6554=ORIENTED_EDGE ( 'NONE', *, *, #8097, .T. ) ;
#6555=VERTEX_POINT ( 'NONE', #3535 ) ;
#6556=CARTESIAN_POINT ( 'NONE',  ( -5.903061651806586596, -2.057626436184838870, 10.50008258189709132 ) ) ;
#6561=CARTESIAN_POINT ( 'NONE',  ( -5.558508435838126260, -2.857531096719055252, 17.99999999999998934 ) ) ;
#6562=CARTESIAN_POINT ( 'NONE',  ( 0.6139731865241387920, -6.220476368274037604, 17.19975545601932865 ) ) ;
#6564=CARTESIAN_POINT ( 'NONE',  ( -0.9735954530124010242, 6.173909381474013358, 18.26281793585238233 ) ) ;
#6565=CARTESIAN_POINT ( 'NONE',  ( 0.7995524673976397434, 6.199337389817260124, 18.61453679452466403 ) ) ;
#6568=CARTESIAN_POINT ( 'NONE',  ( 3.633127580202213380, 4.776802569231102247, 10.49992038825521590 ) ) ;
#6576=ORIENTED_EDGE ( 'NONE', *, *, #3749, .F. ) ;
#6577=CARTESIAN_POINT ( 'NONE',  ( -3.107688324358700349, 5.133887830459841872, 5.873784308702619583 ) ) ;
#6578=CARTESIAN_POINT ( 'NONE',  ( 2.996417732210587381, -5.485687819086892958, 10.88603820591927196 ) ) ;
#6579=CARTESIAN_POINT ( 'NONE',  ( -0.5039005892421214439, 6.230833003620541710, 4.126363889112979244 ) ) ;
#6580=CARTESIAN_POINT ( 'NONE',  ( 5.570760634536775058, 2.834026536768299298, 30.73774718278284013 ) ) ;
#6581=CYLINDRICAL_SURFACE ( 'NONE', #2583, 1.000000000000000444 ) ;
#6583=CARTESIAN_POINT ( 'NONE',  ( -5.317509234263930296, -2.779225709351048401, 5.000000000000004441 ) ) ;
#6586=CARTESIAN_POINT ( 'NONE',  ( -3.567624405365240836, -5.133384272590781450, 30.00004921015706572 ) ) ;
#6591=FACE_BOUND ( 'NONE', #7894, .T. ) ;
#6595=CARTESIAN_POINT ( 'NONE',  ( 5.770331821586463406, -2.404225004693450352, 18.87380055247394850 ) ) ;
#6597=ORIENTED_EDGE ( 'NONE', *, *, #9514, .F. ) ;
#6598=CARTESIAN_POINT ( 'NONE',  ( -2.849269941562030173, -5.281123252784012401, 17.38480617551148200 ) ) ;
#6602=EDGE_CURVE ( 'NONE', #1820, #14280, #13231, .T. ) ;
#6606=DIRECTION ( 'NONE',  ( 0.8090169943749421222, 0.5877852522924802425, 0.000000000000000000 ) ) ;
#6607=CARTESIAN_POINT ( 'NONE',  ( -0.2622916576876348493, 5.995491482261827265, 31.97384942646813855 ) ) ;
#6608=CARTESIAN_POINT ( 'NONE',  ( 3.311576095066638636, -5.004818610361268405, 5.973778239432936843 ) ) ;
#6609=CARTESIAN_POINT ( 'NONE',  ( 6.081590040723080293, -1.446205118472996931, 5.873673286359928802 ) ) ;
#6610=CARTESIAN_POINT ( 'NONE',  ( 2.094888807778566729E-14, 6.000000000000000888, 30.00000000000000000 ) ) ;
#6611=CARTESIAN_POINT ( 'NONE',  ( -7.490007020835664164, -2.433650805992495503, 17.99999999999998934 ) ) ;
#6612=EDGE_CURVE ( 'NONE', #6278, #4624, #3450, .T. ) ;
#6613=ORIENTED_EDGE ( 'NONE', *, *, #14246, .F. ) ;
#6616=DIRECTION ( 'NONE',  ( -0.5877852522924685852, -0.8090169943749507819, 0.000000000000000000 ) ) ;
#6618=ORIENTED_EDGE ( 'NONE', *, *, #14471, .F. ) ;
#6619=FACE_OUTER_BOUND ( 'NONE', #6687, .T. ) ;
#6621=ORIENTED_EDGE ( 'NONE', *, *, #14856, .T. ) ;
#6623=CARTESIAN_POINT ( 'NONE',  ( -4.435347140101074004, 4.403429997944469321, 5.000000000000004441 ) ) ;
#6624=FACE_OUTER_BOUND ( 'NONE', #1372, .T. ) ;
#6627=CARTESIAN_POINT ( 'NONE',  ( -3.420659742068348219, -4.931142898501759575, 10.50004946353775637 ) ) ;
#6629=CARTESIAN_POINT ( 'NONE',  ( 7.490007020835748541, -2.433650805992050969, 24.49999999999999289 ) ) ;
#6631=EDGE_CURVE ( 'NONE', #13293, #2588, #9829, .T. ) ;
#6634=ORIENTED_EDGE ( 'NONE', *, *, #13896, .F. ) ;
#6638=CARTESIAN_POINT ( 'NONE',  ( 3.253823204785158296, -5.337590213880479162, 12.37305891554298931 ) ) ;
#6639=CARTESIAN_POINT ( 'NONE',  ( 5.770331821586379029, 2.404225004693657297, 4.126199447526043507 ) ) ;
#6642=CARTESIAN_POINT ( 'NONE',  ( -3.458467055437286053, 5.207305717053834826, 31.97359571723301741 ) ) ;
#6653=EDGE_LOOP ( 'NONE', ( #12986, #11392 ) ) ;
#6654=CARTESIAN_POINT ( 'NONE',  ( 3.312524433819890035, -5.004191858253928871, 4.025919472168997260 ) ) ;
#6656=CARTESIAN_POINT ( 'NONE',  ( -3.781065399486098322, 4.978303713186375212, 17.00008258189709309 ) ) ;
#6657=DIRECTION ( 'NONE',  ( -0.3090169943749447867, -0.9510565162951544194, 0.000000000000000000 ) ) ;
#6661=CARTESIAN_POINT ( 'NONE',  ( 4.290381260516283213, 4.545736887716198105, 5.615177803758427899 ) ) ;
#6664=CARTESIAN_POINT ( 'NONE',  ( 4.141923667210649640, 4.342011609040460129, 4.384382673013946352 ) ) ;
#6666=CARTESIAN_POINT ( 'NONE',  ( -3.458467055437213666, -5.207305717053880123, 30.02640428276698259 ) ) ;
#6669=DIRECTION ( 'NONE',  ( 0.000000000000000000, 0.000000000000000000, -1.000000000000000000 ) ) ;
#6670=CARTESIAN_POINT ( 'NONE',  ( 6.176542424588121527, -0.9554180641285238140, 31.00000000000000000 ) ) ;
#6673=CARTESIAN_POINT ( 'NONE',  ( -2.931156713028654437, 5.520271803279126033, 25.00436969680153965 ) ) ;
#6675=EDGE_LOOP ( 'NONE', ( #10608, #6145, #2357, #7425 ) ) ;
#6677=CARTESIAN_POINT ( 'NONE',  ( 6.123233995736766282E-16, -6.250000000000000888, 6.000000000000004441 ) ) ;
#6678=CARTESIAN_POINT ( 'NONE',  ( 4.267936573529090616, 4.217499624512361045, 24.76229037835931734 ) ) ;
#6679=CARTESIAN_POINT ( 'NONE',  ( -5.329907877631393731, 2.755840666746176559, 4.738056759968538145 ) ) ;
#6680=CARTESIAN_POINT ( 'NONE',  ( 0.000000000000000000, 0.000000000000000000, 0.000000000000000000 ) ) ;
#6682=CARTESIAN_POINT ( 'NONE',  ( -5.317509234263931184, -2.779225709351047957, 5.130649613488544425 ) ) ;
#6684=CARTESIAN_POINT ( 'NONE',  ( -3.736532060718004811, 4.696070028785960027, 30.02622176056705428 ) ) ;
#6687=EDGE_LOOP ( 'NONE', ( #2494, #14256, #2246, #6987 ) ) ;
#6689=ORIENTED_EDGE ( 'NONE', *, *, #9503, .T. ) ;
#6690=CARTESIAN_POINT ( 'NONE',  ( 2.668367453516610865, 5.373994336898140212, 31.00000000000000000 ) ) ;
#6692=ORIENTED_EDGE ( 'NONE', *, *, #13374, .F. ) ;
#6694=DIRECTION ( 'NONE',  ( 0.9510565162951500895, 0.3090169943749582204, 0.000000000000000000 ) ) ;
#6695=ADVANCED_FACE ( 'NONE', ( #13766 ), #7647, .F. ) ;
#6699=ADVANCED_FACE ( 'NONE', ( #13532 ), #10042, .F. ) ;
#6700=CARTESIAN_POINT ( 'NONE',  ( -0.2622916576875202743, 5.995491482261835259, 18.97384942646813144 ) ) ;
#6701=CARTESIAN_POINT ( 'NONE',  ( -2.817313151351109823, -5.579000502529473771, 5.132341256341692137 ) ) ;
#6704=CARTESIAN_POINT ( 'NONE',  ( -2.668367453516831134, 5.373994336898032742, 17.86763921416087797 ) ) ;
#6706=CARTESIAN_POINT ( 'NONE',  ( -5.931734679891428108, -0.9039278060245539148, 17.73617396794403689 ) ) ;
#6709=ORIENTED_EDGE ( 'NONE', *, *, #15476, .T. ) ;
#6710=ORIENTED_EDGE ( 'NONE', *, *, #14093, .F. ) ;
#6712=CARTESIAN_POINT ( 'NONE',  ( 3.253823204785093459, -5.337590213880519130, 18.87305891554299464 ) ) ;
#6713=LINE ( 'NONE', #11704, #7086 ) ;
#6714=EDGE_LOOP ( 'NONE', ( #4276, #2322, #9025, #5107 ) ) ;
#6716=VECTOR ( 'NONE', #2458, 1000.000000000000114 ) ;
#6718=CARTESIAN_POINT ( 'NONE',  ( -5.935543223013843850, -0.8771126767607685393, 31.00000000000000000 ) ) ;
#6721=CARTESIAN_POINT ( 'NONE',  ( 5.903347812666364547, -1.076697810262513322, 12.11397738943082736 ) ) ;
#6724=FACE_BOUND ( 'NONE', #13051, .T. ) ;
#6728=CARTESIAN_POINT ( 'NONE',  ( 3.568242062701418416, 5.132954954975583739, 19.00004906876532118 ) ) ;
#6733=CARTESIAN_POINT ( 'NONE',  ( -3.159082487394895722, 5.393634094348264796, 17.20045537531157365 ) ) ;
#6735=CARTESIAN_POINT ( 'NONE',  ( 6.081590040723103385, 1.446205118472900786, 23.62632671364005787 ) ) ;
#6737=DIRECTION ( 'NONE',  ( 0.8090169943749510040, -0.5877852522924683631, 0.000000000000000000 ) ) ;
#6738=DIRECTION ( 'NONE',  ( 0.000000000000000000, 0.000000000000000000, -1.000000000000000000 ) ) ;
#6741=CARTESIAN_POINT ( 'NONE',  ( 3.735808404764980661, 4.696639218303141128, 4.026019798777603853 ) ) ;
#6745=AXIS2_PLACEMENT_3D ( 'NONE', #10202, #7965, #2880 ) ;
#6747=FACE_OUTER_BOUND ( 'NONE', #138, .T. ) ;
#6748=CARTESIAN_POINT ( 'NONE',  ( 0.9737725088284505670, 6.173885267451787229, 24.23735758726573053 ) ) ;
#6751=CARTESIAN_POINT ( 'NONE',  ( -2.841041022017575468, 5.567186575787166802, 24.76225281721715987 ) ) ;
#6752=CARTESIAN_POINT ( 'NONE',  ( -0.1323602877610131345, -6.000000000000007105, 25.49999999999999645 ) ) ;
#6753=ORIENTED_EDGE ( 'NONE', *, *, #14160, .T. ) ;
#6756=CARTESIAN_POINT ( 'NONE',  ( 5.665707375537505364, -1.979196487016587014, 16.99992038825522656 ) ) ;
#6760=B_SPLINE_CURVE_WITH_KNOTS ( 'NONE', 3,
 ( #4106, #7920, #14929, #4021, #13805, #12842, #4343, #12692, #6510, #11654, #6741, #15014, #9131, #6664, #3147, #5233, #1867, #2914 ),
 .UNSPECIFIED., .F., .F.,
 ( 4, 2, 2, 2, 2, 2, 2, 2, 4 ),
 ( 0.003131918686235953941, 0.003523310662250245945, 0.003914702638264537515, 0.004306094614278829953, 0.004697486590293121524, 0.005088878566307413961, 0.005480270542321705532, 0.005871662518335997102, 0.006263054494350289540 ),
 .UNSPECIFIED. ) ;
#6761=DIRECTION ( 'NONE',  ( -0.3090169943749447867, -0.9510565162951544194, 0.000000000000000000 ) ) ;
#6762=FACE_OUTER_BOUND ( 'NONE', #3679, .T. ) ;
#6764=CARTESIAN_POINT ( 'NONE',  ( 6.176542424588148172, -0.9554180641283416264, 24.36939309276500509 ) ) ;
#6771=CARTESIAN_POINT ( 'NONE',  ( 2.082642335314403343E-14, -6.250000000000000888, 31.00000000000000000 ) ) ;
#6772=CARTESIAN_POINT ( 'NONE',  ( -4.005361199354941171, -4.468319061418822180, 4.199777826161208871 ) ) ;
#6773=CARTESIAN_POINT ( 'NONE',  ( -3.011385983131281030, -5.190390249166461523, 5.799520541027148646 ) ) ;
#6782=CARTESIAN_POINT ( 'NONE',  ( -4.286401442266592809, 4.198423832313131321, 5.000000000000004441 ) ) ;
#6784=CARTESIAN_POINT ( 'NONE',  ( -0.9739805876846552302, -5.920636045238190093, 18.26171386814421638 ) ) ;
#6786=VERTEX_POINT ( 'NONE', #1594 ) ;
#6792=ORIENTED_EDGE ( 'NONE', *, *, #13029, .T. ) ;
#6795=CARTESIAN_POINT ( 'NONE',  ( -2.817313151351206635, 5.579000502529421368, 31.00000000000000000 ) ) ;
#6796=CARTESIAN_POINT ( 'NONE',  ( 2.930922878467330683, 5.520395124723648017, 25.00389213124970311 ) ) ;
#6799=CARTESIAN_POINT ( 'NONE',  ( -7.799024015210642702, -1.482594289697281020, 11.49999999999998224 ) ) ;
#6800=EDGE_CURVE ( 'NONE', #13757, #2306, #14892, .T. ) ;
#6810=CARTESIAN_POINT ( 'NONE',  ( -4.154121946521027731, 4.670585111242834486, 17.20112161576660981 ) ) ;
#6813=CARTESIAN_POINT ( 'NONE',  ( 6.123233995736766282E-16, 6.000000000000000888, 6.000000000000005329 ) ) ;
#6814=EDGE_LOOP ( 'NONE', ( #2491, #7019, #10115, #9800 ) ) ;
#6815=LINE ( 'NONE', #15161, #2838 ) ;
#6816=CARTESIAN_POINT ( 'NONE',  ( 6.123233995736766282E-16, -6.000000000000000888, 6.000000000000005329 ) ) ;
#6817=CARTESIAN_POINT ( 'NONE',  ( 2.840966774240180293, -5.567223638426896493, 17.73809786915986564 ) ) ;
#6827=CARTESIAN_POINT ( 'NONE',  ( 0.8738239080081631194, 6.188820299975577477, 25.00355795710154894 ) ) ;
#6831=ADVANCED_FACE ( 'NONE', ( #15047 ), #3900, .F. ) ;
#6834=ORIENTED_EDGE ( 'NONE', *, *, #12237, .F. ) ;
#6839=DIRECTION ( 'NONE',  ( 0.8090169943749421222, 0.5877852522924802425, 0.000000000000000000 ) ) ;
#6840=FACE_OUTER_BOUND ( 'NONE', #13234, .T. ) ;
#6844=FACE_BOUND ( 'NONE', #10841, .T. ) ;
#6852=CARTESIAN_POINT ( 'NONE',  ( -2.668367453516813814, -5.373994336898041624, 24.49999999999999289 ) ) ;
#6854=CARTESIAN_POINT ( 'NONE',  ( -3.420659742068393072, 4.931142898501730265, 31.99995053646223653 ) ) ;
#6857=CARTESIAN_POINT ( 'NONE',  ( -0.5039005892418949584, 6.230833003620559474, 23.62636388911295171 ) ) ;
#6859=CYLINDRICAL_SURFACE ( 'NONE', #11629, 1.000000000000000888 ) ;
#6862=CARTESIAN_POINT ( 'NONE',  ( -5.935543223013826086, -0.8771126767608832253, 17.99999999999998934 ) ) ;
#6863=CARTESIAN_POINT ( 'NONE',  ( -0.6144377077728601089, -5.969178481556079774, 17.20033966857735663 ) ) ;
#6868=CARTESIAN_POINT ( 'NONE',  ( 3.882809187878895507, -4.899079348630081654, 18.97400098023329562 ) ) ;
#6871=CARTESIAN_POINT ( 'NONE',  ( 5.486982057989242101, -2.429327048029762626, 18.79931806258173665 ) ) ;
#6874=CARTESIAN_POINT ( 'NONE',  ( 0.2619456584322039094, -5.995505046955617701, 4.026071939286484103 ) ) ;
#6876=CARTESIAN_POINT ( 'NONE',  ( -3.882673863916208390, -4.899192824801000157, 4.025914576658296440 ) ) ;
#6882=CARTESIAN_POINT ( 'NONE',  ( -5.935543223013847403, -0.8771126767607489993, 5.000000000000004441 ) ) ;
#6885=ORIENTED_EDGE ( 'NONE', *, *, #12497, .F. ) ;
#6886=CARTESIAN_POINT ( 'NONE',  ( 3.421280866381210650, -4.930711975950862858, 3.999950679266884634 ) ) ;
#6888=CARTESIAN_POINT ( 'NONE',  ( -3.459447313391952328, 5.206669755180917569, 17.02599901976669017 ) ) ;
#6889=EDGE_CURVE ( 'NONE', #478, #4153, #5468, .T. ) ;
#6890=FACE_OUTER_BOUND ( 'NONE', #10516, .T. ) ;
#6891=CARTESIAN_POINT ( 'NONE',  ( 5.558508435838283468, 2.857531096718751051, 24.36762589283694425 ) ) ;
#6892=VERTEX_POINT ( 'NONE', #12801 ) ;
#6894=FACE_BOUND ( 'NONE', #2435, .T. ) ;
#6895=CARTESIAN_POINT ( 'NONE',  ( 2.996417732210528762, -5.485687819086929373, 17.38603820591928439 ) ) ;
#6898=EDGE_CURVE ( 'NONE', #15036, #398, #10950, .T. ) ;
#6905=CARTESIAN_POINT ( 'NONE',  ( 2.031800924094035195E-13, 6.250000000000000888, 23.49999999999999289 ) ) ;
#6909=DIRECTION ( 'NONE',  ( 0.000000000000000000, 0.000000000000000000, 1.000000000000000000 ) ) ;
#6910=ORIENTED_EDGE ( 'NONE', *, *, #14100, .T. ) ;
#6911=CARTESIAN_POINT ( 'NONE',  ( -5.648794263291730289, 2.676232015153646504, 18.61441947245482709 ) ) ;
#6912=ORIENTED_EDGE ( 'NONE', *, *, #9889, .T. ) ;
#6913=EDGE_CURVE ( 'NONE', #10984, #2248, #3255, .T. ) ;
#6914=FACE_OUTER_BOUND ( 'NONE', #8157, .T. ) ;
#6916=CARTESIAN_POINT ( 'NONE',  ( 5.558508435838322548, -2.857531096718671115, 24.49999999999999289 ) ) ;
#6918=CARTESIAN_POINT ( 'NONE',  ( 5.131373506000584506, 7.062729720844102665, 31.00000000000000000 ) ) ;
#6923=VECTOR ( 'NONE', #4421, 1000.000000000000000 ) ;
#6925=ORIENTED_EDGE ( 'NONE', *, *, #14615, .T. ) ;
#6927=CARTESIAN_POINT ( 'NONE',  ( 3.419318284370212790, 4.932111238568167799, 30.00007997643738022 ) ) ;
#6930=ADVANCED_FACE ( 'NONE', ( #6624 ), #9090, .F. ) ;
#6931=CIRCLE ( 'NONE', #2603, 6.250000000000000888 ) ;
#6932=CARTESIAN_POINT ( 'NONE',  ( -3.311384659207154968, 5.004923837169406475, 31.97358595436693918 ) ) ;
#6935=DIRECTION ( 'NONE',  ( -0.3090169943749447867, -0.9510565162951544194, 0.000000000000000000 ) ) ;
#6939=CARTESIAN_POINT ( 'NONE',  ( 2.996417732210555851, 5.485687819086916051, 31.61396179408072626 ) ) ;
#6940=CARTESIAN_POINT ( 'NONE',  ( 5.317509234263941842, 2.779225709351030638, 31.00000000000000000 ) ) ;
#6941=EDGE_LOOP ( 'NONE', ( #14029, #11527, #2634, #13235 ) ) ;
#6944=B_SPLINE_CURVE_WITH_KNOTS ( 'NONE', 3,
 ( #13324, #10862, #6101, #10943, #4907, #8168, #11888, #7053, #11810, #10630, #15492, #11020, #120, #7367, #12209, #13404, #6182, #2514 ),
 .UNSPECIFIED., .F., .F.,
 ( 4, 2, 2, 2, 2, 2, 2, 2, 4 ),
 ( 0.000000000000000000, 0.0003914898357794942426, 0.0007829796715589884852, 0.001174469507338482674, 0.001565959343117976970, 0.001957449178897471918, 0.002348939014676966648, 0.002740428850456461812, 0.003131918686235956543 ),
 .UNSPECIFIED. ) ;
#6945=ORIENTED_EDGE ( 'NONE', *, *, #7757, .T. ) ;
#6947=CARTESIAN_POINT ( 'NONE',  ( -2.782713018890709211, 5.315928322779123860, 12.00439760644213294 ) ) ;
#6950=CARTESIAN_POINT ( 'NONE',  ( 0.9735856429312852445, -5.920699391845026582, 5.262852839067273081 ) ) ;
#6954=CARTESIAN_POINT ( 'NONE',  ( 6.176542424588118863, -0.9554180641285446862, 5.000000000000004441 ) ) ;
#6956=B_SPLINE_CURVE_WITH_KNOTS ( 'NONE', 3,
 ( #13418, #13642, #14852, #3632, #12146, #6434, #12375, #11266, #6354, #8508, #11188, #287, #4996, #5150, #2596, #11109, #1245, #11032 ),
 .UNSPECIFIED., .F., .F.,
 ( 4, 2, 2, 2, 2, 2, 2, 2, 4 ),
 ( 0.003131486019301991160, 0.003522824630466697866, 0.003914163241631404139, 0.004305501852796111278, 0.004696840463960817551, 0.005088179075125523823, 0.005479517686290230963, 0.005870856297454938102, 0.006262194908619644375 ),
 .UNSPECIFIED. ) ;
#6957=CARTESIAN_POINT ( 'NONE',  ( 4.344313232727172291, -4.493553492990049136, 4.495630303198468347 ) ) ;
#6961=CARTESIAN_POINT ( 'NONE',  ( -5.330004929009523273, 2.755647751839523707, 24.76239891805597537 ) ) ;
#6964=CARTESIAN_POINT ( 'NONE',  ( -6.105861027178926648, 1.337741388557089461, 25.29954462468842991 ) ) ;
#6967=EDGE_LOOP ( 'NONE', ( #12179, #3006 ) ) ;
#6969=CARTESIAN_POINT ( 'NONE',  ( -5.940390500375658078, 6.474944468551550258, 5.000000000000004441 ) ) ;
#6972=CARTESIAN_POINT ( 'NONE',  ( -4.290821322214476652, -4.545321419741457980, 25.11441947245483419 ) ) ;
#6976=EDGE_CURVE ( 'NONE', #3914, #11745, #7350, .T. ) ;
#6978=CARTESIAN_POINT ( 'NONE',  ( 2.692143549875383179, 5.362363179736484575, 31.26194324003146718 ) ) ;
#6979=CARTESIAN_POINT ( 'NONE',  ( 0.1323408341374962827, 6.250000000000000888, 25.50000000000002132 ) ) ;
#6984=CARTESIAN_POINT ( 'NONE',  ( 2.930600586412863251, -5.520563544161807279, 25.00308643866044989 ) ) ;
#6985=EDGE_CURVE ( 'NONE', #721, #8233, #8306, .T. ) ;
#6987=ORIENTED_EDGE ( 'NONE', *, *, #14060, .F. ) ;
#6989=CYLINDRICAL_SURFACE ( 'NONE', #15456, 1.000000000000000666 ) ;
#6993=CARTESIAN_POINT ( 'NONE',  ( -3.158825713737527963, 5.393784879207143668, 5.799331489075775004 ) ) ;
#6998=DIRECTION ( 'NONE',  ( -0.5877852522924685852, -0.8090169943749507819, 0.000000000000000000 ) ) ;
#7004=CARTESIAN_POINT ( 'NONE',  ( 4.322356511625595310, 7.650514973136599117, 11.49999999999998224 ) ) ;
#7005=CARTESIAN_POINT ( 'NONE',  ( -5.935543223013836744, -0.8771126767608161678, 11.49999999999998224 ) ) ;
#7007=CARTESIAN_POINT ( 'NONE',  ( 3.311576095066539160, -5.004818610361334130, 18.97377823943292086 ) ) ;
#7010=CARTESIAN_POINT ( 'NONE',  ( -6.250000000000000888, 0.000000000000000000, 0.000000000000000000 ) ) ;
#7012=VECTOR ( 'NONE', #8002, 1000.000000000000114 ) ;
#7013=CARTESIAN_POINT ( 'NONE',  ( 0.6151877315910210253, -6.220340188096013634, 31.79906673469668732 ) ) ;
#7014=CARTESIAN_POINT ( 'NONE',  ( 3.159612573729224216, 5.393342049074633771, 31.80026515017676658 ) ) ;
#7016=ORIENTED_EDGE ( 'NONE', *, *, #4161, .F. ) ;
#7017=EDGE_CURVE ( 'NONE', #11546, #9142, #10392, .T. ) ;
#7018=EDGE_LOOP ( 'NONE', ( #1443, #15390, #11449, #392 ) ) ;
#7019=ORIENTED_EDGE ( 'NONE', *, *, #9903, .F. ) ;
#7021=DIRECTION ( 'NONE',  ( -0.3090169943749446202, -0.9510565162951544194, 0.000000000000000000 ) ) ;
#7022=EDGE_CURVE ( 'NONE', #727, #12035, #8111, .T. ) ;
#7026=CARTESIAN_POINT ( 'NONE',  ( -0.8002302970944432658, 5.947135855825893991, 23.88601773212297630 ) ) ;
#7030=CARTESIAN_POINT ( 'NONE',  ( 6.021135683317697662, -1.680226122398213340, 4.026227171247320769 ) ) ;
#7032=CARTESIAN_POINT ( 'NONE',  ( 3.159612573729294827, -5.393342049074592026, 30.19973484982324408 ) ) ;
#7035=CARTESIAN_POINT ( 'NONE',  ( 3.459597053047735127, 5.206576120509819106, 18.97408542334169823 ) ) ;
#7036=ORIENTED_EDGE ( 'NONE', *, *, #1067, .F. ) ;
#7037=CARTESIAN_POINT ( 'NONE',  ( -5.620879908643923173, 2.102487719022013479, 25.47377823943293862 ) ) ;
#7038=EDGE_LOOP ( 'NONE', ( #14506, #4949, #8692, #13933 ) ) ;
#7040=CARTESIAN_POINT ( 'NONE',  ( -5.615811513734953131, 2.743665920700568250, 25.00308643866045344 ) ) ;
#7042=EDGE_LOOP ( 'NONE', ( #5921, #2126 ) ) ;
#7043=CARTESIAN_POINT ( 'NONE',  ( 3.419318284370244765, -4.932111238568142930, 12.49992002356259668 ) ) ;
#7044=CARTESIAN_POINT ( 'NONE',  ( 5.330189595673701319, -2.755293208590119836, 17.73617396794405821 ) ) ;
#7047=CARTESIAN_POINT ( 'NONE',  ( -6.176542424588072677, -0.9554180641288341214, 24.49999999999999289 ) ) ;
#7053=CARTESIAN_POINT ( 'NONE',  ( 5.620786884546286721, 2.102685372472903769, 10.52641404563305016 ) ) ;
#7055=CARTESIAN_POINT ( 'NONE',  ( 5.665707375537437862, 1.979196487016773975, 32.00007961174475923 ) ) ;
#7056=ORIENTED_EDGE ( 'NONE', *, *, #13222, .T. ) ;
#7057=DIRECTION ( 'NONE',  ( -0.9510565162951544194, 0.3090169943749447312, 0.000000000000000000 ) ) ;
#7058=CARTESIAN_POINT ( 'NONE',  ( 6.768587589771821120E-14, -6.250000000000000888, 11.49999999999998224 ) ) ;
#7059=CARTESIAN_POINT ( 'NONE',  ( -0.8738118504723636493, -5.936246475285062552, 25.00357242174242245 ) ) ;
#7061=DIRECTION ( 'NONE',  ( 0.5877852522924802425, -0.8090169943749422332, 0.000000000000000000 ) ) ;
#7062=FACE_OUTER_BOUND ( 'NONE', #8378, .T. ) ;
#7064=EDGE_CURVE ( 'NONE', #10038, #15573, #14555, .T. ) ;
#7065=VECTOR ( 'NONE', #2937, 1000.000000000000114 ) ;
#7068=CARTESIAN_POINT ( 'NONE',  ( 5.558508435838283468, 2.857531096718750607, 24.49999999999999289 ) ) ;
#7069=FACE_OUTER_BOUND ( 'NONE', #8373, .T. ) ;
#7072=CARTESIAN_POINT ( 'NONE',  ( 6.176542424588115310, 0.9554180641285648923, 11.49999999999998224 ) ) ;
#7074=CARTESIAN_POINT ( 'NONE',  ( -4.267992336621142080, -4.217442018460050512, 30.73805675996852216 ) ) ;
#7077=AXIS2_PLACEMENT_3D ( 'NONE', #15174, #10402, #12702 ) ;
#7084=CARTESIAN_POINT ( 'NONE',  ( 5.375886393124394758, 2.665038680141264216, 17.49560239355787417 ) ) ;
#7086=VECTOR ( 'NONE', #10519, 1000.000000000000000 ) ;
#7087=CARTESIAN_POINT ( 'NONE',  ( 2.668367453516506504, 5.373994336898192614, 17.99999999999998934 ) ) ;
#7091=CARTESIAN_POINT ( 'NONE',  ( -5.935543223013850955, 0.8771126767607324570, 11.49999999999998224 ) ) ;
#7092=CARTESIAN_POINT ( 'NONE',  ( 5.746619684944255901, 1.730157667110902242, 3.999950679266886855 ) ) ;
#7093=DIRECTION ( 'NONE',  ( 0.8090169943749506709, -0.5877852522924686962, 0.000000000000000000 ) ) ;
#7094=VERTEX_POINT ( 'NONE', #5252 ) ;
#7097=ORIENTED_EDGE ( 'NONE', *, *, #6211, .T. ) ;
#7099=CARTESIAN_POINT ( 'NONE',  ( -3.011139120916598078, 5.190534000030295303, 12.29931806258173843 ) ) ;
#7102=CARTESIAN_POINT ( 'NONE',  ( 7.347880347650999152E-16, -6.000000000000000888, 4.000000000000004441 ) ) ;
#7103=B_SPLINE_CURVE_WITH_KNOTS ( 'NONE', 3,
 ( #2346, #12133, #14351, #8248, #14270, #2107, #2182, #13084, #5860, #4666, #4745, #9764, #913, #3380, #8497, #10785, #4588, #3305 ),
 .UNSPECIFIED., .F., .F.,
 ( 4, 2, 2, 2, 2, 2, 2, 2, 4 ),
 ( 0.000000000000000000, 0.0003914357524127490035, 0.0007828715048254980069, 0.001174307257238247065, 0.001565743009650996014, 0.001957178762063744963, 0.002348614514476494129, 0.002740050266889242862, 0.003131486019301992028 ),
 .UNSPECIFIED. ) ;
#7106=EDGE_CURVE ( 'NONE', #398, #15036, #5631, .T. ) ;
#7109=CARTESIAN_POINT ( 'NONE',  ( 5.770288754215126659, -2.404361317819967869, 4.126180359549290522 ) ) ;
#7112=CARTESIAN_POINT ( 'NONE',  ( 2.817313151351170220, -5.579000502529441796, 30.86936067245787285 ) ) ;
#7114=CARTESIAN_POINT ( 'NONE',  ( 4.322356511625540243, 7.650514973136639973, 17.99999999999998934 ) ) ;
#7118=ORIENTED_EDGE ( 'NONE', *, *, #14093, .T. ) ;
#7120=CARTESIAN_POINT ( 'NONE',  ( -5.558508435838179551, -2.857531096718951336, 31.00000000000000000 ) ) ;
#7121=CARTESIAN_POINT ( 'NONE',  ( -2.817313151351291012, -5.579000502529380512, 24.49999999999999289 ) ) ;
#7124=LINE ( 'NONE', #8403, #11479 ) ;
#7127=CARTESIAN_POINT ( 'NONE',  ( -2.849573632035240944, -5.280958870664618665, 12.11561732698604743 ) ) ;
#7130=CARTESIAN_POINT ( 'NONE',  ( -2.817313151351291012, -5.579000502529380512, 24.49999999999999289 ) ) ;
#7132=EDGE_CURVE ( 'NONE', #8233, #721, #2607, .T. ) ;
#7135=CARTESIAN_POINT ( 'NONE',  ( 2.668367453516610421, 5.373994336898141100, 31.13064961348856130 ) ) ;
#7136=B_SPLINE_CURVE_WITH_KNOTS ( 'NONE', 3,
 ( #12120, #12198, #5850, #8487, #1221, #3447, #11961, #3764, #4736, #12044, #14675, #8564, #13239, #6090, #8642, #2332, #1065, #10775 ),
 .UNSPECIFIED., .F., .F.,
 ( 4, 2, 2, 2, 2, 2, 2, 2, 4 ),
 ( 0.000000000000000000, 0.0003914357524127472687, 0.0007828715048254945375, 0.001174307257238241860, 0.001565743009650989075, 0.001957178762063736290, 0.002348614514476483721, 0.002740050266889230719, 0.003131486019301978150 ),
 .UNSPECIFIED. ) ;
#7139=CARTESIAN_POINT ( 'NONE',  ( -3.011385983131360522, 5.190390249166416226, 4.200479458972859348 ) ) ;
#7140=CARTESIAN_POINT ( 'NONE',  ( 4.286401442266437378, 4.198423832313292081, 17.99999999999998934 ) ) ;
#7142=VERTEX_POINT ( 'NONE', #7297 ) ;
#7143=CARTESIAN_POINT ( 'NONE',  ( 3.882809187879000756, -4.899079348629999053, 31.97400098023329917 ) ) ;
#7146=CARTESIAN_POINT ( 'NONE',  ( -4.267838854167091078, -4.217593933790421801, 5.262398918055981589 ) ) ;
#7161=CARTESIAN_POINT ( 'NONE',  ( -3.883588957979214218, -4.898466244118963253, 12.47377282875266324 ) ) ;
#7162=ORIENTED_EDGE ( 'NONE', *, *, #6612, .T. ) ;
#7163=LINE ( 'NONE', #11124, #3544 ) ;
#7164=CARTESIAN_POINT ( 'NONE',  ( 0.7993401192313895898, -6.199366368793636006, 25.11483246936573011 ) ) ;
#7168=CARTESIAN_POINT ( 'NONE',  ( 3.421280866381198216, -4.930711975950873516, 29.99995067926688108 ) ) ;
#7171=CARTESIAN_POINT ( 'NONE',  ( 5.903347812666358330, -1.076697810262539745, 31.61397738943081492 ) ) ;
#7172=CARTESIAN_POINT ( 'NONE',  ( 0.1323736289504560126, -6.250000000000000888, 32.00000000000000000 ) ) ;
#7173=CARTESIAN_POINT ( 'NONE',  ( 5.317509234263995133, 2.779225709350928053, 17.99999999999998934 ) ) ;
#7175=ADVANCED_FACE ( 'NONE', ( #4989 ), #10712, .F. ) ;
#7176=VERTEX_POINT ( 'NONE', #11975 ) ;
#7177=EDGE_CURVE ( 'NONE', #9802, #7295, #13957, .T. ) ;
#7180=CARTESIAN_POINT ( 'NONE',  ( -4.286401442266640771, 4.198423832313082471, 11.49999999999998224 ) ) ;
#7185=CARTESIAN_POINT ( 'NONE',  ( -5.770167736194668606, -2.404664418229233824, 12.37367328635990482 ) ) ;
#7189=CARTESIAN_POINT ( 'NONE',  ( 2.030576276931546336E-13, -6.250000000000000888, 24.49999999999999289 ) ) ;
#7194=CARTESIAN_POINT ( 'NONE',  ( 5.770288754215089355, 2.404361317820048694, 5.873819640450716584 ) ) ;
#7195=EDGE_LOOP ( 'NONE', ( #2632, #14565, #14968, #10438 ) ) ;
#7200=CARTESIAN_POINT ( 'NONE',  ( 0.7988860301922496854, 6.199427171881334075, 30.38455580536195555 ) ) ;
#7201=CARTESIAN_POINT ( 'NONE',  ( -3.458467055437357995, -5.207305717053783312, 23.52640428276697904 ) ) ;
#7202=CARTESIAN_POINT ( 'NONE',  ( -3.923477796648640936, -4.541042560386369331, 25.37303779027050510 ) ) ;
#7204=CARTESIAN_POINT ( 'NONE',  ( 4.141923667210667404, -4.342011609040446807, 12.11561732698604388 ) ) ;
#7205=CARTESIAN_POINT ( 'NONE',  ( 5.843318061569083177, -1.367618216965475808, 17.12696220972948069 ) ) ;
#7208=CARTESIAN_POINT ( 'NONE',  ( 5.317509234263941842, 2.779225709351030638, 30.86760611998364823 ) ) ;
#7209=FACE_OUTER_BOUND ( 'NONE', #5086, .T. ) ;
#7213=B_SPLINE_CURVE_WITH_KNOTS ( 'NONE', 3,
 ( #8190, #4446, #9300, #3244, #8112, #10568, #12074, #15585, #12304, #4687, #1251, #8431, #137, #1172, #3794, #14705, #9855, #6127 ),
 .UNSPECIFIED., .F., .F.,
 ( 4, 2, 2, 2, 2, 2, 2, 2, 4 ),
 ( 0.003131923598876997471, 0.003523316383094313945, 0.003914709167311630419, 0.004306101951528947328, 0.004697494735746264236, 0.005088887519963581144, 0.005480280304180898052, 0.005871673088398214092, 0.006263065872615531000 ),
 .UNSPECIFIED. ) ;
#7215=CARTESIAN_POINT ( 'NONE',  ( 4.286401442266517314, 4.198423832313209481, 31.13239388001635888 ) ) ;
#7219=EDGE_LOOP ( 'NONE', ( #15375, #10689, #4808, #11160 ) ) ;
#7221=DIRECTION ( 'NONE',  ( 0.000000000000000000, 1.000000000000000000, 0.000000000000000000 ) ) ;
#7225=CARTESIAN_POINT ( 'NONE',  ( -2.668367453516831134, 5.373994336898032742, 17.99999999999998934 ) ) ;
#7226=CARTESIAN_POINT ( 'NONE',  ( 4.290130679986412510, 4.545972905167880995, 23.88439807107078394 ) ) ;
#7236=ORIENTED_EDGE ( 'NONE', *, *, #10283, .F. ) ;
#7241=FACE_OUTER_BOUND ( 'NONE', #15626, .T. ) ;
#7243=DIRECTION ( 'NONE',  ( 1.000000000000000000, 0.000000000000000000, 0.000000000000000000 ) ) ;
#7247=CARTESIAN_POINT ( 'NONE',  ( 4.195842658231526023, -4.289229542213112367, 30.49560239355786351 ) ) ;
#7252=CARTESIAN_POINT ( 'NONE',  ( 5.531796221294842830, 2.326749136277297403, 4.126215691297386634 ) ) ;
#7254=VECTOR ( 'NONE', #3286, 1000.000000000000114 ) ;
#7256=B_SPLINE_CURVE_WITH_KNOTS ( 'NONE', 3,
 ( #549, #2866, #13599, #5419, #8845, #10265, #10033, #11218, #14883, #7640, #12564, #7560, #12485, #15117, #4215, #1585, #6464, #12409 ),
 .UNSPECIFIED., .F., .F.,
 ( 4, 2, 2, 2, 2, 2, 2, 2, 4 ),
 ( 0.003131918686235978661, 0.003523310662250268930, 0.003914702638264559199, 0.004306094614278849035, 0.004697486590293139738, 0.005088878566307429574, 0.005480270542321719410, 0.005871662518336009245, 0.006263054494350299949 ),
 .UNSPECIFIED. ) ;
#7257=ORIENTED_EDGE ( 'NONE', *, *, #178, .F. ) ;
#7263=CARTESIAN_POINT ( 'NONE',  ( 5.317509234264001350, -2.779225709350912954, 11.49999999999998224 ) ) ;
#7267=B_SPLINE_CURVE_WITH_KNOTS ( 'NONE', 3,
 ( #12197, #9670, #13238, #4895, #4974, #13152, #6089, #4653, #5928, #14259, #1295, #2330, #4814, #4735, #8236, #8485, #10693, #107 ),
 .UNSPECIFIED., .F., .F.,
 ( 4, 2, 2, 2, 2, 2, 2, 2, 4 ),
 ( 0.000000000000000000, 0.0003914362731607610437, 0.0007828725463215218706, 0.001174308819482282806, 0.001565745092643043741, 0.001957181365803804460, 0.002348617638964565612, 0.002740053912125326764, 0.003131490185286087483 ),
 .UNSPECIFIED. ) ;
#7268=CARTESIAN_POINT ( 'NONE',  ( 7.180990026460762010, -3.384707322287334286, 11.49999999999998224 ) ) ;
#7271=CARTESIAN_POINT ( 'NONE',  ( 4.290381260516336503, -4.545736887716150143, 30.38482219624157565 ) ) ;
#7275=ORIENTED_EDGE ( 'NONE', *, *, #445, .T. ) ;
#7278=ORIENTED_EDGE ( 'NONE', *, *, #7284, .T. ) ;
#7279=CARTESIAN_POINT ( 'NONE',  ( -6.020865209844567190, 1.681180471732243831, 25.47400098023329562 ) ) ;
#7280=ADVANCED_FACE ( 'NONE', ( #46 ), #9522, .F. ) ;
#7281=FACE_OUTER_BOUND ( 'NONE', #6322, .T. ) ;
#7282=CARTESIAN_POINT ( 'NONE',  ( 2.817313151350924638, 5.579000502529565253, 24.49999999999999289 ) ) ;
#7283=CARTESIAN_POINT ( 'NONE',  ( 4.195795028115062664, -4.289273350251292527, 12.00428920362018737 ) ) ;
#7284=EDGE_CURVE ( 'NONE', #7295, #9802, #4871, .T. ) ;
#7286=CARTESIAN_POINT ( 'NONE',  ( -3.312341048453435910, -5.004306261885476559, 12.47398020122238371 ) ) ;
#7287=CARTESIAN_POINT ( 'NONE',  ( -2.817313151351230616, -5.579000502529413374, 18.13234125634167171 ) ) ;
#7289=CARTESIAN_POINT ( 'NONE',  ( 0.5044069930204643226, -5.979990686694983459, 18.87335743227902896 ) ) ;
#7294=CARTESIAN_POINT ( 'NONE',  ( 3.312524433819795000, 5.004191858253993708, 31.97408052783100274 ) ) ;
#7295=VERTEX_POINT ( 'NONE', #10947 ) ;
#7297=CARTESIAN_POINT ( 'NONE',  ( 2.668367453516645504, -5.373994336898123336, 11.49999999999998224 ) ) ;
#7298=CARTESIAN_POINT ( 'NONE',  ( 5.935543223013876712, 0.8771126767605440522, 24.49999999999999289 ) ) ;
#7301=CARTESIAN_POINT ( 'NONE',  ( 7.490007020835748541, -2.433650805992050969, 24.49999999999999289 ) ) ;
#7302=CARTESIAN_POINT ( 'NONE',  ( 4.069800786343640731, 4.744882212776960984, 23.62618035954928786 ) ) ;
#7304=CARTESIAN_POINT ( 'NONE',  ( 5.931793676715094499, -0.9035324301688607562, 4.737601081944046832 ) ) ;
#7306=EDGE_CURVE ( 'NONE', #7463, #3603, #6931, .T. ) ;
#7307=CARTESIAN_POINT ( 'NONE',  ( -5.615811513735013527, 2.743665920700446126, 12.00308643866043745 ) ) ;
#7312=CARTESIAN_POINT ( 'NONE',  ( 6.176542424588125968, 0.9554180641284963915, 17.99999999999998934 ) ) ;
#7314=VERTEX_POINT ( 'NONE', #1358 ) ;
#7317=CARTESIAN_POINT ( 'NONE',  ( 6.768587589771821120E-14, -6.250000000000000888, 11.49999999999998224 ) ) ;
#7319=VERTEX_POINT ( 'NONE', #7263 ) ;
#7320=DIRECTION ( 'NONE',  ( 0.000000000000000000, 1.000000000000000000, 0.000000000000000000 ) ) ;
#7322=PLANE ( 'NONE',  #12886 ) ;
#7325=CARTESIAN_POINT ( 'NONE',  ( 3.107278289587259934, -5.134157760522006342, 30.12635295315577011 ) ) ;
#7327=CARTESIAN_POINT ( 'NONE',  ( -0.2624013748572930349, -5.995472630654521851, 30.02628559691082444 ) ) ;
#7330=CARTESIAN_POINT ( 'NONE',  ( 5.935543223013846514, 0.8771126767607477781, 5.000000000000004441 ) ) ;
#7332=VERTEX_POINT ( 'NONE', #1124 ) ;
#7334=ORIENTED_EDGE ( 'NONE', *, *, #13611, .F. ) ;
#7335=CARTESIAN_POINT ( 'NONE',  ( -3.735642931251201393, 4.696778275484337684, 25.47408052783099919 ) ) ;
#7336=ORIENTED_EDGE ( 'NONE', *, *, #11585, .T. ) ;
#7339=CARTESIAN_POINT ( 'NONE',  ( -5.615973259022280395, -2.743340227996256875, 12.00389213124966759 ) ) ;
#7340=CARTESIAN_POINT ( 'NONE',  ( 6.123233995736766282E-16, 6.000000000000000888, 6.000000000000005329 ) ) ;
#7344=CARTESIAN_POINT ( 'NONE',  ( -6.142908455506903564, -1.155755562476258325, 25.11517780375841014 ) ) ;
#7346=CYLINDRICAL_SURFACE ( 'NONE', #5059, 1.000000000000000888 ) ;
#7348=CARTESIAN_POINT ( 'NONE',  ( 6.143020266950966146, 1.155160780047777891, 5.614419472454844851 ) ) ;
#7350=B_SPLINE_CURVE_WITH_KNOTS ( 'NONE', 3,
 ( #9312, #15124, #4221, #15439, #14152, #10430, #11456, #2059, #5504, #11766, #1827, #14073, #5583, #15281, #4383, #7883, #6701, #4539 ),
 .UNSPECIFIED., .F., .F.,
 ( 4, 2, 2, 2, 2, 2, 2, 2, 4 ),
 ( 0.003131486019301987691, 0.003522824630466694831, 0.003914163241631402404, 0.004305501852796109544, 0.004696840463960814949, 0.005088179075125522088, 0.005479517686290227493, 0.005870856297454933766, 0.006262194908619640038 ),
 .UNSPECIFIED. ) ;
#7351=VERTEX_POINT ( 'NONE', #7340 ) ;
#7352=ORIENTED_EDGE ( 'NONE', *, *, #15177, .F. ) ;
#7353=ORIENTED_EDGE ( 'NONE', *, *, #13572, .T. ) ;
#7354=EDGE_CURVE ( 'NONE', #12191, #1121, #12440, .T. ) ;
#7357=CARTESIAN_POINT ( 'NONE',  ( 3.922396193919052365, -4.541970110199439858, 12.37380682714708691 ) ) ;
#7358=LINE ( 'NONE', #8715, #13647 ) ;
#7360=CARTESIAN_POINT ( 'NONE',  ( -2.692693252389579239, -5.362085866495110764, 11.76382603205595778 ) ) ;
#7361=CARTESIAN_POINT ( 'NONE',  ( -6.105861027178971945, 1.337741388556887401, 5.799544624688434347 ) ) ;
#7362=CARTESIAN_POINT ( 'NONE',  ( 1.000049560716691266, -5.916071405810123807, 17.86967799011533131 ) ) ;
#7363=CARTESIAN_POINT ( 'NONE',  ( 6.250000000000000888, 7.654042494670958593E-16, 53.67766952966368876 ) ) ;
#7367=CARTESIAN_POINT ( 'NONE',  ( 5.903347812666351224, 1.076697810262578381, 10.88602261056916198 ) ) ;
#7370=EDGE_LOOP ( 'NONE', ( #8307, #2708 ) ) ;
#7372=CARTESIAN_POINT ( 'NONE',  ( -4.196288036172428626, 4.288789315524856427, 4.496879510976232730 ) ) ;
#7373=CARTESIAN_POINT ( 'NONE',  ( -0.1306171417087921838, -6.000000000000000888, 10.49999999999998401 ) ) ;
#7375=CARTESIAN_POINT ( 'NONE',  ( 2.841163418881454739, -5.567120626447898069, 31.26236973443874945 ) ) ;
#7376=CARTESIAN_POINT ( 'NONE',  ( -2.817313151351189315, 5.579000502529432026, 5.000000000000004441 ) ) ;
#7377=CARTESIAN_POINT ( 'NONE',  ( 2.817313151350924638, 5.579000502529565253, 24.49999999999999289 ) ) ;
#7379=DIRECTION ( 'NONE',  ( 0.000000000000000000, 1.000000000000000000, 0.000000000000000000 ) ) ;
#7383=FACE_BOUND ( 'NONE', #3341, .T. ) ;
#7386=CARTESIAN_POINT ( 'NONE',  ( 2.094888803305876858E-14, -6.250000000000000888, 30.00000000000000000 ) ) ;
#7387=VERTEX_POINT ( 'NONE', #2395 ) ;
#7390=DIRECTION ( 'NONE',  ( -0.3090169943749584980, 0.9510565162951498674, 0.000000000000000000 ) ) ;
#7393=CARTESIAN_POINT ( 'NONE',  ( -4.143041610105433037, -4.340967609746910760, 23.88602261056917442 ) ) ;
#7394=CARTESIAN_POINT ( 'NONE',  ( 5.329945432499612501, -2.755769831645169088, 5.262290378359324450 ) ) ;
#7395=CARTESIAN_POINT ( 'NONE',  ( 5.558508435838239059, -2.857531096718835428, 31.13237410716304510 ) ) ;
#7396=CARTESIAN_POINT ( 'NONE',  ( 0.9737725088283040176, 6.173885267451808545, 11.23735758726568434 ) ) ;
#7397=ADVANCED_FACE ( 'NONE', ( #12100 ), #5031, .F. ) ;
#7402=CARTESIAN_POINT ( 'NONE',  ( 5.783198643800792738, -1.602922020054615038, 10.52622176056705428 ) ) ;
#7406=AXIS2_PLACEMENT_3D ( 'NONE', #11899, #14128, #770 ) ;
#7407=CARTESIAN_POINT ( 'NONE',  ( -5.940390500375711369, 6.474944468551510290, 11.49999999999998224 ) ) ;
#7414=EDGE_LOOP ( 'NONE', ( #389, #10133 ) ) ;
#7421=CARTESIAN_POINT ( 'NONE',  ( 2.668367453516690357, -5.373994336898101132, 31.00000000000000000 ) ) ;
#7423=CARTESIAN_POINT ( 'NONE',  ( 5.859155363331407962, -2.178872204144911340, 10.52599901976669017 ) ) ;
#7425=ORIENTED_EDGE ( 'NONE', *, *, #13965, .T. ) ;
#7428=CARTESIAN_POINT ( 'NONE',  ( -5.769755079862274094, -2.405651898699083802, 10.62694108445697161 ) ) ;
#7429=CARTESIAN_POINT ( 'NONE',  ( 3.158296126777834889, 5.394094919772085994, 4.201121615766614248 ) ) ;
#7430=CARTESIAN_POINT ( 'NONE',  ( 0.5030929395820232797, 6.230885867001147105, 4.126003191165495743 ) ) ;
#7432=CARTESIAN_POINT ( 'NONE',  ( -4.196288036172456160, -4.288789315524827117, 18.50312048902377526 ) ) ;
#7433=CARTESIAN_POINT ( 'NONE',  ( 3.883716939928997913, -4.898343590941240500, 23.52640428276697904 ) ) ;
#7436=CARTESIAN_POINT ( 'NONE',  ( 0.000000000000000000, 0.000000000000000000, 36.00000000000000711 ) ) ;
#7446=CARTESIAN_POINT ( 'NONE',  ( 4.435347140101025154, -4.403429997944519059, 11.49999999999998224 ) ) ;
#7448=CARTESIAN_POINT ( 'NONE',  ( 0.9739805876849939592, 5.920636045238133249, 24.76171386814422348 ) ) ;
#7450=DIRECTION ( 'NONE',  ( -0.5877852522924685852, -0.8090169943749507819, 0.000000000000000000 ) ) ;
#7454=CARTESIAN_POINT ( 'NONE',  ( -0.9999171162589461925, -6.169494774098552625, 30.86722320330670044 ) ) ;
#7457=EDGE_CURVE ( 'NONE', #9142, #642, #1047, .T. ) ;
#7460=FACE_BOUND ( 'NONE', #12889, .T. ) ;
#7461=CARTESIAN_POINT ( 'NONE',  ( 6.081590040723090063, 1.446205118472959406, 17.12632671364005077 ) ) ;
#7463=VERTEX_POINT ( 'NONE', #8854 ) ;
#7466=CARTESIAN_POINT ( 'NONE',  ( -5.317509234263865459, -2.779225709351170526, 17.99999999999998934 ) ) ;
#7468=ORIENTED_EDGE ( 'NONE', *, *, #5363, .T. ) ;
#7471=CARTESIAN_POINT ( 'NONE',  ( 6.155912734541144182, -1.081577393120831676, 12.00389213124966936 ) ) ;
#7472=CARTESIAN_POINT ( 'NONE',  ( 5.984377695197238722, -1.807429553002233513, 32.00004906876532118 ) ) ;
#7476=CARTESIAN_POINT ( 'NONE',  ( 5.317509234264064411, -2.779225709350791718, 24.63239388001634111 ) ) ;
#7480=CARTESIAN_POINT ( 'NONE',  ( -5.842945980534664407, 1.369128644668877515, 10.62621569129736976 ) ) ;
#7481=CARTESIAN_POINT ( 'NONE',  ( -5.621278735166202800, -2.101423246382545962, 12.47408052783098853 ) ) ;
#7482=CARTESIAN_POINT ( 'NONE',  ( 4.005785023174299297, 4.467917056767537254, 23.70047945897283270 ) ) ;
#7483=EDGE_LOOP ( 'NONE', ( #11725, #15611 ) ) ;
#7487=CARTESIAN_POINT ( 'NONE',  ( -5.746837578675942915, -1.729433780394465936, 25.49995053646222232 ) ) ;
#7492=CARTESIAN_POINT ( 'NONE',  ( 0.000000000000000000, 6.250000000000000888, 25.49999999999999645 ) ) ;
#7494=VECTOR ( 'NONE', #1055, 1000.000000000000114 ) ;
#7497=CARTESIAN_POINT ( 'NONE',  ( 3.107278289587211972, 5.134157760522037428, 5.873647046844244102 ) ) ;
#7500=CARTESIAN_POINT ( 'NONE',  ( -6.081464507797644359, 1.446657058464150714, 30.12619944752604084 ) ) ;
#7503=ORIENTED_EDGE ( 'NONE', *, *, #2535, .F. ) ;
#7506=CARTESIAN_POINT ( 'NONE',  ( 5.375913338529108465, -2.664979843780403090, 30.49571079637980020 ) ) ;
#7507=CARTESIAN_POINT ( 'NONE',  ( 4.290130679986563500, 4.545972905167733558, 4.384398071070797265 ) ) ;
#7509=CARTESIAN_POINT ( 'NONE',  ( -6.105861027178926648, -1.337741388557088129, 17.20045537531157720 ) ) ;
#7510=CARTESIAN_POINT ( 'NONE',  ( 6.000000000000000888, 7.347880794884120722E-16, 0.000000000000000000 ) ) ;
#7511=CARTESIAN_POINT ( 'NONE',  ( 0.5031281619708453112, 5.980084330432663187, 10.62602272744524079 ) ) ;
#7513=CARTESIAN_POINT ( 'NONE',  ( -6.176542424588119751, 0.9554180641285462405, 5.132341256341692137 ) ) ;
#7514=CARTESIAN_POINT ( 'NONE',  ( -2.931156713028594929, 5.520271803279157119, 18.50436969680152899 ) ) ;
#7522=CARTESIAN_POINT ( 'NONE',  ( -5.317509234263920526, -2.779225709351067053, 31.00000000000000000 ) ) ;
#7523=CARTESIAN_POINT ( 'NONE',  ( -5.615973259022258190, 2.743340227996296843, 23.99610786875029689 ) ) ;
#7524=CARTESIAN_POINT ( 'NONE',  ( 0.000000000000000000, 6.250000000000000888, 6.000000000000005329 ) ) ;
#7525=CARTESIAN_POINT ( 'NONE',  ( 5.984377695197213853, 1.807429553002318556, 29.99995093123466816 ) ) ;
#7527=CARTESIAN_POINT ( 'NONE',  ( 4.435347140101010055, 4.403429997944536822, 5.000000000000004441 ) ) ;
#7529=CARTESIAN_POINT ( 'NONE',  ( 5.531757352715596987, -2.326874507723346586, 4.126193172852896218 ) ) ;
#7536=CARTESIAN_POINT ( 'NONE',  ( 3.254737477227931830, 5.337033878705248036, 12.37367328635990482 ) ) ;
#7540=CARTESIAN_POINT ( 'NONE',  ( 5.570760634536868317, -2.834026536768118554, 18.26225281721714566 ) ) ;
#7542=ORIENTED_EDGE ( 'NONE', *, *, #1535, .T. ) ;
#7544=CARTESIAN_POINT ( 'NONE',  ( -2.782713018890674572, -5.315928322779141624, 17.49560239355786706 ) ) ;
#7545=CARTESIAN_POINT ( 'NONE',  ( 5.649053410273110032, -2.675685104943178239, 12.11517780375842790 ) ) ;
#7546=CARTESIAN_POINT ( 'NONE',  ( -4.435347140101107755, -4.403429997944438234, 18.13060690723497004 ) ) ;
#7547=CARTESIAN_POINT ( 'NONE',  ( -5.487348639458908828, 2.428538342494374280, 4.199777826161211536 ) ) ;
#7548=CARTESIAN_POINT ( 'NONE',  ( -0.8738239080079619470, -6.188820299975602346, 12.00355795710141393 ) ) ;
#7549=CARTESIAN_POINT ( 'NONE',  ( 5.409274167810742995, -2.597759609440460693, 25.11519382448850379 ) ) ;
#7552=CARTESIAN_POINT ( 'NONE',  ( 2.848727059636119385, -5.281416301279810099, 5.614425215719389683 ) ) ;
#7553=CARTESIAN_POINT ( 'NONE',  ( -4.154121946520940689, 4.670585111242914422, 30.20112161576660981 ) ) ;
#7554=CARTESIAN_POINT ( 'NONE',  ( -5.375763363753415014, -2.665284979407607668, 12.00389795015984973 ) ) ;
#7555=CARTESIAN_POINT ( 'NONE',  ( -5.782947755040645177, -1.603807858344059145, 10.52601979877758964 ) ) ;
#7559=EDGE_LOOP ( 'NONE', ( #3096, #11144, #14253, #3438 ) ) ;
#7560=CARTESIAN_POINT ( 'NONE',  ( -5.842988226680518871, -1.369004370660901193, 23.62619317285289000 ) ) ;
#7561=EDGE_CURVE ( 'NONE', #7562, #5302, #2118, .T. ) ;
#7562=VERTEX_POINT ( 'NONE', #6270 ) ;
#7563=CARTESIAN_POINT ( 'NONE',  ( -5.931817299736819038, -0.9033986943604223052, 24.76229037835931734 ) ) ;
#7565=B_SPLINE_CURVE_WITH_KNOTS ( 'NONE', 3,
 ( #7524, #12370, #10155, #13725, #11261, #361, #5227, #15009, #10074, #14924, #4099, #7680, #15083, #12605, #6579, #11414, #515, #5385 ),
 .UNSPECIFIED., .F., .F.,
 ( 4, 2, 2, 2, 2, 2, 2, 2, 4 ),
 ( 0.000000000000000000, 0.0003914362731607609353, 0.0007828725463215216538, 0.001174308819482282372, 0.001565745092643043091, 0.001957181365803803592, 0.002348617638964564745, 0.002740053912125325897, 0.003131490185286086615 ),
 .UNSPECIFIED. ) ;
#7566=ORIENTED_EDGE ( 'NONE', *, *, #869, .T. ) ;
#7568=CARTESIAN_POINT ( 'NONE',  ( 0.6156307853269531449, 5.969051238897255196, 5.798705734106810006 ) ) ;
#7570=DIRECTION ( 'NONE',  ( 0.9510565162951500895, 0.3090169943749582204, 0.000000000000000000 ) ) ;
#7573=CARTESIAN_POINT ( 'NONE',  ( -3.011139120916495049, -5.190534000030354811, 10.70068193741825624 ) ) ;
#7574=CARTESIAN_POINT ( 'NONE',  ( 2.668367453516584220, -5.373994336898154422, 17.99999999999998934 ) ) ;
#7576=CARTESIAN_POINT ( 'NONE',  ( 5.726049995854485708, -2.506679546901836364, 10.70045537531157365 ) ) ;
#7578=VERTEX_POINT ( 'NONE', #1476 ) ;
#7579=ORIENTED_EDGE ( 'NONE', *, *, #3072, .T. ) ;
#7581=CARTESIAN_POINT ( 'NONE',  ( 0.8730424326982343386, 5.936362132114442858, 17.49500690218563292 ) ) ;
#7583=VECTOR ( 'NONE', #4641, 1000.000000000000114 ) ;
#7585=CARTESIAN_POINT ( 'NONE',  ( -0.5042987395407722007, -5.979983180450076041, 5.873293041799771963 ) ) ;
#7586=EDGE_CURVE ( 'NONE', #1426, #12192, #295, .T. ) ;
#7587=CARTESIAN_POINT ( 'NONE',  ( 0.9735856429313065608, -5.920699391845023030, 31.26285283906726775 ) ) ;
#7588=CARTESIAN_POINT ( 'NONE',  ( 0.9739805876848602884, 5.920636045238155454, 11.76171386814421105 ) ) ;
#7591=CARTESIAN_POINT ( 'NONE',  ( -5.935543223013826086, -0.8771126767608832253, 17.99999999999998934 ) ) ;
#7594=EDGE_CURVE ( 'NONE', #8395, #15526, #6956, .T. ) ;
#7603=CARTESIAN_POINT ( 'NONE',  ( 6.780834054130108014E-14, -6.250000000000000888, 10.49999999999998224 ) ) ;
#7604=CARTESIAN_POINT ( 'NONE',  ( 6.105747081304161661, 1.338335777572316587, 30.19973484982324408 ) ) ;
#7605=CARTESIAN_POINT ( 'NONE',  ( 5.131373506000546314, 7.062729720844130199, 11.49999999999998224 ) ) ;
#7606=ADVANCED_FACE ( 'NONE', ( #13339 ), #9847, .F. ) ;
#7607=FACE_BOUND ( 'NONE', #2612, .T. ) ;
#7609=CARTESIAN_POINT ( 'NONE',  ( 5.915755444410804031, -1.003187219519845463, 4.496879510976233618 ) ) ;
#7611=CARTESIAN_POINT ( 'NONE',  ( -4.152999119457946087, -4.671604476854382959, 30.19973484982325118 ) ) ;
#7612=B_SPLINE_CURVE_WITH_KNOTS ( 'NONE', 3,
 ( #12136, #2431, #3701, #5863, #1237, #4669, #8578, #13672, #13409, #14355, #8330, #13168, #14921, #3855, #12449, #4988, #10152, #1466 ),
 .UNSPECIFIED., .F., .F.,
 ( 4, 2, 2, 2, 2, 2, 2, 2, 4 ),
 ( 0.003131918686235957410, 0.003523310662250250282, 0.003914702638264542719, 0.004306094614278836025, 0.004697486590293128463, 0.005088878566307420900, 0.005480270542321714206, 0.005871662518336005776, 0.006263054494350299081 ),
 .UNSPECIFIED. ) ;
#7619=CARTESIAN_POINT ( 'NONE',  ( 6.176542424588149949, -0.9554180641283412934, 24.49999999999999289 ) ) ;
#7622=CARTESIAN_POINT ( 'NONE',  ( -5.408775798201109986, -2.598833957129771388, 18.61397738943081848 ) ) ;
#7625=CARTESIAN_POINT ( 'NONE',  ( -3.458467055437294935, -5.207305717053827721, 17.02640428276697904 ) ) ;
#7630=CARTESIAN_POINT ( 'NONE',  ( 2.782156709077283629, 5.316215864844116012, 17.49687951097622829 ) ) ;
#7634=CARTESIAN_POINT ( 'NONE',  ( 5.903472034603569618, -2.056448723544995083, 23.49991780678443121 ) ) ;
#7639=EDGE_LOOP ( 'NONE', ( #7353, #2867 ) ) ;
#7640=CARTESIAN_POINT ( 'NONE',  ( -5.746996058422711329, -1.729015645942137080, 23.49992038825522300 ) ) ;
#7641=ORIENTED_EDGE ( 'NONE', *, *, #6051, .T. ) ;
#7643=VERTEX_POINT ( 'NONE', #3785 ) ;
#7645=CARTESIAN_POINT ( 'NONE',  ( 6.123233995736766282E-16, 6.000000000000000888, 6.000000000000005329 ) ) ;
#7647=CYLINDRICAL_SURFACE ( 'NONE', #298, 1.000000000000000888 ) ;
#7649=CARTESIAN_POINT ( 'NONE',  ( -3.311384659207106118, -5.004923837169439338, 10.52641404563304839 ) ) ;
#7650=EDGE_CURVE ( 'NONE', #6002, #4153, #53, .T. ) ;
#7651=CARTESIAN_POINT ( 'NONE',  ( -6.155867707731072613, -1.081837891426109310, 25.00436969680152188 ) ) ;
#7653=CARTESIAN_POINT ( 'NONE',  ( 6.021135683317715426, -1.680226122398147615, 10.52622717124729590 ) ) ;
#7654=CARTESIAN_POINT ( 'NONE',  ( 3.632753594129258801, 4.777047695051034992, 12.49995053646221166 ) ) ;
#7660=DIRECTION ( 'NONE',  ( 0.9510565162951500895, 0.3090169943749582204, 0.000000000000000000 ) ) ;
#7662=EDGE_LOOP ( 'NONE', ( #336, #6910 ) ) ;
#7664=CARTESIAN_POINT ( 'NONE',  ( 0.2619456584322226722, -5.995505046955614148, 30.02607193928647433 ) ) ;
#7665=CARTESIAN_POINT ( 'NONE',  ( -0.9740856415299394833, 6.173834621338617268, 17.73852653055527995 ) ) ;
#7666=CARTESIAN_POINT ( 'NONE',  ( 5.558508435838239059, -2.857531096718835428, 31.00000000000000000 ) ) ;
#7669=CARTESIAN_POINT ( 'NONE',  ( -5.725684683139646403, 2.507514573674684222, 5.798878384233398187 ) ) ;
#7670=CARTESIAN_POINT ( 'NONE',  ( 4.141923667210613225, 4.342011609040499209, 10.88438267301394724 ) ) ;
#7672=AXIS2_PLACEMENT_3D ( 'NONE', #14191, #6738, #14112 ) ;
#7678=CARTESIAN_POINT ( 'NONE',  ( -4.286401442266594586, 4.198423832313132209, 5.130649613488546201 ) ) ;
#7679=CARTESIAN_POINT ( 'NONE',  ( 2.817313151351126699, -5.579000502529464889, 11.36936067245786397 ) ) ;
#7680=CARTESIAN_POINT ( 'NONE',  ( -0.8736772044959963957, 6.188841968496059387, 4.496115732928120501 ) ) ;
#7681=CARTESIAN_POINT ( 'NONE',  ( 5.985119669071111481, 1.805077827356575737, 12.49991741810287138 ) ) ;
#7684=CARTESIAN_POINT ( 'NONE',  ( 3.421280866381043673, -4.930711975950980985, 23.49995067926686687 ) ) ;
#7690=FACE_BOUND ( 'NONE', #7042, .T. ) ;
#7694=AXIS2_PLACEMENT_3D ( 'NONE', #10527, #3129, #15381 ) ;
#7695=CARTESIAN_POINT ( 'NONE',  ( -4.344502777243535618, -4.493369211529261165, 10.99610786875028623 ) ) ;
#7698=CARTESIAN_POINT ( 'NONE',  ( 6.020822430078836440, -1.681351817312256802, 18.97408542334169823 ) ) ;
#7702=DIRECTION ( 'NONE',  ( 0.5877852522924802425, -0.8090169943749422332, 0.000000000000000000 ) ) ;
#7707=CARTESIAN_POINT ( 'NONE',  ( 5.317509234264000462, -2.779225709350912954, 11.36763921416086554 ) ) ;
#7708=CARTESIAN_POINT ( 'NONE',  ( -2.782769401326221193, 5.315896561274827015, 30.49571079637980375 ) ) ;
#7709=FACE_OUTER_BOUND ( 'NONE', #3742, .T. ) ;
#7711=ORIENTED_EDGE ( 'NONE', *, *, #13482, .F. ) ;
#7713=AXIS2_PLACEMENT_3D ( 'NONE', #2049, #13988, #4369 ) ;
#7716=VERTEX_POINT ( 'NONE', #12221 ) ;
#7717=DIRECTION ( 'NONE',  ( -0.9510565162951544194, 0.3090169943749447312, 0.000000000000000000 ) ) ;
#7718=DIRECTION ( 'NONE',  ( -0.3090169943749446202, -0.9510565162951544194, 0.000000000000000000 ) ) ;
#7719=EDGE_LOOP ( 'NONE', ( #5843, #12718, #432, #5262 ) ) ;
#7721=CARTESIAN_POINT ( 'NONE',  ( -0.6152055445544960532, 5.969096820685168225, 18.79904968670266996 ) ) ;
#7722=CARTESIAN_POINT ( 'NONE',  ( -0.2622538972263849244, 6.245673238944479344, 25.47385994369194862 ) ) ;
#7725=CARTESIAN_POINT ( 'NONE',  ( -4.267838854167249174, 4.217593933790261040, 17.73760108194402108 ) ) ;
#7727=DIRECTION ( 'NONE',  ( 0.9510565162951500895, 0.3090169943749582204, 0.000000000000000000 ) ) ;
#7729=CARTESIAN_POINT ( 'NONE',  ( -0.6139731865239675956, 6.220476368274055368, 30.19975545601933220 ) ) ;
#7730=VECTOR ( 'NONE', #443, 1000.000000000000000 ) ;
#7731=EDGE_LOOP ( 'NONE', ( #6387, #12114, #6689, #4887 ) ) ;
#7732=EDGE_LOOP ( 'NONE', ( #11298, #14966, #13167, #4151 ) ) ;
#7734=B_SPLINE_CURVE_WITH_KNOTS ( 'NONE', 3,
 ( #6141, #9721, #13208, #2301, #9638, #6059, #9872, #2548, #1187, #4944, #3812, #3733, #2465, #7171, #5018, #4782, #10820, #8449 ),
 .UNSPECIFIED., .F., .F.,
 ( 4, 2, 2, 2, 2, 2, 2, 2, 4 ),
 ( 0.000000000000000000, 0.0003914898357794974410, 0.0007829796715589948820, 0.001174469507338492431, 0.001565959343117989764, 0.001957449178897487096, 0.002348939014676984863, 0.002740428850456482195, 0.003131918686235979528 ),
 .UNSPECIFIED. ) ;
#7735=EDGE_LOOP ( 'NONE', ( #13126, #13366, #9544, #11335 ) ) ;
#7736=CARTESIAN_POINT ( 'NONE',  ( -5.558508435838157347, -2.857531096718993080, 11.49999999999998224 ) ) ;
#7737=CARTESIAN_POINT ( 'NONE',  ( 5.725930890718283983, 2.506952462184149688, 4.200668510924229437 ) ) ;
#7738=ORIENTED_EDGE ( 'NONE', *, *, #4191, .T. ) ;
#7739=CARTESIAN_POINT ( 'NONE',  ( -5.570820891630725136, -2.833901239560486562, 17.73763026556123634 ) ) ;
#7741=CARTESIAN_POINT ( 'NONE',  ( 2.817313151351089839, 5.579000502529481764, 31.00000000000000000 ) ) ;
#7743=CARTESIAN_POINT ( 'NONE',  ( -5.409007216690712383, 2.598315788643666302, 5.614425215719389683 ) ) ;
#7744=CARTESIAN_POINT ( 'NONE',  ( 6.081836621194449677, -1.445163676684796394, 30.12694108445700181 ) ) ;
#7747=CARTESIAN_POINT ( 'NONE',  ( 2.848727059635975056, 5.281416301279890035, 10.88557478428060499 ) ) ;
#7752=EDGE_LOOP ( 'NONE', ( #3192, #14014 ) ) ;
#7757=EDGE_CURVE ( 'NONE', #4447, #5302, #6760, .T. ) ;
#7758=CARTESIAN_POINT ( 'NONE',  ( -5.940390500375673177, 6.474944468551537824, 31.00000000000000000 ) ) ;
#7759=CARTESIAN_POINT ( 'NONE',  ( 0.5039005892421982713, -6.230833003620535493, 10.62636388911296415 ) ) ;
#7760=CARTESIAN_POINT ( 'NONE',  ( 5.935543223013879377, -0.8771126767605279539, 17.99999999999998934 ) ) ;
#7762=CARTESIAN_POINT ( 'NONE',  ( 2.668367453516523824, -5.373994336898184621, 24.36935038651144936 ) ) ;
#7768=DIRECTION ( 'NONE',  ( -0.3090169943749579429, 0.9510565162951502005, 0.000000000000000000 ) ) ;
#7776=CARTESIAN_POINT ( 'NONE',  ( -2.849269941562104780, 5.281123252783969768, 18.61519382448850024 ) ) ;
#7778=ORIENTED_EDGE ( 'NONE', *, *, #14325, .F. ) ;
#7779=CARTESIAN_POINT ( 'NONE',  ( -2.817313151351229727, -5.579000502529412486, 17.86762589283693359 ) ) ;
#7783=CARTESIAN_POINT ( 'NONE',  ( 6.176542424588118863, -0.9554180641285446862, 5.000000000000004441 ) ) ;
#7785=CYLINDRICAL_SURFACE ( 'NONE', #3248, 0.9999999999999998890 ) ;
#7786=CARTESIAN_POINT ( 'NONE',  ( -5.666074146198007533, -1.978051345703136121, 6.000049320733126912 ) ) ;
#7788=CARTESIAN_POINT ( 'NONE',  ( 5.558508435838322548, -2.857531096718671115, 24.36765874365829987 ) ) ;
#7789=CARTESIAN_POINT ( 'NONE',  ( -5.408775798201144624, -2.598833957129699002, 12.11397738943082558 ) ) ;
#7790=CARTESIAN_POINT ( 'NONE',  ( -5.330004929009548142, -2.755647751839476189, 11.23760108194400686 ) ) ;
#7793=ORIENTED_EDGE ( 'NONE', *, *, #14649, .T. ) ;
#7798=ORIENTED_EDGE ( 'NONE', *, *, #5282, .F. ) ;
#7800=CARTESIAN_POINT ( 'NONE',  ( -2.817313151351189315, 5.579000502529432026, 5.000000000000004441 ) ) ;
#7802=CARTESIAN_POINT ( 'NONE',  ( -0.6139731865237586517, 6.220476368274074019, 23.69975545601929667 ) ) ;
#7805=CARTESIAN_POINT ( 'NONE',  ( -2.782713018890612844, -5.315928322779175375, 10.99560239355786528 ) ) ;
#7807=FACE_OUTER_BOUND ( 'NONE', #11760, .T. ) ;
#7811=ORIENTED_EDGE ( 'NONE', *, *, #2500, .F. ) ;
#7813=ORIENTED_EDGE ( 'NONE', *, *, #1490, .F. ) ;
#7814=CARTESIAN_POINT ( 'NONE',  ( 2.996920846510471748, -5.485395142346797925, 18.61441947245482709 ) ) ;
#7815=CARTESIAN_POINT ( 'NONE',  ( 6.105747081304157220, 1.338335777572337015, 4.199734849823245852 ) ) ;
#7820=EDGE_CURVE ( 'NONE', #727, #14255, #8897, .T. ) ;
#7821=CARTESIAN_POINT ( 'NONE',  ( -2.997451966578434046, 5.485105005465995553, 31.61517780375841369 ) ) ;
#7822=CARTESIAN_POINT ( 'NONE',  ( 0.8730628416138880299, 6.188929913094940893, 17.49504929893120320 ) ) ;
#7824=CARTESIAN_POINT ( 'NONE',  ( 5.866817325727518906, -1.260653813891916997, 12.30022217383879024 ) ) ;
#7825=CARTESIAN_POINT ( 'NONE',  ( 2.692335458626835543, 5.362264153667240407, 11.23760108194400509 ) ) ;
#7830=AXIS2_PLACEMENT_3D ( 'NONE', #4930, #8519, #7390 ) ;
#7833=VECTOR ( 'NONE', #10530, 1000.000000000000114 ) ;
#7836=CARTESIAN_POINT ( 'NONE',  ( -3.883588957979326128, 4.898466244118876212, 17.02622717124729945 ) ) ;
#7838=CARTESIAN_POINT ( 'NONE',  ( -2.849573632035434123, 5.280958870664516525, 23.88438267301393125 ) ) ;
#7840=B_SPLINE_CURVE_WITH_KNOTS ( 'NONE', 3,
 ( #10980, #6764, #13904, #15189, #3016, #5491, #6530, #12557, #13669, #7634, #10335, #11518, #9151, #4287, #13986, #3092, #7788, #1656 ),
 .UNSPECIFIED., .F., .F.,
 ( 4, 2, 2, 2, 2, 2, 2, 2, 4 ),
 ( 0.003131486019301993329, 0.003522824630466700035, 0.003914163241631406741, 0.004305501852796113013, 0.004696840463960820153, 0.005088179075125527293, 0.005479517686290233565, 0.005870856297454939837, 0.006262194908619646977 ),
 .UNSPECIFIED. ) ;
#7843=CARTESIAN_POINT ( 'NONE',  ( 2.668367453516524268, -5.373994336898184621, 24.49999999999999289 ) ) ;
#7845=CARTESIAN_POINT ( 'NONE',  ( -4.290821322214424249, -4.545321419741505942, 18.61441947245482709 ) ) ;
#7848=LINE ( 'NONE', #2679, #10034 ) ;
#7853=PRODUCT_DEFINITION_CONTEXT ( 'detailed design', #10449, 'design' ) ;
#7854=CARTESIAN_POINT ( 'NONE',  ( 5.985119669071152337, -1.805077827356440734, 17.00008258189709309 ) ) ;
#7855=CARTESIAN_POINT ( 'NONE',  ( -4.291255145204043053, -4.544933371694706459, 10.88603820591927018 ) ) ;
#7856=EDGE_CURVE ( 'NONE', #9215, #7578, #15289, .T. ) ;
#7859=AXIS2_PLACEMENT_3D ( 'NONE', #4058, #5423, #4218 ) ;
#7861=CARTESIAN_POINT ( 'NONE',  ( -3.882673863916437540, 4.899192824800819857, 25.47408542334170178 ) ) ;
#7866=CARTESIAN_POINT ( 'NONE',  ( 3.011899281037277998, 5.190111395030357677, 25.30022217383879379 ) ) ;
#7870=DIRECTION ( 'NONE',  ( 0.8090169943749510040, -0.5877852522924683631, 0.000000000000000000 ) ) ;
#7872=DIRECTION ( 'NONE',  ( -0.9510565162951544194, 0.3090169943749447312, 0.000000000000000000 ) ) ;
#7874=CARTESIAN_POINT ( 'NONE',  ( 4.195795028114904568, 4.289273350251447070, 23.99571079637980020 ) ) ;
#7875=EDGE_LOOP ( 'NONE', ( #4556, #12892 ) ) ;
#7877=ORIENTED_EDGE ( 'NONE', *, *, #11259, .F. ) ;
#7881=CARTESIAN_POINT ( 'NONE',  ( -2.849573632035176995, -5.280958870664654192, 5.615617326986058977 ) ) ;
#7883=CARTESIAN_POINT ( 'NONE',  ( -2.841519077896070389, -5.566940434250053471, 5.263796168408048537 ) ) ;
#7886=CARTESIAN_POINT ( 'NONE',  ( -5.903843691985222186, -2.055287728870673902, 6.000049068765331839 ) ) ;
#7887=CARTESIAN_POINT ( 'NONE',  ( -3.011385983131474209, 5.190390249166348724, 17.20047945897284691 ) ) ;
#7889=CARTESIAN_POINT ( 'NONE',  ( 2.840966774240201609, 5.567223638426886723, 31.26190213084010239 ) ) ;
#7894=EDGE_LOOP ( 'NONE', ( #341, #8374 ) ) ;
#7895=CARTESIAN_POINT ( 'NONE',  ( 3.566234721238037864, -5.134387337253829564, 18.99991741810287493 ) ) ;
#7896=CARTESIAN_POINT ( 'NONE',  ( 6.172651332693080306, 0.9815532474594598211, 4.738097869159890507 ) ) ;
#7897=ORIENTED_EDGE ( 'NONE', *, *, #13872, .F. ) ;
#7898=CARTESIAN_POINT ( 'NONE',  ( 5.935543223013879377, -0.8771126767605279539, 17.99999999999998934 ) ) ;
#7900=CARTESIAN_POINT ( 'NONE',  ( -5.935543223013862502, 0.8771126767606655106, 5.132360785839114925 ) ) ;
#7902=CARTESIAN_POINT ( 'NONE',  ( 2.817313151351004130, -5.579000502529524397, 24.49999999999999289 ) ) ;
#7903=CARTESIAN_POINT ( 'NONE',  ( 4.005785023174413872, 4.467917056767434225, 10.70047945897283981 ) ) ;
#7910=VERTEX_POINT ( 'NONE', #10623 ) ;
#7911=CARTESIAN_POINT ( 'NONE',  ( -2.931212650151771015, 5.520239928492759240, 17.49574050496989841 ) ) ;
#7912=FACE_OUTER_BOUND ( 'NONE', #12212, .T. ) ;
#7915=CARTESIAN_POINT ( 'NONE',  ( 2.817313151351047207, 5.579000502529503080, 11.49999999999998224 ) ) ;
#7916=CARTESIAN_POINT ( 'NONE',  ( -0.9999171162587678907, -6.169494774098581935, 24.36722320330673242 ) ) ;
#7920=CARTESIAN_POINT ( 'NONE',  ( 2.668367453516627741, 5.373994336898131330, 4.869383044678627925 ) ) ;
#7924=FACE_BOUND ( 'NONE', #4890, .T. ) ;
#7925=CARTESIAN_POINT ( 'NONE',  ( 6.106056299406752430, -1.336851112280646348, 30.20112161576662047 ) ) ;
#7929=CARTESIAN_POINT ( 'NONE',  ( -3.458467055437442372, 5.207305717053728245, 25.47359571723300320 ) ) ;
#7930=CARTESIAN_POINT ( 'NONE',  ( -0.2638277032946870215, -5.995407492418050488, 25.47332055281518137 ) ) ;
#7933=ADVANCED_FACE ( 'NONE', ( #7209 ), #834, .F. ) ;
#7937=CARTESIAN_POINT ( 'NONE',  ( -5.317509234263873452, 2.779225709351156315, 24.49999999999999289 ) ) ;
#7945=CARTESIAN_POINT ( 'NONE',  ( 2.817313151351169331, -5.579000502529441796, 31.00000000000000000 ) ) ;
#7947=CARTESIAN_POINT ( 'NONE',  ( -3.311384659207082581, -5.004923837169455325, 30.02641404563305016 ) ) ;
#7950=CARTESIAN_POINT ( 'NONE',  ( -2.817313151351230172, -5.579000502529412486, 17.99999999999998934 ) ) ;
#7951=ADVANCED_FACE ( 'NONE', ( #2177 ), #13160, .F. ) ;
#7954=CARTESIAN_POINT ( 'NONE',  ( -7.490007020835642848, -2.433650805992559896, 24.49999999999999289 ) ) ;
#7956=EDGE_CURVE ( 'NONE', #5801, #8675, #10552, .T. ) ;
#7958=DIRECTION ( 'NONE',  ( -0.3090169943749446202, -0.9510565162951544194, 0.000000000000000000 ) ) ;
#7959=CARTESIAN_POINT ( 'NONE',  ( 3.780072143464109580, 4.979057943639827677, 16.99991780678442055 ) ) ;
#7965=DIRECTION ( 'NONE',  ( 0.000000000000000000, 1.000000000000000000, 0.000000000000000000 ) ) ;
#7966=CARTESIAN_POINT ( 'NONE',  ( 4.435347140100995844, 4.403429997944548369, 31.13237410716305575 ) ) ;
#7967=CARTESIAN_POINT ( 'NONE',  ( 4.005998022989905039, 4.467726698309312461, 12.29931806258173665 ) ) ;
#7969=ORIENTED_EDGE ( 'NONE', *, *, #12558, .F. ) ;
#7970=VERTEX_POINT ( 'NONE', #14194 ) ;
#7971=CARTESIAN_POINT ( 'NONE',  ( 2.817313151351065859, -5.579000502529494199, 17.99999999999998934 ) ) ;
#7975=VECTOR ( 'NONE', #4848, 1000.000000000000000 ) ;
#7978=CARTESIAN_POINT ( 'NONE',  ( 4.416779112813501662, 4.422345839825947422, 24.76225281721715632 ) ) ;
#7982=FACE_OUTER_BOUND ( 'NONE', #4712, .T. ) ;
#7990=CARTESIAN_POINT ( 'NONE',  ( 4.267936573529295785, -4.217499624512150547, 4.737709621640687097 ) ) ;
#7991=ORIENTED_EDGE ( 'NONE', *, *, #10365, .T. ) ;
#7992=CARTESIAN_POINT ( 'NONE',  ( 3.566234721238159544, -5.134387337253744299, 5.999917418102892697 ) ) ;
#7995=ORIENTED_EDGE ( 'NONE', *, *, #2542, .T. ) ;
#7997=FACE_BOUND ( 'NONE', #5023, .T. ) ;
#8002=DIRECTION ( 'NONE',  ( 0.9510565162951499785, 0.3090169943749582204, 0.000000000000000000 ) ) ;
#8006=UNCERTAINTY_MEASURE_WITH_UNIT (LENGTH_MEASURE( 1.000000000000000082E-05 ), #8244, 'distance_accuracy_value', 'NONE');
#8007=CARTESIAN_POINT ( 'NONE',  ( 5.935543223013858949, -0.8771126767606638452, 5.000000000000004441 ) ) ;
#8008=CARTESIAN_POINT ( 'NONE',  ( -5.842988226680554398, 1.369004370660755532, 18.87380682714709579 ) ) ;
#8012=CARTESIAN_POINT ( 'NONE',  ( 4.344265632482025907, -4.493596842505014344, 25.00425949503011225 ) ) ;
#8017=B_SPLINE_CURVE_WITH_KNOTS ( 'NONE', 3,
 ( #8874, #10137, #2574, #418, #13704, #2734, #14674, #3763, #14830, #3915, #12275, #6249, #13621, #11084, #7585, #8950, #11240, #185 ),
 .UNSPECIFIED., .F., .F.,
 ( 4, 2, 2, 2, 2, 2, 2, 2, 4 ),
 ( 0.003131923598876996603, 0.003523316383094313511, 0.003914709167311630419, 0.004306101951528947328, 0.004697494735746264236, 0.005088887519963581144, 0.005480280304180897184, 0.005871673088398214092, 0.006263065872615531000 ),
 .UNSPECIFIED. ) ;
#8018=CARTESIAN_POINT ( 'NONE',  ( -5.666074146197961348, 1.978051345703259578, 23.49995067926686687 ) ) ;
#8025=CARTESIAN_POINT ( 'NONE',  ( 5.649053410273064735, 2.675685104943274606, 10.88482219624156322 ) ) ;
#8027=DIRECTION ( 'NONE',  ( 0.000000000000000000, 0.000000000000000000, -1.000000000000000000 ) ) ;
#8030=EDGE_CURVE ( 'NONE', #14335, #2248, #15095, .T. ) ;
#8031=CARTESIAN_POINT ( 'NONE',  ( 5.558508435838253270, 2.857531096718811892, 17.99999999999998934 ) ) ;
#8032=EDGE_LOOP ( 'NONE', ( #14749, #13064, #13836, #490 ) ) ;
#8033=ADVANCED_FACE ( 'NONE', ( #10856 ), #14681, .F. ) ;
#8035=DIRECTION ( 'NONE',  ( 0.8090169943749421222, 0.5877852522924802425, 0.000000000000000000 ) ) ;
#8036=B_SPLINE_CURVE_WITH_KNOTS ( 'NONE', 3,
 ( #3905, #8780, #13609, #7651, #7344, #8860, #12499, #1597, #9739, #8552, #13376, #12186, #1285, #1675, #2958, #1988, #14077, #10277 ),
 .UNSPECIFIED., .F., .F.,
 ( 4, 2, 2, 2, 2, 2, 2, 2, 4 ),
 ( 0.000000000000000000, 0.0003914357524127481361, 0.0007828715048254962722, 0.001174307257238244463, 0.001565743009650992544, 0.001957178762063741927, 0.002348614514476491527, 0.002740050266889241127, 0.003131486019301990727 ),
 .UNSPECIFIED. ) ;
#8037=CARTESIAN_POINT ( 'NONE',  ( -3.923477796648489058, -4.541042560386503446, 5.873037790270514868 ) ) ;
#8041=CARTESIAN_POINT ( 'NONE',  ( 5.409423237179108668, -2.597448116730828982, 23.88438267301394191 ) ) ;
#8043=CARTESIAN_POINT ( 'NONE',  ( -5.558508435838188433, -2.857531096718932684, 5.000000000000004441 ) ) ;
#8050=ORIENTED_EDGE ( 'NONE', *, *, #1073, .F. ) ;
#8051=VERTEX_POINT ( 'NONE', #3615 ) ;
#8052=CARTESIAN_POINT ( 'NONE',  ( 3.735808404764909163, -4.696639218303197083, 25.47398020122238904 ) ) ;
#8058=CARTESIAN_POINT ( 'NONE',  ( -5.621278735166214346, -2.101423246382510879, 31.97408052783100985 ) ) ;
#8067=DIRECTION ( 'NONE',  ( -0.5877852522924685852, -0.8090169943749508930, 0.000000000000000000 ) ) ;
#8069=CARTESIAN_POINT ( 'NONE',  ( 3.632753594129383146, -4.777047695050938181, 4.000049463537775907 ) ) ;
#8070=EDGE_CURVE ( 'NONE', #5942, #567, #13748, .T. ) ;
#8072=VERTEX_POINT ( 'NONE', #2661 ) ;
#8073=CARTESIAN_POINT ( 'NONE',  ( 2.996920846510591208, -5.485395142346733977, 5.614419472454843962 ) ) ;
#8076=CARTESIAN_POINT ( 'NONE',  ( 6.176542424588109093, 0.9554180641286111886, 31.00000000000000000 ) ) ;
#8077=EDGE_LOOP ( 'NONE', ( #10359, #5184 ) ) ;
#8078=CARTESIAN_POINT ( 'NONE',  ( -5.935543223013842073, 0.8771126767608004027, 17.86760611998364823 ) ) ;
#8081=CARTESIAN_POINT ( 'NONE',  ( -4.435347140101107755, -4.403429997944436458, 17.99999999999998934 ) ) ;
#8083=CARTESIAN_POINT ( 'NONE',  ( -2.668367453516648169, -5.373994336898122448, 31.13236078583911137 ) ) ;
#8084=FILL_AREA_STYLE ('',( #757 ) ) ;
#8091=DIRECTION ( 'NONE',  ( -1.000000000000000000, 0.000000000000000000, 0.000000000000000000 ) ) ;
#8092=LINE ( 'NONE', #4270, #6462 ) ;
#8094=EDGE_CURVE ( 'NONE', #860, #13214, #11094, .T. ) ;
#8097=EDGE_CURVE ( 'NONE', #6042, #7463, #2580, .T. ) ;
#8099=VERTEX_POINT ( 'NONE', #9759 ) ;
#8100=CARTESIAN_POINT ( 'NONE',  ( -5.615811513734980664, 2.743665920700508742, 18.50308643866043568 ) ) ;
#8105=DIRECTION ( 'NONE',  ( 0.9510565162951500895, 0.3090169943749582204, 0.000000000000000000 ) ) ;
#8109=CARTESIAN_POINT ( 'NONE',  ( 6.155912734541126419, 1.081577393120926711, 10.99610786875027735 ) ) ;
#8111=B_SPLINE_CURVE_WITH_KNOTS ( 'NONE', 3,
 ( #10739, #10658, #15599, #7247, #13357, #2216, #10900, #11838, #4617, #7168, #4940, #7325, #6139, #12006, #15678, #5973, #1184, #10817 ),
 .UNSPECIFIED., .F., .F.,
 ( 4, 2, 2, 2, 2, 2, 2, 2, 4 ),
 ( 0.000000000000000000, 0.0003914898357794968989, 0.0007829796715589937978, 0.001174469507338490697, 0.001565959343117987596, 0.001957449178897484494, 0.002348939014676981393, 0.002740428850456478292, 0.003131918686235975191 ),
 .UNSPECIFIED. ) ;
#8112=CARTESIAN_POINT ( 'NONE',  ( 0.6144377077730162062, 5.969178481556063787, 30.20033966857735663 ) ) ;
#8113=ORIENTED_EDGE ( 'NONE', *, *, #4484, .T. ) ;
#8115=CARTESIAN_POINT ( 'NONE',  ( 4.286401442266519091, 4.198423832313208592, 30.86763921416088863 ) ) ;
#8116=ORIENTED_EDGE ( 'NONE', *, *, #12161, .T. ) ;
#8117=FACE_OUTER_BOUND ( 'NONE', #10206, .T. ) ;
#8119=CARTESIAN_POINT ( 'NONE',  ( 3.882809187878849322, 4.899079348630116293, 17.02599901976669017 ) ) ;
#8121=CARTESIAN_POINT ( 'NONE',  ( -0.8738043859789326184, 6.188821459035897199, 25.00341560223737503 ) ) ;
#8123=CARTESIAN_POINT ( 'NONE',  ( 4.195842658231499378, -4.289229542213141677, 10.99560239355786173 ) ) ;
#8126=CARTESIAN_POINT ( 'NONE',  ( -5.903057025253884760, -1.078199533779625963, 17.38438267301393481 ) ) ;
#8129=EDGE_LOOP ( 'NONE', ( #14333, #7162, #243, #6480 ) ) ;
#8130=VERTEX_POINT ( 'NONE', #3692 ) ;
#8131=EDGE_LOOP ( 'NONE', ( #411, #8315, #7275, #11981 ) ) ;
#8132=CARTESIAN_POINT ( 'NONE',  ( 4.344265632482128048, -4.493596842504916644, 12.00425949503009093 ) ) ;
#8133=FACE_OUTER_BOUND ( 'NONE', #13580, .T. ) ;
#8134=EDGE_LOOP ( 'NONE', ( #698, #6463, #2210, #12366 ) ) ;
#8138=CARTESIAN_POINT ( 'NONE',  ( -5.317509234263920526, -2.779225709351067053, 31.00000000000000000 ) ) ;
#8140=CARTESIAN_POINT ( 'NONE',  ( 4.435347140100866170, 4.403429997944679819, 24.49999999999999289 ) ) ;
#8143=EDGE_CURVE ( 'NONE', #3740, #13757, #1808, .T. ) ;
#8147=LINE ( 'NONE', #5683, #7833 ) ;
#8149=CARTESIAN_POINT ( 'NONE',  ( 2.817313151350985034, 5.579000502529535943, 18.13063932754211649 ) ) ;
#8150=B_SPLINE_CURVE_WITH_KNOTS ( 'NONE', 3,
 ( #1287, #99, #13304, #8226, #7271, #4884, #13227, #6161, #5917, #15701, #973, #4723, #7032, #4966, #10764, #2241, #7112, #11948 ),
 .UNSPECIFIED., .F., .F.,
 ( 4, 2, 2, 2, 2, 2, 2, 2, 4 ),
 ( 0.000000000000000000, 0.0003914357524127478108, 0.0007828715048254956217, 0.001174307257238243378, 0.001565743009650992328, 0.001957178762063741060, 0.002348614514476489792, 0.002740050266889238959, 0.003131486019301987257 ),
 .UNSPECIFIED. ) ;
#8152=CARTESIAN_POINT ( 'NONE',  ( -5.317509234263873452, 2.779225709351156315, 24.63061695532138629 ) ) ;
#8153=ORIENTED_EDGE ( 'NONE', *, *, #364, .F. ) ;
#8154=CARTESIAN_POINT ( 'NONE',  ( 0.000000000000000000, 6.250000000000000888, 12.49999999999998401 ) ) ;
#8155=CARTESIAN_POINT ( 'NONE',  ( 4.142173849413723907, -4.341773579105426606, 17.38480617551147844 ) ) ;
#8156=CARTESIAN_POINT ( 'NONE',  ( 5.570760634536855882, 2.834026536768143423, 24.23774718278285789 ) ) ;
#8157=EDGE_LOOP ( 'NONE', ( #10056, #2772, #8212, #9421 ) ) ;
#8158=CARTESIAN_POINT ( 'NONE',  ( 3.253823204785082357, 5.337590213880527124, 10.62694108445697339 ) ) ;
#8160=CARTESIAN_POINT ( 'NONE',  ( -3.159082487394832217, -5.393634094348301211, 18.79954462468841569 ) ) ;
#8163=SURFACE_STYLE_USAGE ( .BOTH. , #2261 ) ;
#8166=B_SPLINE_CURVE_WITH_KNOTS ( 'NONE', 3,
 ( #60, #4926, #13427, #9781, #14627, #3716, #3946, #2922, #10245, #11274, #8820, #12383, #13650, #12698, #9061, #5241, #12543, #7619 ),
 .UNSPECIFIED., .F., .F.,
 ( 4, 2, 2, 2, 2, 2, 2, 2, 4 ),
 ( 0.000000000000000000, 0.0003914357524127498708, 0.0007828715048254997417, 0.001174307257238249667, 0.001565743009650999483, 0.001957178762063747999, 0.002348614514476496298, 0.002740050266889245030, 0.003131486019301993329 ),
 .UNSPECIFIED. ) ;
#8168=CARTESIAN_POINT ( 'NONE',  ( 5.486982057989171047, 2.429327048029922942, 10.70068193741825802 ) ) ;
#8169=CARTESIAN_POINT ( 'NONE',  ( -5.409007216690653763, 2.598315788643790203, 18.61442521571937192 ) ) ;
#8172=CARTESIAN_POINT ( 'NONE',  ( -4.291255145204205590, 4.544933371694557245, 25.11396179408071205 ) ) ;
#8173=B_SPLINE_CURVE_WITH_KNOTS ( 'NONE', 3,
 ( #15597, #4698, #3105, #11836, #6288, #13202, #3572, #7396, #14475, #8362, #8443, #10973, #2378, #1413, #13279, #13509, #9867, #6054 ),
 .UNSPECIFIED., .F., .F.,
 ( 4, 2, 2, 2, 2, 2, 2, 2, 4 ),
 ( 0.003131490185286017660, 0.003522829482338626830, 0.003914168779391236433, 0.004305508076443845603, 0.004696847373496454772, 0.005088186670549063942, 0.005479525967601673112, 0.005870865264654282281, 0.006262204561706891451 ),
 .UNSPECIFIED. ) ;
#8175=EDGE_LOOP ( 'NONE', ( #5901, #13759 ) ) ;
#8177=CARTESIAN_POINT ( 'NONE',  ( -6.081509788407727157, 1.446521464462764417, 18.87381964045070859 ) ) ;
#8178=ORIENTED_EDGE ( 'NONE', *, *, #4656, .F. ) ;
#8179=B_SPLINE_CURVE_WITH_KNOTS ( 'NONE', 3,
 ( #13974, #11584, #6751, #6673, #682, #3230, #3312, #7929, #11743, #15496, #7861, #1876, #5633, #8172, #13012, #5555, #14048, #2112 ),
 .UNSPECIFIED., .F., .F.,
 ( 4, 2, 2, 2, 2, 2, 2, 2, 4 ),
 ( 0.000000000000000000, 0.0003914357524127493287, 0.0007828715048254986575, 0.001174307257238248149, 0.001565743009650997315, 0.001957178762063746698, 0.002348614514476494563, 0.002740050266889243295, 0.003131486019301991160 ),
 .UNSPECIFIED. ) ;
#8180=CARTESIAN_POINT ( 'NONE',  ( -5.935543223013831415, 0.8771126767608680153, 24.49999999999999289 ) ) ;
#8182=ADVANCED_FACE ( 'NONE', ( #8958 ), #10065, .F. ) ;
#8187=CARTESIAN_POINT ( 'NONE',  ( 6.081590040723071411, 1.446205118473034013, 10.62632671364004722 ) ) ;
#8188=CARTESIAN_POINT ( 'NONE',  ( 5.131373506000491247, 7.062729720844170167, 17.99999999999998934 ) ) ;
#8190=CARTESIAN_POINT ( 'NONE',  ( 2.094888807778566729E-14, 6.000000000000000888, 30.00000000000000000 ) ) ;
#8195=CARTESIAN_POINT ( 'NONE',  ( -0.7993282387950335632, 5.947240459526521583, 12.11484358216956991 ) ) ;
#8197=DIRECTION ( 'NONE',  ( -0.3090169943749446202, -0.9510565162951544194, 0.000000000000000000 ) ) ;
#8204=CARTESIAN_POINT ( 'NONE',  ( -5.648794263291753381, -2.676232015153594102, 4.385580527545152485 ) ) ;
#8206=CARTESIAN_POINT ( 'NONE',  ( 0.5043776560897653694, -6.230795654995838539, 31.87337476296011474 ) ) ;
#8208=CARTESIAN_POINT ( 'NONE',  ( 5.843318061569051203, 1.367618216965616362, 12.37303779027049089 ) ) ;
#8210=VECTOR ( 'NONE', #12978, 1000.000000000000000 ) ;
#8212=ORIENTED_EDGE ( 'NONE', *, *, #4484, .F. ) ;
#8214=FACE_OUTER_BOUND ( 'NONE', #1664, .T. ) ;
#8217=CARTESIAN_POINT ( 'NONE',  ( -0.5044069930201257046, 5.979990686695010105, 25.37335743227903606 ) ) ;
#8218=CARTESIAN_POINT ( 'NONE',  ( -4.435347140101012720, -4.403429997944533270, 4.869360672457872852 ) ) ;
#8220=VECTOR ( 'NONE', #13903, 1000.000000000000114 ) ;
#8223=CARTESIAN_POINT ( 'NONE',  ( 6.143020266950980357, -1.155160780047701508, 4.385580527545153373 ) ) ;
#8226=CARTESIAN_POINT ( 'NONE',  ( 4.344313232727158969, -4.493553492990063347, 30.49563030319846391 ) ) ;
#8230=CARTESIAN_POINT ( 'NONE',  ( -5.531209434046284734, 2.328189801702745587, 25.37303779027051220 ) ) ;
#8231=VERTEX_POINT ( 'NONE', #5296 ) ;
#8233=VERTEX_POINT ( 'NONE', #14914 ) ;
#8235=CARTESIAN_POINT ( 'NONE',  ( -6.105861027178947076, -1.337741388556997313, 30.20045537531156654 ) ) ;
#8236=CARTESIAN_POINT ( 'NONE',  ( 0.5039005892421229982, -6.230833003620540822, 4.126363889112978356 ) ) ;
#8238=CARTESIAN_POINT ( 'NONE',  ( -5.375763363753407909, 2.665284979407616550, 17.49610204984017159 ) ) ;
#8240=CARTESIAN_POINT ( 'NONE',  ( -0.1306070469491344976, -6.250000000000003553, 23.49999999999998934 ) ) ;
#8242=CARTESIAN_POINT ( 'NONE',  ( -5.558508435838095174, -2.857531096719115649, 24.49999999999999289 ) ) ;
#8243=CARTESIAN_POINT ( 'NONE',  ( 2.030576276931546336E-13, -6.000000000000000888, 25.49999999999999645 ) ) ;
#8244=( LENGTH_UNIT ( ) NAMED_UNIT ( * ) SI_UNIT ( .MILLI., .METRE. ) );
#8248=CARTESIAN_POINT ( 'NONE',  ( -6.155867707731084160, -1.081837891426048248, 18.50436969680152899 ) ) ;
#8250=CARTESIAN_POINT ( 'NONE',  ( 5.915755444410793373, 1.003187219519900752, 31.50312048902375395 ) ) ;
#8251=ORIENTED_EDGE ( 'NONE', *, *, #11861, .T. ) ;
#8253=DIRECTION ( 'NONE',  ( 0.000000000000000000, 1.000000000000000000, 0.000000000000000000 ) ) ;
#8254=ORIENTED_EDGE ( 'NONE', *, *, #160, .T. ) ;
#8256=DIRECTION ( 'NONE',  ( 0.8090169943749421222, 0.5877852522924802425, 0.000000000000000000 ) ) ;
#8257=VECTOR ( 'NONE', #8304, 1000.000000000000000 ) ;
#8260=CARTESIAN_POINT ( 'NONE',  ( 5.571002711501470195, 2.833546409886167350, 24.76379616840807074 ) ) ;
#8261=EDGE_CURVE ( 'NONE', #8538, #4157, #9601, .T. ) ;
#8265=FACE_BOUND ( 'NONE', #13703, .T. ) ;
#8266=B_SPLINE_CURVE_WITH_KNOTS ( 'NONE', 3,
 ( #5640, #11593, #6607, #855, #5721, #15420, #2938, #10491, #12632, #1731, #12711, #11679, #1810, #541, #617, #15262, #5489, #5410 ),
 .UNSPECIFIED., .F., .F.,
 ( 4, 2, 2, 2, 2, 2, 2, 2, 4 ),
 ( 0.000000000000000000, 0.0003914904498596298880, 0.0007829808997192597760, 0.001174471349578889772, 0.001565961799438519552, 0.001957452249298139140, 0.002348942699157758728, 0.002740433149017377883, 0.003131923598876997471 ),
 .UNSPECIFIED. ) ;
#8271=CARTESIAN_POINT ( 'NONE',  ( -0.1306497350716639139, 6.000000000000002665, 10.49999999999998224 ) ) ;
#8273=VERTEX_POINT ( 'NONE', #651 ) ;
#8274=EDGE_CURVE ( 'NONE', #15705, #860, #11862, .T. ) ;
#8275=EDGE_CURVE ( 'NONE', #5575, #8394, #736, .T. ) ;
#8277=CARTESIAN_POINT ( 'NONE',  ( -4.005361199355036206, 4.468319061418737803, 31.80022217383877248 ) ) ;
#8278=CARTESIAN_POINT ( 'NONE',  ( -2.668367453516768517, 5.373994336898062052, 11.49999999999998224 ) ) ;
#8281=CARTESIAN_POINT ( 'NONE',  ( 3.312524433819702185, 5.004191858254053216, 18.97408052783099563 ) ) ;
#8283=CARTESIAN_POINT ( 'NONE',  ( 2.848235266351003325, -5.281699484015657475, 10.88602261056917442 ) ) ;
#8285=CARTESIAN_POINT ( 'NONE',  ( 0.8736772044960189332, -6.188841968496057611, 30.49611573292811428 ) ) ;
#8287=CARTESIAN_POINT ( 'NONE',  ( -0.5031281619706412522, -5.980084330432680950, 17.12602272744524257 ) ) ;
#8289=VERTEX_POINT ( 'NONE', #9570 ) ;
#8291=CARTESIAN_POINT ( 'NONE',  ( 2.930600586412946740, 5.520563544161762870, 30.49691356133955011 ) ) ;
#8293=ORIENTED_EDGE ( 'NONE', *, *, #8473, .F. ) ;
#8296=CARTESIAN_POINT ( 'NONE',  ( 0.8737888311110059147, -5.936248257219507884, 5.503441851412170571 ) ) ;
#8297=CARTESIAN_POINT ( 'NONE',  ( 4.153663429050612699, 4.670992970568521585, 25.29933148907577944 ) ) ;
#8300=LINE ( 'NONE', #6799, #9985 ) ;
#8302=CARTESIAN_POINT ( 'NONE',  ( 3.459597053047918980, -5.206576120509697425, 4.025914576658297328 ) ) ;
#8304=DIRECTION ( 'NONE',  ( 0.000000000000000000, 1.000000000000000000, 0.000000000000000000 ) ) ;
#8306=B_SPLINE_CURVE_WITH_KNOTS ( 'NONE', 3,
 ( #4861, #13115, #2380, #4779, #1263, #3334, #6056, #1028, #14390, #11923, #8281, #4700, #2462, #1109, #9470, #12085, #9552, #7087 ),
 .UNSPECIFIED., .F., .F.,
 ( 4, 2, 2, 2, 2, 2, 2, 2, 4 ),
 ( 0.000000000000000000, 0.0003914898357794968447, 0.0007829796715589936893, 0.001174469507338490480, 0.001565959343117987379, 0.001957449178897484061, 0.002348939014676980960, 0.002740428850456477858, 0.003131918686235974757 ),
 .UNSPECIFIED. ) ;
#8307=ORIENTED_EDGE ( 'NONE', *, *, #9282, .F. ) ;
#8310=ORIENTED_EDGE ( 'NONE', *, *, #12029, .T. ) ;
#8311=CARTESIAN_POINT ( 'NONE',  ( 0.1306070469493592900, 6.250000000000000000, 29.99999999999999289 ) ) ;
#8312=EDGE_CURVE ( 'NONE', #7910, #2947, #8300, .T. ) ;
#8313=CARTESIAN_POINT ( 'NONE',  ( -2.997451966578516203, -5.485105005465951145, 23.88482219624157210 ) ) ;
#8314=CARTESIAN_POINT ( 'NONE',  ( -4.267838854167235851, -4.217593933790273475, 24.76239891805597182 ) ) ;
#8315=ORIENTED_EDGE ( 'NONE', *, *, #6913, .T. ) ;
#8316=CARTESIAN_POINT ( 'NONE',  ( -6.172552660730993068, 0.9821660343537826909, 31.26379616840805653 ) ) ;
#8317=CARTESIAN_POINT ( 'NONE',  ( -0.5042675786779248215, -6.230788509548839116, 5.873310683104476126 ) ) ;
#8320=CARTESIAN_POINT ( 'NONE',  ( 5.317509234263941842, 2.779225709351030638, 31.00000000000000000 ) ) ;
#8321=DIRECTION ( 'NONE',  ( -0.3090169943749584425, 0.9510565162951498674, 0.000000000000000000 ) ) ;
#8322=( NAMED_UNIT ( * ) SI_UNIT ( $, .STERADIAN. ) SOLID_ANGLE_UNIT ( ) );
#8326=CARTESIAN_POINT ( 'NONE',  ( 3.632753594129297880, 4.777047695051003018, 31.99995053646222942 ) ) ;
#8328=CARTESIAN_POINT ( 'NONE',  ( 5.783198643800752770, 1.602922020054757590, 31.97377823943293151 ) ) ;
#8330=CARTESIAN_POINT ( 'NONE',  ( -5.782947755040664717, 1.603807858343995640, 12.47398020122238194 ) ) ;
#8331=CARTESIAN_POINT ( 'NONE',  ( -0.6156307853268694341, -5.969051238897262301, 12.29870573410680201 ) ) ;
#8332=CARTESIAN_POINT ( 'NONE',  ( 5.621197618055745693, 2.101623592078328162, 25.47398020122238194 ) ) ;
#8336=ORIENTED_EDGE ( 'NONE', *, *, #14100, .F. ) ;
#8338=CARTESIAN_POINT ( 'NONE',  ( -4.142620314836288564, -4.341347824677590950, 5.614425215719389683 ) ) ;
#8342=EDGE_CURVE ( 'NONE', #278, #5925, #9491, .T. ) ;
#8346=ADVANCED_FACE ( 'NONE', ( #7982 ), #15461, .F. ) ;
#8348=CARTESIAN_POINT ( 'NONE',  ( -5.558508435838126260, -2.857531096719055252, 17.99999999999998934 ) ) ;
#8356=CARTESIAN_POINT ( 'NONE',  ( 5.903347812666377870, 1.076697810262441823, 23.88602261056918152 ) ) ;
#8360=CARTESIAN_POINT ( 'NONE',  ( 5.782895619916165408, -1.604017620858050330, 5.974080527831013399 ) ) ;
#8362=CARTESIAN_POINT ( 'NONE',  ( 1.000082492230778053, 6.169467968613697728, 11.63152538105394740 ) ) ;
#8364=VECTOR ( 'NONE', #3443, 1000.000000000000000 ) ;
#8365=CARTESIAN_POINT ( 'NONE',  ( 4.195795028115014702, -4.289273350251340489, 18.50428920362019980 ) ) ;
#8368=CARTESIAN_POINT ( 'NONE',  ( -5.858813228503648496, -2.179803269293280721, 4.026227171247319880 ) ) ;
#8371=CARTESIAN_POINT ( 'NONE',  ( -5.558508435838198203, 2.857531096718914476, 11.49999999999998224 ) ) ;
#8372=CARTESIAN_POINT ( 'NONE',  ( -5.842945980534674177, 1.369128644668844652, 30.12621569129737864 ) ) ;
#8373=EDGE_LOOP ( 'NONE', ( #13675, #14920, #11994, #1292 ) ) ;
#8374=ORIENTED_EDGE ( 'NONE', *, *, #11282, .F. ) ;
#8376=ORIENTED_EDGE ( 'NONE', *, *, #14362, .T. ) ;
#8378=EDGE_LOOP ( 'NONE', ( #2368, #6792, #3891, #2568 ) ) ;
#8381=CARTESIAN_POINT ( 'NONE',  ( -0.7993282387949094403, 5.947240459526536682, 25.11484358216957347 ) ) ;
#8384=B_SPLINE_CURVE_WITH_KNOTS ( 'NONE', 3,
 ( #4171, #13869, #7990, #12831, #2013, #1779, #12682, #3209, #8069, #6886, #6654, #11485, #588, #5766, #979, #13145, #4647, #4487 ),
 .UNSPECIFIED., .F., .F.,
 ( 4, 2, 2, 2, 2, 2, 2, 2, 4 ),
 ( 0.000000000000000000, 0.0003914898357794963568, 0.0007829796715589927136, 0.001174469507338489179, 0.001565959343117986511, 0.001957449178897483627, 0.002348939014676980960, 0.002740428850456478726, 0.003131918686235975625 ),
 .UNSPECIFIED. ) ;
#8389=ADVANCED_FACE ( 'NONE', ( #11712 ), #5680, .F. ) ;
#8390=CARTESIAN_POINT ( 'NONE',  ( 2.817313151351187983, -5.579000502529432026, 5.000000000000004441 ) ) ;
#8394=VERTEX_POINT ( 'NONE', #2081 ) ;
#8395=VERTEX_POINT ( 'NONE', #4562 ) ;
#8396=DIRECTION ( 'NONE',  ( 0.8090169943749506709, -0.5877852522924689183, 0.000000000000000000 ) ) ;
#8399=CARTESIAN_POINT ( 'NONE',  ( -6.176542424588102875, -0.9554180641286524889, 30.86765874365832119 ) ) ;
#8403=CARTESIAN_POINT ( 'NONE',  ( -7.180990026460683850, -3.384707322287710873, 24.49999999999999289 ) ) ;
#8405=CARTESIAN_POINT ( 'NONE',  ( 5.375913338529156427, -2.664979843780304058, 17.49571079637979665 ) ) ;
#8406=CARTESIAN_POINT ( 'NONE',  ( -0.1323408341372861174, -6.250000000000005329, 25.50000000000000355 ) ) ;
#8407=CARTESIAN_POINT ( 'NONE',  ( -4.291255145204106114, 4.544933371694646063, 12.11396179408069607 ) ) ;
#8408=CARTESIAN_POINT ( 'NONE',  ( 5.935543223013850955, 0.8771126767607274610, 30.86935038651144936 ) ) ;
#8409=CARTESIAN_POINT ( 'NONE',  ( -4.435347140101154828, -4.403429997944389385, 24.49999999999999289 ) ) ;
#8414=CARTESIAN_POINT ( 'NONE',  ( 5.903230462362950348, 1.077253041748909013, 31.61442521571937547 ) ) ;
#8415=EDGE_LOOP ( 'NONE', ( #10052, #11065 ) ) ;
#8417=CARTESIAN_POINT ( 'NONE',  ( 0.5039079366033171192, -5.980031194523144578, 10.62637068109811800 ) ) ;
#8421=DIRECTION ( 'NONE',  ( -0.9510565162951545304, 0.3090169943749447867, 0.000000000000000000 ) ) ;
#8422=CARTESIAN_POINT ( 'NONE',  ( 2.817313151350925526, 5.579000502529565253, 24.36939309276499799 ) ) ;
#8425=CARTESIAN_POINT ( 'NONE',  ( -0.5042675786779022840, -6.230788509548840892, 31.87331068310447790 ) ) ;
#8427=CARTESIAN_POINT ( 'NONE',  ( -2.817313151351189315, 5.579000502529432026, 5.000000000000004441 ) ) ;
#8431=CARTESIAN_POINT ( 'NONE',  ( 0.8738118504725876923, 5.936246475285029689, 31.50357242174242600 ) ) ;
#8432=ORIENTED_EDGE ( 'NONE', *, *, #6898, .F. ) ;
#8435=AXIS2_PLACEMENT_3D ( 'NONE', #664, #11492, #1863 ) ;
#8439=EDGE_CURVE ( 'NONE', #15704, #5008, #9208, .T. ) ;
#8441=FACE_BOUND ( 'NONE', #11004, .T. ) ;
#8443=CARTESIAN_POINT ( 'NONE',  ( 0.9740012993920699191, 6.173846968979631811, 11.76164920628442978 ) ) ;
#8445=CARTESIAN_POINT ( 'NONE',  ( 3.010624175977939299, -5.190832888732245465, 18.79888242247940155 ) ) ;
#8449=CARTESIAN_POINT ( 'NONE',  ( 5.935543223013862502, -0.8771126767606430841, 31.00000000000000000 ) ) ;
#8450=CARTESIAN_POINT ( 'NONE',  ( 0.6139731865240156683, -6.220476368274049150, 30.19975545601932865 ) ) ;
#8451=CARTESIAN_POINT ( 'NONE',  ( 5.409274167810623091, 2.597759609440709827, 4.384806175511482884 ) ) ;
#8452=CARTESIAN_POINT ( 'NONE',  ( 2.782156709077223677, 5.316215864844147099, 23.99687951097623184 ) ) ;
#8457=ORIENTED_EDGE ( 'NONE', *, *, #1564, .T. ) ;
#8459=CARTESIAN_POINT ( 'NONE',  ( -4.267992336621238891, 4.217442018459959030, 11.76194324003145120 ) ) ;
#8460=VERTEX_POINT ( 'NONE', #172 ) ;
#8468=B_SPLINE_CURVE_WITH_KNOTS ( 'NONE', 3,
 ( #7121, #14339, #2169, #2252, #8313, #11957, #10773, #7201, #2329, #3367, #15630, #4734, #12117, #3606, #5846, #13237, #12042, #9582 ),
 .UNSPECIFIED., .F., .F.,
 ( 4, 2, 2, 2, 2, 2, 2, 2, 4 ),
 ( 0.000000000000000000, 0.0003914357524127469435, 0.0007828715048254938870, 0.001174307257238240993, 0.001565743009650987774, 0.001957178762063734555, 0.002348614514476480251, 0.002740050266889226815, 0.003131486019301972078 ),
 .UNSPECIFIED. ) ;
#8469=CARTESIAN_POINT ( 'NONE',  ( -5.558508435838198203, 2.857531096718914476, 11.49999999999998224 ) ) ;
#8473=EDGE_CURVE ( 'NONE', #1512, #7319, #95, .T. ) ;
#8482=ORIENTED_EDGE ( 'NONE', *, *, #13524, .T. ) ;
#8483=CARTESIAN_POINT ( 'NONE',  ( -5.570820891630731353, 2.833901239560472796, 24.76236973443873524 ) ) ;
#8484=CARTESIAN_POINT ( 'NONE',  ( 2.668367453516585108, -5.373994336898155311, 17.86935038651144225 ) ) ;
#8485=CARTESIAN_POINT ( 'NONE',  ( 0.2619041840694849577, -6.245686665308502583, 4.026058494337955374 ) ) ;
#8487=CARTESIAN_POINT ( 'NONE',  ( -6.155867707731105476, -1.081837891425919462, 31.50436969680151833 ) ) ;
#8488=CARTESIAN_POINT ( 'NONE',  ( 3.159612573729145168, -5.393342049074681732, 23.69973484982322987 ) ) ;
#8489=CARTESIAN_POINT ( 'NONE',  ( -4.142620314836348960, -4.341347824677533218, 12.11442521571935238 ) ) ;
#8490=CARTESIAN_POINT ( 'NONE',  ( -3.458467055437342008, 5.207305717053796634, 12.47359571723300498 ) ) ;
#8493=CARTESIAN_POINT ( 'NONE',  ( 0.7993282387953127843, -5.947240459526482503, 25.11484358216956991 ) ) ;
#8497=CARTESIAN_POINT ( 'NONE',  ( -5.615973259022252861, -2.743340227996308389, 18.50389213124969956 ) ) ;
#8499=EDGE_LOOP ( 'NONE', ( #11376, #337 ) ) ;
#8500=DIRECTION ( 'NONE',  ( 0.000000000000000000, 0.000000000000000000, -1.000000000000000000 ) ) ;
#8501=CARTESIAN_POINT ( 'NONE',  ( 0.2619456584322786274, -5.995505046955611483, 10.52607193928646367 ) ) ;
#8503=ORIENTED_EDGE ( 'NONE', *, *, #14362, .F. ) ;
#8506=CARTESIAN_POINT ( 'NONE',  ( -4.286401442266640771, 4.198423832313082471, 11.49999999999998224 ) ) ;
#8508=CARTESIAN_POINT ( 'NONE',  ( -3.567258970016137010, 5.133675764669563435, 23.49991780678443121 ) ) ;
#8510=CARTESIAN_POINT ( 'NONE',  ( -6.142844459177239536, 1.156093792145192145, 12.11560192892920895 ) ) ;
#8514=CARTESIAN_POINT ( 'NONE',  ( 6.020822430078810683, 1.681351817312345842, 17.02591457665827690 ) ) ;
#8516=ORIENTED_EDGE ( 'NONE', *, *, #9736, .T. ) ;
#8519=DIRECTION ( 'NONE',  ( 0.9510565162951500895, 0.3090169943749582204, 0.000000000000000000 ) ) ;
#8520=VERTEX_POINT ( 'NONE', #8469 ) ;
#8523=EDGE_CURVE ( 'NONE', #14489, #3268, #14310, .T. ) ;
#8525=LINE ( 'NONE', #10814, #4414 ) ;
#8526=LINE ( 'NONE', #12239, #8857 ) ;
#8528=CARTESIAN_POINT ( 'NONE',  ( 3.106366801611956330, -5.134708448381311463, 18.87303779027049799 ) ) ;
#8530=CARTESIAN_POINT ( 'NONE',  ( 1.354942164306246880E-13, -6.000000000000000888, 16.99999999999998579 ) ) ;
#8532=CARTESIAN_POINT ( 'NONE',  ( -3.159082487394813565, 5.393634094348312757, 30.20045537531155944 ) ) ;
#8533=CARTESIAN_POINT ( 'NONE',  ( 5.665824935993584610, 1.978765057080994483, 4.000049463537776795 ) ) ;
#8537=EDGE_LOOP ( 'NONE', ( #15687, #6047 ) ) ;
#8538=VERTEX_POINT ( 'NONE', #11073 ) ;
#8539=CARTESIAN_POINT ( 'NONE',  ( -3.011139120916709988, 5.190534000030228690, 25.29931806258175087 ) ) ;
#8542=B_SPLINE_CURVE_WITH_KNOTS ( 'NONE', 3,
 ( #6905, #13007, #15330, #14045, #1873, #15171, #5552, #6748, #11581, #678, #11662, #6827, #15407, #15249, #4504, #10399, #6979, #3154 ),
 .UNSPECIFIED., .F., .F.,
 ( 4, 2, 2, 2, 2, 2, 2, 2, 4 ),
 ( 0.003131490185285879316, 0.003522829482338505399, 0.003914168779391132350, 0.004305508076443757999, 0.004696847373496385383, 0.005088186670549011033, 0.005479525967601636682, 0.005870865264654263199, 0.006262204561706889716 ),
 .UNSPECIFIED. ) ;
#8549=CARTESIAN_POINT ( 'NONE',  ( -5.746996058422787712, 1.729015645941882839, 32.00007961174476634 ) ) ;
#8552=CARTESIAN_POINT ( 'NONE',  ( -5.903843691985159126, -2.055287728870867525, 25.50004906876533184 ) ) ;
#8561=CARTESIAN_POINT ( 'NONE',  ( -6.020865209844592059, -1.681180471732148130, 30.02599901976670438 ) ) ;
#8564=CARTESIAN_POINT ( 'NONE',  ( -5.770167736194690811, -2.404664418229182754, 31.87367328635992081 ) ) ;
#8567=CARTESIAN_POINT ( 'NONE',  ( -2.782769401326190106, -5.315896561274842114, 12.00428920362018914 ) ) ;
#8569=CARTESIAN_POINT ( 'NONE',  ( 5.665824935993590827, 1.978765057080975387, 30.00004946353777413 ) ) ;
#8574=CARTESIAN_POINT ( 'NONE',  ( -5.935543223013847403, -0.8771126767607489993, 5.000000000000004441 ) ) ;
#8575=ADVANCED_FACE ( 'NONE', ( #2643 ), #3828, .F. ) ;
#8577=EDGE_LOOP ( 'NONE', ( #3568, #6501, #9082, #10983 ) ) ;
#8578=CARTESIAN_POINT ( 'NONE',  ( -5.531209434046333584, 2.328189801702630124, 12.37303779027049089 ) ) ;
#8584=CYLINDRICAL_SURFACE ( 'NONE', #8959, 1.000000000000000222 ) ;
#8587=CARTESIAN_POINT ( 'NONE',  ( -6.155854678529477653, 1.081900940642092523, 12.00425949503009626 ) ) ;
#8589=FACE_BOUND ( 'NONE', #8077, .T. ) ;
#8595=ORIENTED_EDGE ( 'NONE', *, *, #5524, .F. ) ;
#8598=CARTESIAN_POINT ( 'NONE',  ( 5.317509234264026219, 2.779225709350867213, 24.36760611998364823 ) ) ;
#8602=CARTESIAN_POINT ( 'NONE',  ( 2.030576276931546336E-13, -6.250000000000000888, 24.49999999999999289 ) ) ;
#8604=CARTESIAN_POINT ( 'NONE',  ( 5.915699123067165388, -1.003533581835512223, 5.503897950159859498 ) ) ;
#8607=CARTESIAN_POINT ( 'NONE',  ( 5.843075991566629490, -1.368655265450851033, 25.37364704684422634 ) ) ;
#8611=CARTESIAN_POINT ( 'NONE',  ( -5.866984344570847831, 1.259800266528558810, 10.70068193741824736 ) ) ;
#8613=CARTESIAN_POINT ( 'NONE',  ( -5.487348639458900834, 2.428538342494392488, 30.19977782616121331 ) ) ;
#8619=AXIS2_PLACEMENT_3D ( 'NONE', #9123, #12684, #3140 ) ;
#8621=CARTESIAN_POINT ( 'NONE',  ( -5.984595133899149211, -1.806709459528761164, 12.49995078984291830 ) ) ;
#8625=CARTESIAN_POINT ( 'NONE',  ( -5.915641100987835799, 1.003868594704728556, 31.50428920362020335 ) ) ;
#8627=CARTESIAN_POINT ( 'NONE',  ( 3.311576095066635972, -5.004818610361267517, 31.97377823943292086 ) ) ;
#8629=DIRECTION ( 'NONE',  ( 0.8090169943749506709, -0.5877852522924686962, 0.000000000000000000 ) ) ;
#8634=AXIS2_PLACEMENT_3D ( 'NONE', #5577, #5651, #787 ) ;
#8635=EDGE_LOOP ( 'NONE', ( #85, #1935, #7641, #1085 ) ) ;
#8637=CARTESIAN_POINT ( 'NONE',  ( -5.615811513734976224, -2.743665920700520733, 10.99691356133951992 ) ) ;
#8638=CARTESIAN_POINT ( 'NONE',  ( 4.069800786343786392, 4.744882212776837527, 4.126180359549290522 ) ) ;
#8639=EDGE_CURVE ( 'NONE', #14280, #1820, #14954, .T. ) ;
#8640=CARTESIAN_POINT ( 'NONE',  ( 0.9740012993920164064, 6.173846968979639804, 5.261649206284398694 ) ) ;
#8641=ADVANCED_FACE ( 'NONE', ( #14894 ), #2957, .F. ) ;
#8642=CARTESIAN_POINT ( 'NONE',  ( -5.615973259022300823, -2.743340227996212910, 31.50389213124968890 ) ) ;
#8646=CARTESIAN_POINT ( 'NONE',  ( 2.030576276931546336E-13, -6.250000000000000888, 24.49999999999999289 ) ) ;
#8656=CARTESIAN_POINT ( 'NONE',  ( -5.903843691985187547, 2.055287728870776487, 23.49995093123466461 ) ) ;
#8660=CARTESIAN_POINT ( 'NONE',  ( 7.347880431581855163E-16, -6.250000000000000888, 4.000000000000004441 ) ) ;
#8668=CARTESIAN_POINT ( 'NONE',  ( 6.155912734541138853, 1.081577393120855435, 17.49610786875029689 ) ) ;
#8669=ORIENTED_EDGE ( 'NONE', *, *, #5743, .F. ) ;
#8671=B_SPLINE_CURVE_WITH_KNOTS ( 'NONE', 3,
 ( #6050, #15595, #7394, #1975, #9547, #14384, #4936, #3490, #4857, #14550, #8360, #13198, #3725, #12236, #8604, #13660, #4038, #5165 ),
 .UNSPECIFIED., .F., .F.,
 ( 4, 2, 2, 2, 2, 2, 2, 2, 4 ),
 ( 0.000000000000000000, 0.0003914898357794944052, 0.0007829796715589888104, 0.001174469507338483324, 0.001565959343117977621, 0.001957449178897471918, 0.002348939014676966648, 0.002740428850456460945, 0.003131918686235955242 ),
 .UNSPECIFIED. ) ;
#8673=CARTESIAN_POINT ( 'NONE',  ( -3.567258970015958486, -5.133675764669688668, 12.50008219321555103 ) ) ;
#8675=VERTEX_POINT ( 'NONE', #4066 ) ;
#8677=DIRECTION ( 'NONE',  ( 0.000000000000000000, 0.000000000000000000, 1.000000000000000000 ) ) ;
#8680=CYLINDRICAL_SURFACE ( 'NONE', #10628, 1.000000000000000666 ) ;
#8684=CARTESIAN_POINT ( 'NONE',  ( -0.1323602877611954887, -6.000000000000003553, 32.00000000000000711 ) ) ;
#8686=CARTESIAN_POINT ( 'NONE',  ( 5.903230462362974329, -1.077253041748779783, 10.88557478428060676 ) ) ;
#8688=CARTESIAN_POINT ( 'NONE',  ( -5.915653884842693166, -1.003805156977521040, 12.00439760644213294 ) ) ;
#8689=CARTESIAN_POINT ( 'NONE',  ( -5.935543223013858949, 0.8771126767606857166, 31.00000000000000000 ) ) ;
#8692=ORIENTED_EDGE ( 'NONE', *, *, #6898, .T. ) ;
#8693=EDGE_LOOP ( 'NONE', ( #11202, #11408, #11542, #3263 ) ) ;
#8695=EDGE_LOOP ( 'NONE', ( #11890, #10694, #12913, #3640 ) ) ;
#8697=CARTESIAN_POINT ( 'NONE',  ( -5.903843691985196429, -2.055287728870748065, 12.50004906876531052 ) ) ;
#8698=CARTESIAN_POINT ( 'NONE',  ( 5.859155363331372435, 2.178872204145008151, 31.97400098023329917 ) ) ;
#8702=CARTESIAN_POINT ( 'NONE',  ( 3.922396193919089669, -4.541970110199406108, 31.87380682714711355 ) ) ;
#8704=CARTESIAN_POINT ( 'NONE',  ( 6.143020266950992792, -1.155160780047631786, 10.88558052754513206 ) ) ;
#8707=VECTOR ( 'NONE', #5931, 1000.000000000000000 ) ;
#8709=B_SPLINE_CURVE_WITH_KNOTS ( 'NONE', 3,
 ( #12124, #3298, #3613, #9511, #14264, #14192, #12996, #8490, #9588, #2420, #14432, #2100, #3536, #8407, #10699, #13242, #14345, #2258 ),
 .UNSPECIFIED., .F., .F.,
 ( 4, 2, 2, 2, 2, 2, 2, 2, 4 ),
 ( 0.000000000000000000, 0.0003914357524127503587, 0.0007828715048255007174, 0.001174307257238250968, 0.001565743009651001435, 0.001957178762063751468, 0.002348614514476503237, 0.002740050266889254571, 0.003131486019302005472 ),
 .UNSPECIFIED. ) ;
#8711=CARTESIAN_POINT ( 'NONE',  ( 5.621197618055712830, -2.101623592078419644, 30.02601979877761451 ) ) ;
#8713=CARTESIAN_POINT ( 'NONE',  ( 0.9737725088282187524, 6.173885267451822756, 4.737357587265641712 ) ) ;
#8714=CARTESIAN_POINT ( 'NONE',  ( -4.286401442266628337, -4.198423832313095794, 17.99999999999998934 ) ) ;
#8715=CARTESIAN_POINT ( 'NONE',  ( 5.940390500375550609, 6.474944468551622201, 5.000000000000004441 ) ) ;
#8718=CARTESIAN_POINT ( 'NONE',  ( 5.746619684944299422, -1.730157667110755026, 12.50004932073310471 ) ) ;
#8719=DIRECTION ( 'NONE',  ( 0.9510565162951500895, 0.3090169943749582204, 0.000000000000000000 ) ) ;
#8724=B_SPLINE_CURVE_WITH_KNOTS ( 'NONE', 3,
 ( #9509, #9429, #6678, #9586, #3372, #12045, #1144, #14343, #13895, #905, #5773, #3008, #7866, #14430, #3533, #11510, #14262, #13156 ),
 .UNSPECIFIED., .F., .F.,
 ( 4, 2, 2, 2, 2, 2, 2, 2, 4 ),
 ( 0.000000000000000000, 0.0003914898357794975494, 0.0007829796715589950988, 0.001174469507338492648, 0.001565959343117990198, 0.001957449178897487964, 0.002348939014676985296, 0.002740428850456482629, 0.003131918686235980395 ),
 .UNSPECIFIED. ) ;
#8725=ADVANCED_FACE ( 'NONE', ( #10045 ), #11383, .F. ) ;
#8727=ORIENTED_EDGE ( 'NONE', *, *, #10599, .T. ) ;
#8728=CARTESIAN_POINT ( 'NONE',  ( -6.081464507797620378, 1.446657058464248857, 17.12619944752603729 ) ) ;
#8730=CARTESIAN_POINT ( 'NONE',  ( -4.142620314836507056, 4.341347824677379563, 23.88557478428061387 ) ) ;
#8731=CARTESIAN_POINT ( 'NONE',  ( 5.725930890718287536, 2.506952462184140362, 30.20066851092423832 ) ) ;
#8733=CARTESIAN_POINT ( 'NONE',  ( 2.930600586412791309, 5.520563544161844582, 23.99691356133952524 ) ) ;
#8735=CARTESIAN_POINT ( 'NONE',  ( 5.903230462362961894, -1.077253041748847062, 4.385574784280630745 ) ) ;
#8740=EDGE_CURVE ( 'NONE', #2306, #5609, #1276, .T. ) ;
#8743=CARTESIAN_POINT ( 'NONE',  ( -2.841041022017357420, -5.567186575787277825, 11.23774718278287921 ) ) ;
#8746=CARTESIAN_POINT ( 'NONE',  ( -5.935543223013826086, -0.8771126767608832253, 17.99999999999998934 ) ) ;
#8750=CARTESIAN_POINT ( 'NONE',  ( -3.420659742068472120, -4.931142898501675198, 23.50004946353776702 ) ) ;
#8751=CARTESIAN_POINT ( 'NONE',  ( 5.558508435838260375, -2.857531096718794128, 11.63237410716304332 ) ) ;
#8755=CARTESIAN_POINT ( 'NONE',  ( 2.692335458626773370, 5.362264153667272382, 17.73760108194401752 ) ) ;
#8757=CARTESIAN_POINT ( 'NONE',  ( -4.435347140101010055, -4.403429997944535046, 5.000000000000004441 ) ) ;
#8758=CARTESIAN_POINT ( 'NONE',  ( -7.180990026460705167, -3.384707322287646480, 17.99999999999998934 ) ) ;
#8759=CARTESIAN_POINT ( 'NONE',  ( 1.354942164390165777E-13, -6.250000000000000888, 16.99999999999998579 ) ) ;
#8760=CARTESIAN_POINT ( 'NONE',  ( -5.903119516422464130, -1.077859910107564545, 12.11519382448850557 ) ) ;
#8765=ORIENTED_EDGE ( 'NONE', *, *, #4384, .F. ) ;
#8770=CARTESIAN_POINT ( 'NONE',  ( -3.632151824461228973, 4.777505256984487580, 25.50004932073311892 ) ) ;
#8771=ORIENTED_EDGE ( 'NONE', *, *, #5042, .T. ) ;
#8773=CARTESIAN_POINT ( 'NONE',  ( -6.176542424588096658, -0.9554180641287005615, 11.63237410716304687 ) ) ;
#8775=CARTESIAN_POINT ( 'NONE',  ( -0.6151877315909173305, 6.220340188096023404, 25.29906673469658784 ) ) ;
#8778=CARTESIAN_POINT ( 'NONE',  ( -3.634089073485536669, 4.776071126502611008, 17.00007997643736957 ) ) ;
#8780=CARTESIAN_POINT ( 'NONE',  ( -6.176542424588071789, -0.9554180641288338993, 24.63237410716305575 ) ) ;
#8782=CARTESIAN_POINT ( 'NONE',  ( -5.770167736194723673, 2.404664418229099265, 30.12632671364008274 ) ) ;
#8788=CARTESIAN_POINT ( 'NONE',  ( 5.531757352715602316, -2.326874507723326158, 30.12619317285288645 ) ) ;
#8791=ORIENTED_EDGE ( 'NONE', *, *, #939, .F. ) ;
#8794=CARTESIAN_POINT ( 'NONE',  ( 2.031800924177950305E-13, 6.000000000000000888, 23.49999999999999289 ) ) ;
#8795=CARTESIAN_POINT ( 'NONE',  ( 3.459597053047760440, -5.206576120509801342, 23.52591457665828756 ) ) ;
#8798=CARTESIAN_POINT ( 'NONE',  ( -6.020865209844624921, 1.681180471732039550, 5.974000980233303615 ) ) ;
#8799=CARTESIAN_POINT ( 'NONE',  ( 0.8737888311112075312, -5.936248257219478575, 25.00344185141216613 ) ) ;
#8805=ORIENTED_EDGE ( 'NONE', *, *, #14842, .T. ) ;
#8806=CARTESIAN_POINT ( 'NONE',  ( -6.142908455506932874, 1.155755562476104892, 17.38482219624156855 ) ) ;
#8807=CARTESIAN_POINT ( 'NONE',  ( 4.416779112813673080, -4.422345839825776892, 11.23774718278287743 ) ) ;
#8808=CARTESIAN_POINT ( 'NONE',  ( -2.668367453516892418, 5.373994336898001656, 24.49999999999999289 ) ) ;
#8809=CARTESIAN_POINT ( 'NONE',  ( 0.5042987395409762597, 5.979983180450060054, 25.37329304179976219 ) ) ;
#8810=B_SPLINE_CURVE_WITH_KNOTS ( 'NONE', 3,
 ( #6813, #11724, #5538, #4337, #1938, #10615, #593, #12687, #12835, #9194, #3213, #3293, #1784, #5694, #12916, #11648, #9424, #15475 ),
 .UNSPECIFIED., .F., .F.,
 ( 4, 2, 2, 2, 2, 2, 2, 2, 4 ),
 ( 0.000000000000000000, 0.0003914904498596247923, 0.0007829808997192495845, 0.001174471349578874377, 0.001565961799438499169, 0.001957452249298123961, 0.002348942699157748754, 0.002740433149017373546, 0.003131923598876998338 ),
 .UNSPECIFIED. ) ;
#8812=CARTESIAN_POINT ( 'NONE',  ( 3.254737477227991782, 5.337033878705210732, 5.873673286359927026 ) ) ;
#8815=CARTESIAN_POINT ( 'NONE',  ( 5.621197618055676415, 2.101623592078516012, 5.973980201222398811 ) ) ;
#8817=FACE_BOUND ( 'NONE', #6553, .T. ) ;
#8820=CARTESIAN_POINT ( 'NONE',  ( 6.020822430078855980, -1.681351817312188635, 25.47408542334170889 ) ) ;
#8821=B_SPLINE_CURVE_WITH_KNOTS ( 'NONE', 3,
 ( #6190, #15651, #11028, #126, #4753, #13875, #6348, #15010, #13563, #14848, #7448, #10231, #6428, #13726, #8809, #12292, #1630, #3858 ),
 .UNSPECIFIED., .F., .F.,
 ( 4, 2, 2, 2, 2, 2, 2, 2, 4 ),
 ( 0.003131923598876995302, 0.003523316383094312644, 0.003914709167311630419, 0.004306101951528947328, 0.004697494735746265103, 0.005088887519963582878, 0.005480280304180899786, 0.005871673088398216694, 0.006263065872615534470 ),
 .UNSPECIFIED. ) ;
#8822=VECTOR ( 'NONE', #14728, 1000.000000000000000 ) ;
#8825=CARTESIAN_POINT ( 'NONE',  ( 5.558508435838291462, -2.857531096718732400, 17.99999999999998934 ) ) ;
#8827=EDGE_LOOP ( 'NONE', ( #11622, #15295 ) ) ;
#8828=CARTESIAN_POINT ( 'NONE',  ( -2.692215568229842315, -5.362327947133593398, 17.73770962164069331 ) ) ;
#8833=CARTESIAN_POINT ( 'NONE',  ( 7.490007020835706797, -2.433650805992179755, 11.49999999999998224 ) ) ;
#8834=CARTESIAN_POINT ( 'NONE',  ( 4.267558728637101950, 4.217879122113895818, 17.73617396794403689 ) ) ;
#8839=DIRECTION ( 'NONE',  ( -0.9510565162951545304, 0.3090169943749447867, 0.000000000000000000 ) ) ;
#8844=VERTEX_POINT ( 'NONE', #15681 ) ;
#8845=CARTESIAN_POINT ( 'NONE',  ( -5.409007216690583597, -2.598315788643936308, 23.88557478428062097 ) ) ;
#8846=VECTOR ( 'NONE', #14406, 1000.000000000000000 ) ;
#8848=CARTESIAN_POINT ( 'NONE',  ( -3.311384659207313064, 5.004923837169304335, 25.47358595436692852 ) ) ;
#8850=ORIENTED_EDGE ( 'NONE', *, *, #15341, .T. ) ;
#8854=CARTESIAN_POINT ( 'NONE',  ( 6.250000000000000888, 7.654042494670958593E-16, 0.000000000000000000 ) ) ;
#8855=DIRECTION ( 'NONE',  ( -0.5877852522924685852, -0.8090169943749508930, 0.000000000000000000 ) ) ;
#8857=VECTOR ( 'NONE', #9550, 1000.000000000000000 ) ;
#8858=DIRECTION ( 'NONE',  ( 0.9510565162951500895, 0.3090169943749582204, 0.000000000000000000 ) ) ;
#8860=CARTESIAN_POINT ( 'NONE',  ( -6.105925084677645387, -1.337450587213346642, 25.29933148907576523 ) ) ;
#8862=CARTESIAN_POINT ( 'NONE',  ( 5.903472034603518992, -2.056448723545135859, 10.49991780678442410 ) ) ;
#8863=CARTESIAN_POINT ( 'NONE',  ( 3.736691294293371435, 4.695920479336417763, 12.47358595436692319 ) ) ;
#8864=ORIENTED_EDGE ( 'NONE', *, *, #652, .T. ) ;
#8867=EDGE_LOOP ( 'NONE', ( #1659, #9320, #2652, #6597 ) ) ;
#8871=CARTESIAN_POINT ( 'NONE',  ( 3.253823204785141421, 5.337590213880490708, 4.126941084456995590 ) ) ;
#8873=EDGE_LOOP ( 'NONE', ( #6576, #10358, #8376, #1914 ) ) ;
#8874=CARTESIAN_POINT ( 'NONE',  ( 7.347880347650999152E-16, -6.000000000000000888, 4.000000000000004441 ) ) ;
#8875=CARTESIAN_POINT ( 'NONE',  ( 0.9735954530126567086, -6.173909381473971614, 18.26281793585244984 ) ) ;
#8876=CARTESIAN_POINT ( 'NONE',  ( 0.000000000000000000, 6.250000000000000888, 18.99999999999998934 ) ) ;
#8881=CARTESIAN_POINT ( 'NONE',  ( -2.997753866155858038, 5.484939622623821620, 10.88439807107077861 ) ) ;
#8882=CARTESIAN_POINT ( 'NONE',  ( 2.782156709077347134, 5.316215864844083150, 10.99687951097621230 ) ) ;
#8889=ORIENTED_EDGE ( 'NONE', *, *, #8070, .T. ) ;
#8890=CARTESIAN_POINT ( 'NONE',  ( -3.632151824461058887, 4.777505256984618143, 6.000049320733126024 ) ) ;
#8891=CARTESIAN_POINT ( 'NONE',  ( 4.344313232727135876, -4.493553492990087328, 10.99563030319846924 ) ) ;
#8892=CARTESIAN_POINT ( 'NONE',  ( 0.2622538972264840673, -6.245673238944474015, 12.47385994369198059 ) ) ;
#8893=CARTESIAN_POINT ( 'NONE',  ( 6.172614129015234319, 0.9817721000788910413, 11.76236973443872991 ) ) ;
#8895=CARTESIAN_POINT ( 'NONE',  ( 2.996417732210567841, 5.485687819086908057, 5.613961794080714718 ) ) ;
#8897=LINE ( 'NONE', #5544, #2337 ) ;
#8899=CYLINDRICAL_SURFACE ( 'NONE', #14594, 0.9999999999999998890 ) ;
#8901=FACE_BOUND ( 'NONE', #4212, .T. ) ;
#8904=CARTESIAN_POINT ( 'NONE',  ( -2.817313151351170220, -5.579000502529442684, 11.36762589283694425 ) ) ;
#8907=CARTESIAN_POINT ( 'NONE',  ( -5.903119516422453472, -1.077859910107617836, 18.61519382448850024 ) ) ;
#8908=B_SPLINE_CURVE_WITH_KNOTS ( 'NONE', 3,
 ( #4320, #9488, #5753, #14171, #648, #885, #9256, #3352, #5600, #2078, #6876, #11709, #3276, #10368, #10446, #2153, #8218, #810 ),
 .UNSPECIFIED., .F., .F.,
 ( 4, 2, 2, 2, 2, 2, 2, 2, 4 ),
 ( 0.000000000000000000, 0.0003914357524127488950, 0.0007828715048254977901, 0.001174307257238246848, 0.001565743009650995580, 0.001957178762063744529, 0.002348614514476491961, 0.002740050266889240260, 0.003131486019301987691 ),
 .UNSPECIFIED. ) ;
#8911=CARTESIAN_POINT ( 'NONE',  ( -3.882673863916308754, -4.899192824800922885, 17.02591457665827690 ) ) ;
#8913=DIRECTION ( 'NONE',  ( -0.5877852522924685852, -0.8090169943749507819, 0.000000000000000000 ) ) ;
#8914=CARTESIAN_POINT ( 'NONE',  ( -5.935543223013862502, 0.8771126767606658436, 4.867606119983655333 ) ) ;
#8916=CARTESIAN_POINT ( 'NONE',  ( 6.176542424588125968, 0.9554180641284963915, 17.99999999999998934 ) ) ;
#8917=CARTESIAN_POINT ( 'NONE',  ( 4.267558728637259158, -4.217879122113739498, 5.263826032055956894 ) ) ;
#8918=CARTESIAN_POINT ( 'NONE',  ( -3.107583187530443602, 5.133966411712675537, 30.12619317285289000 ) ) ;
#8919=DIRECTION ( 'NONE',  ( -1.000000000000000000, 0.000000000000000000, 0.000000000000000000 ) ) ;
#8920=CARTESIAN_POINT ( 'NONE',  ( -5.746996058422751297, -1.729015645942007184, 10.49992038825521767 ) ) ;
#8921=VERTEX_POINT ( 'NONE', #13360 ) ;
#8926=EDGE_LOOP ( 'NONE', ( #9500, #2690 ) ) ;
#8927=DIRECTION ( 'NONE',  ( 0.5877852522924802425, -0.8090169943749422332, 0.000000000000000000 ) ) ;
#8931=CARTESIAN_POINT ( 'NONE',  ( 0.7995298244854619485, 5.947211616899248376, 5.614560146198583901 ) ) ;
#8936=EDGE_CURVE ( 'NONE', #15690, #6555, #7734, .T. ) ;
#8937=CARTESIAN_POINT ( 'NONE',  ( -4.286401442266582151, -4.198423832313145532, 11.36935038651143515 ) ) ;
#8940=CARTESIAN_POINT ( 'NONE',  ( 6.081836621194455006, -1.445163676684758425, 10.62694108445696806 ) ) ;
#8944=EDGE_LOOP ( 'NONE', ( #11815, #13027, #394, #11006 ) ) ;
#8945=B_SPLINE_CURVE_WITH_KNOTS ( 'NONE', 3,
 ( #12493, #4220, #6700, #5502, #7721, #11455, #10117, #5426, #6545, #1592, #6470, #5270, #11303, #11378, #558, #10271, #9089, #15201 ),
 .UNSPECIFIED., .F., .F.,
 ( 4, 2, 2, 2, 2, 2, 2, 2, 4 ),
 ( 0.000000000000000000, 0.0003914904498596247923, 0.0007829808997192493677, 0.001174471349578873943, 0.001565961799438498735, 0.001957452249298123528, 0.002348942699157747886, 0.002740433149017373112, 0.003131923598876997471 ),
 .UNSPECIFIED. ) ;
#8950=CARTESIAN_POINT ( 'NONE',  ( -0.2638277032948904699, -5.995407492418041606, 5.973320552815183149 ) ) ;
#8952=CARTESIAN_POINT ( 'NONE',  ( 0.8736516769107001146, -5.936271176698233454, 30.49606771578675435 ) ) ;
#8953=CARTESIAN_POINT ( 'NONE',  ( -4.435347140101089991, 4.403429997944455110, 31.13063932754212004 ) ) ;
#8958=FACE_OUTER_BOUND ( 'NONE', #7195, .T. ) ;
#8959=AXIS2_PLACEMENT_3D ( 'NONE', #3861, #11107, #13565 ) ;
#8963=VERTEX_POINT ( 'NONE', #9795 ) ;
#8965=EDGE_CURVE ( 'NONE', #1678, #7319, #5655, .T. ) ;
#8967=CARTESIAN_POINT ( 'NONE',  ( -5.770167736194681041, 2.404664418229203626, 17.12632671364005787 ) ) ;
#8968=CARTESIAN_POINT ( 'NONE',  ( 4.290381260516300088, -4.545736887716183894, 10.88482219624156144 ) ) ;
#8971=VECTOR ( 'NONE', #13687, 1000.000000000000000 ) ;
#8974=CARTESIAN_POINT ( 'NONE',  ( 3.107278289587092512, -5.134157760522109371, 23.62635295315576656 ) ) ;
#8977=CARTESIAN_POINT ( 'NONE',  ( 5.915755444410787156, 1.003187219519937168, 5.503120489023787698 ) ) ;
#8983=B_SPLINE_CURVE_WITH_KNOTS ( 'NONE', 3,
 ( #10314, #1559, #13734, #1790, #4185, #10080, #12614, #6666, #6586, #5316, #12377, #12693, #7611, #12458, #11268, #368, #10161, #15167 ),
 .UNSPECIFIED., .F., .F.,
 ( 4, 2, 2, 2, 2, 2, 2, 2, 4 ),
 ( 0.000000000000000000, 0.0003914357524127487866, 0.0007828715048254975733, 0.001174307257238246414, 0.001565743009650995147, 0.001957178762063744096, 0.002348614514476492828, 0.002740050266889241561, 0.003131486019301990293 ),
 .UNSPECIFIED. ) ;
#8984=CARTESIAN_POINT ( 'NONE',  ( -3.458467055437238091, -5.207305717053865912, 10.52640428276697371 ) ) ;
#8987=CARTESIAN_POINT ( 'NONE',  ( -4.286401442266688733, 4.198423832313033621, 17.99999999999998934 ) ) ;
#8988=EDGE_CURVE ( 'NONE', #15705, #3990, #9078, .T. ) ;
#8990=EDGE_LOOP ( 'NONE', ( #7056, #10131, #11508, #11118 ) ) ;
#8992=CARTESIAN_POINT ( 'NONE',  ( -2.668367453516752974, -5.373994336898072710, 17.86760611998364823 ) ) ;
#8997=CARTESIAN_POINT ( 'NONE',  ( 5.131373506000599605, 7.062729720844090231, 5.000000000000004441 ) ) ;
#8999=LINE ( 'NONE', #1889, #5715 ) ;
#9001=CARTESIAN_POINT ( 'NONE',  ( -5.317509234263900098, -2.779225709351108797, 11.49999999999998224 ) ) ;
#9002=EDGE_LOOP ( 'NONE', ( #12153, #9646 ) ) ;
#9006=CYLINDRICAL_SURFACE ( 'NONE', #4527, 1.000000000000000666 ) ;
#9008=DIRECTION ( 'NONE',  ( 0.9510565162951500895, 0.3090169943749582204, 0.000000000000000000 ) ) ;
#9012=CARTESIAN_POINT ( 'NONE',  ( 0.8738118504725739255, 5.936246475285030577, 5.503572421742425114 ) ) ;
#9015=EDGE_CURVE ( 'NONE', #3400, #11831, #184, .T. ) ;
#9016=CARTESIAN_POINT ( 'NONE',  ( -6.176542424588105540, -0.9554180641286327269, 5.000000000000004441 ) ) ;
#9019=CARTESIAN_POINT ( 'NONE',  ( 6.176542424588136626, 0.9554180641284277797, 24.49999999999999289 ) ) ;
#9021=CARTESIAN_POINT ( 'NONE',  ( -0.1306394121199157821, 6.250000000000001776, 30.00000000000000355 ) ) ;
#9024=EDGE_LOOP ( 'NONE', ( #2388, #13092 ) ) ;
#9025=ORIENTED_EDGE ( 'NONE', *, *, #11241, .T. ) ;
#9026=CARTESIAN_POINT ( 'NONE',  ( 4.435347140100978081, -4.403429997944567020, 18.13234125634167526 ) ) ;
#9028=VERTEX_POINT ( 'NONE', #463 ) ;
#9030=CARTESIAN_POINT ( 'NONE',  ( 0.2619041840696289536, -6.245686665308496366, 17.02605849433793850 ) ) ;
#9032=CARTESIAN_POINT ( 'NONE',  ( -5.746996058422793929, 1.729015645941861079, 6.000079611744768115 ) ) ;
#9033=CARTESIAN_POINT ( 'NONE',  ( 0.000000000000000000, 6.250000000000000888, 18.99999999999998934 ) ) ;
#9036=EDGE_CURVE ( 'NONE', #4157, #8538, #1304, .T. ) ;
#9037=DIRECTION ( 'NONE',  ( 0.8090169943749421222, 0.5877852522924802425, 0.000000000000000000 ) ) ;
#9043=CARTESIAN_POINT ( 'NONE',  ( -4.286401442266640771, 4.198423832313082471, 11.49999999999998224 ) ) ;
#9045=VERTEX_POINT ( 'NONE', #4072 ) ;
#9046=CARTESIAN_POINT ( 'NONE',  ( -0.1323736289504294505, 6.250000000000000000, 12.49999999999997335 ) ) ;
#9047=CARTESIAN_POINT ( 'NONE',  ( 7.490007020835748541, -2.433650805992050969, 24.49999999999999289 ) ) ;
#9048=CARTESIAN_POINT ( 'NONE',  ( -2.782769401326385061, 5.315896561274740861, 23.99571079637979665 ) ) ;
#9049=CARTESIAN_POINT ( 'NONE',  ( 5.616116467183629446, 2.743044348085603712, 12.00425949503009448 ) ) ;
#9051=CARTESIAN_POINT ( 'NONE',  ( 2.692143549875295250, -5.362363179736532537, 24.23805675996853992 ) ) ;
#9052=CARTESIAN_POINT ( 'NONE',  ( 3.459597053047814175, -5.206576120509766703, 17.02591457665827690 ) ) ;
#9055=CARTESIAN_POINT ( 'NONE',  ( -3.312341048453377734, -5.004306261885516527, 31.97398020122239259 ) ) ;
#9060=CARTESIAN_POINT ( 'NONE',  ( 6.155973317223314645, -1.081218830693557287, 17.49691356133953590 ) ) ;
#9061=CARTESIAN_POINT ( 'NONE',  ( 6.155912734541165499, -1.081577393120706887, 25.00389213124970311 ) ) ;
#9068=DIRECTION ( 'NONE',  ( 0.000000000000000000, 0.000000000000000000, -1.000000000000000000 ) ) ;
#9069=CARTESIAN_POINT ( 'NONE',  ( 5.783198643800806948, -1.602922020054565078, 17.02622176056705783 ) ) ;
#9076=CARTESIAN_POINT ( 'NONE',  ( -5.931817299736851901, -0.9033986943602198005, 5.262290378359327114 ) ) ;
#9078=LINE ( 'NONE', #8758, #8220 ) ;
#9079=CARTESIAN_POINT ( 'NONE',  ( 6.020822430078800025, -1.681351817312382702, 5.974085423341712442 ) ) ;
#9082=ORIENTED_EDGE ( 'NONE', *, *, #13102, .T. ) ;
#9085=LINE ( 'NONE', #2788, #2493 ) ;
#9086=ORIENTED_EDGE ( 'NONE', *, *, #8274, .T. ) ;
#9087=CARTESIAN_POINT ( 'NONE',  ( -5.935543223013831415, 0.8771126767608680153, 24.49999999999999289 ) ) ;
#9088=CARTESIAN_POINT ( 'NONE',  ( -5.842988226680558839, -1.369004370660723779, 30.12619317285289711 ) ) ;
#9089=CARTESIAN_POINT ( 'NONE',  ( -0.1306497350715971340, 6.000000000000004441, 16.99999999999998579 ) ) ;
#9090=CYLINDRICAL_SURFACE ( 'NONE', #4378, 1.000000000000000222 ) ;
#9092=CARTESIAN_POINT ( 'NONE',  ( 0.1306497350718684169, -6.000000000000000000, 16.99999999999998934 ) ) ;
#9093=CARTESIAN_POINT ( 'NONE',  ( -4.142620314836461759, 4.341347824677426637, 17.38557478428062097 ) ) ;
#9094=DIRECTION ( 'NONE',  ( -0.9510565162951544194, 0.3090169943749447312, 0.000000000000000000 ) ) ;
#9098=ORIENTED_EDGE ( 'NONE', *, *, #11370, .F. ) ;
#9100=EDGE_LOOP ( 'NONE', ( #13147, #1780 ) ) ;
#9101=CARTESIAN_POINT ( 'NONE',  ( 4.416397290909879203, -4.422724436066459930, 18.26379616840804943 ) ) ;
#9105=CARTESIAN_POINT ( 'NONE',  ( 5.915699123067186704, -1.003533581835382327, 18.50389795015985328 ) ) ;
#9107=VECTOR ( 'NONE', #10101, 1000.000000000000114 ) ;
#9108=CARTESIAN_POINT ( 'NONE',  ( -5.931734679891459194, 0.9039278060243389756, 5.263826032055957782 ) ) ;
#9111=CARTESIAN_POINT ( 'NONE',  ( 5.931828553037982843, -0.9033193133618682147, 11.76194324003145653 ) ) ;
#9112=CARTESIAN_POINT ( 'NONE',  ( 5.783198643800785632, 1.602922020054637908, 18.97377823943291730 ) ) ;
#9119=EDGE_CURVE ( 'NONE', #11432, #4730, #4557, .T. ) ;
#9123=CARTESIAN_POINT ( 'NONE',  ( -5.131373506000878493, 7.062729720843910819, 24.49999999999999289 ) ) ;
#9124=CARTESIAN_POINT ( 'NONE',  ( 1.354942165116848791E-13, 6.250000000000000888, 16.99999999999998579 ) ) ;
#9126=CARTESIAN_POINT ( 'NONE',  ( 5.616089948629776174, 2.743103014345448454, 23.99563030319847101 ) ) ;
#9127=FACE_OUTER_BOUND ( 'NONE', #4130, .T. ) ;
#9128=CARTESIAN_POINT ( 'NONE',  ( 2.817313151351108047, 5.579000502529472882, 5.000000000000004441 ) ) ;
#9129=CARTESIAN_POINT ( 'NONE',  ( -4.154121946520942465, -4.670585111242909981, 18.79887838423337953 ) ) ;
#9131=CARTESIAN_POINT ( 'NONE',  ( 4.005785023174460058, 4.467917056767396033, 4.200479458972858460 ) ) ;
#9134=FACE_BOUND ( 'NONE', #7370, .T. ) ;
#9135=CARTESIAN_POINT ( 'NONE',  ( -5.935543223013842962, 0.8771126767608004027, 18.13236078583909361 ) ) ;
#9140=EDGE_CURVE ( 'NONE', #3737, #9045, #12327, .T. ) ;
#9141=CARTESIAN_POINT ( 'NONE',  ( -0.6144377077727894987, -5.969178481556086879, 23.70033966857735663 ) ) ;
#9142=VERTEX_POINT ( 'NONE', #12807 ) ;
#9143=DIRECTION ( 'NONE',  ( -0.5877852522924685852, -0.8090169943749508930, 0.000000000000000000 ) ) ;
#9144=CARTESIAN_POINT ( 'NONE',  ( -0.9999171162589696182, -6.169494774098548184, 4.867223203306743073 ) ) ;
#9148=DIRECTION ( 'NONE',  ( 0.8090169943749506709, -0.5877852522924686962, 0.000000000000000000 ) ) ;
#9149=CARTESIAN_POINT ( 'NONE',  ( -5.329907877631355539, -2.755840666746254275, 5.261943240031468072 ) ) ;
#9151=CARTESIAN_POINT ( 'NONE',  ( 5.726049995854543440, -2.506679546901704470, 23.70045537531157365 ) ) ;
#9152=CARTESIAN_POINT ( 'NONE',  ( -5.770167736194727226, 2.404664418229086831, 4.126326713640078303 ) ) ;
#9153=CARTESIAN_POINT ( 'NONE',  ( -4.286401442266546624, -4.198423832313178394, 31.00000000000000000 ) ) ;
#9154=EDGE_LOOP ( 'NONE', ( #2171, #12753 ) ) ;
#9158=ORIENTED_EDGE ( 'NONE', *, *, #14246, .T. ) ;
#9161=LINE ( 'NONE', #10425, #5644 ) ;
#9164=CARTESIAN_POINT ( 'NONE',  ( 5.487097279078525958, -2.429065649168602015, 23.70047945897283270 ) ) ;
#9170=CARTESIAN_POINT ( 'NONE',  ( -0.7993401192311766490, 6.199366368793662652, 31.61483246936573011 ) ) ;
#9171=ORIENTED_EDGE ( 'NONE', *, *, #13177, .T. ) ;
#9172=ORIENTED_EDGE ( 'NONE', *, *, #2098, .T. ) ;
#9173=EDGE_LOOP ( 'NONE', ( #7503, #4835 ) ) ;
#9174=CARTESIAN_POINT ( 'NONE',  ( 3.882809187878950574, -4.899079348630037245, 12.47400098023328674 ) ) ;
#9175=CARTESIAN_POINT ( 'NONE',  ( -2.668367453516691690, -5.373994336898102020, 11.49999999999998224 ) ) ;
#9176=ORIENTED_EDGE ( 'NONE', *, *, #7457, .F. ) ;
#9179=CARTESIAN_POINT ( 'NONE',  ( 5.558508435838239059, -2.857531096718835428, 31.00000000000000000 ) ) ;
#9180=CARTESIAN_POINT ( 'NONE',  ( 2.030576276931546336E-13, -6.250000000000000888, 25.49999999999999645 ) ) ;
#9183=CARTESIAN_POINT ( 'NONE',  ( 5.931793676715101604, 0.9035324301688090198, 18.26239891805595050 ) ) ;
#9188=CARTESIAN_POINT ( 'NONE',  ( 3.883716939928966383, 4.898343590941268033, 18.97359571723300675 ) ) ;
#9192=CARTESIAN_POINT ( 'NONE',  ( 4.069800786343853893, -4.744882212776776242, 5.873819640450717472 ) ) ;
#9193=CARTESIAN_POINT ( 'NONE',  ( -5.558508435838188433, -2.857531096718932684, 5.000000000000004441 ) ) ;
#9194=CARTESIAN_POINT ( 'NONE',  ( -1.000049560716552044, 5.916071405810145123, 4.869677990115311772 ) ) ;
#9196=DIRECTION ( 'NONE',  ( -0.5877852522924685852, -0.8090169943749508930, 0.000000000000000000 ) ) ;
#9197=CARTESIAN_POINT ( 'NONE',  ( -0.8738239080078270549, -6.188820299975621886, 25.00355795710143170 ) ) ;
#9204=ADVANCED_FACE ( 'NONE', ( #5744 ), #11619, .F. ) ;
#9206=FACE_BOUND ( 'NONE', #14900, .T. ) ;
#9207=EDGE_CURVE ( 'NONE', #12866, #4157, #11773, .T. ) ;
#9208=B_SPLINE_CURVE_WITH_KNOTS ( 'NONE', 3,
 ( #6954, #11787, #3355, #888, #8223, #13058, #13138, #7030, #11858, #14324, #3431, #7109, #5913, #10761, #12341, #14412, #1362, #12103 ),
 .UNSPECIFIED., .F., .F.,
 ( 4, 2, 2, 2, 2, 2, 2, 2, 4 ),
 ( 0.003131486019301987257, 0.003522824630466693530, 0.003914163241631399802, 0.004305501852796106074, 0.004696840463960812347, 0.005088179075125518619, 0.005479517686290224891, 0.005870856297454931164, 0.006262194908619637436 ),
 .UNSPECIFIED. ) ;
#9209=CARTESIAN_POINT ( 'NONE',  ( -5.746996058422752185, 1.729015645941996304, 19.00007961174475568 ) ) ;
#9213=CARTESIAN_POINT ( 'NONE',  ( 3.882809187878850654, -4.899079348630117181, 25.47400098023329917 ) ) ;
#9214=LINE ( 'NONE', #768, #13350 ) ;
#9215=VERTEX_POINT ( 'NONE', #5589 ) ;
#9216=CARTESIAN_POINT ( 'NONE',  ( 7.180990026460803755, -3.384707322287205944, 24.49999999999999289 ) ) ;
#9219=ADVANCED_FACE ( 'NONE', ( #10436 ), #13121, .F. ) ;
#9220=DIRECTION ( 'NONE',  ( -0.3090169943749447867, -0.9510565162951544194, 0.000000000000000000 ) ) ;
#9226=CARTESIAN_POINT ( 'NONE',  ( 5.903596343266283242, 2.055998103990630099, 10.50004921015705150 ) ) ;
#9227=CARTESIAN_POINT ( 'NONE',  ( -5.984595133899197172, 1.806709459528603956, 4.000049210157070156 ) ) ;
#9228=LINE ( 'NONE', #3399, #13044 ) ;
#9229=ORIENTED_EDGE ( 'NONE', *, *, #15431, .F. ) ;
#9231=CARTESIAN_POINT ( 'NONE',  ( -4.435347140101058017, -4.403429997944488861, 11.63060690723496293 ) ) ;
#9242=CARTESIAN_POINT ( 'NONE',  ( -5.746996058422731757, -1.729015645942072688, 16.99992038825522656 ) ) ;
#9246=VERTEX_POINT ( 'NONE', #10585 ) ;
#9247=VERTEX_POINT ( 'NONE', #6940 ) ;
#9250=CARTESIAN_POINT ( 'NONE',  ( 3.419318284370132410, -4.932111238568221978, 25.49992002356261622 ) ) ;
#9251=CARTESIAN_POINT ( 'NONE',  ( 2.030576276931546336E-13, -6.000000000000000888, 25.49999999999999645 ) ) ;
#9255=CARTESIAN_POINT ( 'NONE',  ( -5.329907877631348434, -2.755840666746270262, 31.26194324003147429 ) ) ;
#9256=CARTESIAN_POINT ( 'NONE',  ( -3.255128505894222535, -5.336774832660773349, 4.126199447526042619 ) ) ;
#9262=EDGE_CURVE ( 'NONE', #13656, #13850, #14987, .T. ) ;
#9263=CARTESIAN_POINT ( 'NONE',  ( -5.935543223013848291, -0.8771126767607491104, 4.867639214160894845 ) ) ;
#9265=DIRECTION ( 'NONE',  ( 0.8090169943749506709, -0.5877852522924686962, 0.000000000000000000 ) ) ;
#9266=EDGE_LOOP ( 'NONE', ( #5593, #5402, #9520, #12569 ) ) ;
#9268=EDGE_LOOP ( 'NONE', ( #1919, #11079 ) ) ;
#9269=CARTESIAN_POINT ( 'NONE',  ( 6.780834061396424457E-14, 6.250000000000000888, 10.49999999999998224 ) ) ;
#9271=CARTESIAN_POINT ( 'NONE',  ( 6.176542424588121527, -0.9554180641285238140, 31.00000000000000000 ) ) ;
#9272=CARTESIAN_POINT ( 'NONE',  ( 5.770331821586450971, 2.404225004693483658, 23.62619944752604439 ) ) ;
#9275=FACE_BOUND ( 'NONE', #4094, .T. ) ;
#9278=CARTESIAN_POINT ( 'NONE',  ( -3.883588957979317247, -4.898466244118881541, 25.47377282875268278 ) ) ;
#9282=EDGE_CURVE ( 'NONE', #3268, #14489, #10810, .T. ) ;
#9284=FACE_BOUND ( 'NONE', #6533, .T. ) ;
#9285=CARTESIAN_POINT ( 'NONE',  ( -5.317509234263907203, 2.779225709351096363, 18.13061695532137207 ) ) ;
#9289=FACE_OUTER_BOUND ( 'NONE', #12966, .T. ) ;
#9291=CARTESIAN_POINT ( 'NONE',  ( -5.558508435838167117, 2.857531096718976205, 18.13060690723497004 ) ) ;
#9298=FACE_BOUND ( 'NONE', #4056, .T. ) ;
#9300=CARTESIAN_POINT ( 'NONE',  ( 0.2624013748573350013, 5.995472630654520074, 30.02628559691082444 ) ) ;
#9301=AXIS2_PLACEMENT_3D ( 'NONE', #2113, #3314, #5711 ) ;
#9307=EDGE_CURVE ( 'NONE', #7142, #15044, #5100, .T. ) ;
#9310=CARTESIAN_POINT ( 'NONE',  ( 4.069800786343690469, 4.744882212776914798, 17.12618035954927720 ) ) ;
#9312=CARTESIAN_POINT ( 'NONE',  ( -4.435347140101010055, -4.403429997944535046, 5.000000000000004441 ) ) ;
#9314=CARTESIAN_POINT ( 'NONE',  ( 4.142173849413770981, -4.341773579105383085, 10.88480617551147134 ) ) ;
#9316=CARTESIAN_POINT ( 'NONE',  ( 5.317509234263932072, 2.779225709351047957, 5.000000000000004441 ) ) ;
#9317=CARTESIAN_POINT ( 'NONE',  ( -5.375605342016431365, -2.665598297262440131, 17.49687951097621763 ) ) ;
#9318=CARTESIAN_POINT ( 'NONE',  ( 5.903230462362958342, 1.077253041748864604, 12.11442521571935949 ) ) ;
#9320=ORIENTED_EDGE ( 'NONE', *, *, #9950, .T. ) ;
#9327=CARTESIAN_POINT ( 'NONE',  ( -5.375763363753427448, -2.665284979407579691, 31.50389795015983552 ) ) ;
#9335=CARTESIAN_POINT ( 'NONE',  ( -5.866923913994641637, -1.260079467906541684, 4.200479458972859348 ) ) ;
#9339=VERTEX_POINT ( 'NONE', #14803 ) ;
#9343=CARTESIAN_POINT ( 'NONE',  ( 4.344265632482186668, -4.493596842504861577, 5.504259495030091820 ) ) ;
#9344=CARTESIAN_POINT ( 'NONE',  ( 4.286401442266496886, -4.198423832313229020, 17.86760611998365178 ) ) ;
#9345=CARTESIAN_POINT ( 'NONE',  ( 6.172651332693114057, 0.9815532474592564283, 24.23809786915987985 ) ) ;
#9348=CARTESIAN_POINT ( 'NONE',  ( -5.746837578675986435, 1.729433780394314502, 17.00004946353775992 ) ) ;
#9349=FACE_BOUND ( 'NONE', #14587, .T. ) ;
#9352=CARTESIAN_POINT ( 'NONE',  ( -2.841519077896259127, -5.566940434249956660, 24.76379616840806008 ) ) ;
#9353=VECTOR ( 'NONE', #4729, 1000.000000000000114 ) ;
#9357=CARTESIAN_POINT ( 'NONE',  ( -6.020865209844600052, 1.681180471732123483, 12.47400098023328674 ) ) ;
#9359=FACE_BOUND ( 'NONE', #8415, .T. ) ;
#9363=CARTESIAN_POINT ( 'NONE',  ( 3.566234721237978356, -5.134387337253871308, 25.49991741810288559 ) ) ;
#9365=CARTESIAN_POINT ( 'NONE',  ( -0.9737778612003452627, -5.920671847850547564, 24.23736375884649519 ) ) ;
#9368=DIRECTION ( 'NONE',  ( 0.5877852522924802425, -0.8090169943749422332, 0.000000000000000000 ) ) ;
#9373=CARTESIAN_POINT ( 'NONE',  ( 6.106056299406772858, 1.336851112280557974, 25.29887838423337953 ) ) ;
#9374=CYLINDRICAL_SURFACE ( 'NONE', #4796, 1.000000000000000222 ) ;
#9375=CARTESIAN_POINT ( 'NONE',  ( -4.435347140101074004, 4.403429997944469321, 5.000000000000004441 ) ) ;
#9377=FACE_BOUND ( 'NONE', #10969, .T. ) ;
#9379=CARTESIAN_POINT ( 'NONE',  ( -4.196038884587139250, -4.289036423669302600, 30.49610204984016448 ) ) ;
#9380=ORIENTED_EDGE ( 'NONE', *, *, #9594, .T. ) ;
#9382=CARTESIAN_POINT ( 'NONE',  ( 2.782156709077397760, 5.316215864844059169, 30.49687951097622118 ) ) ;
#9384=FACE_OUTER_BOUND ( 'NONE', #4832, .T. ) ;
#9387=CARTESIAN_POINT ( 'NONE',  ( 4.435347140100915908, 4.403429997944633634, 17.86765874365829276 ) ) ;
#9395=CARTESIAN_POINT ( 'NONE',  ( 5.915755444410801367, 1.003187219519861895, 12.00312048902374862 ) ) ;
#9396=EDGE_CURVE ( 'NONE', #7094, #10183, #4358, .T. ) ;
#9399=ORIENTED_EDGE ( 'NONE', *, *, #14160, .F. ) ;
#9400=ORIENTED_EDGE ( 'NONE', *, *, #13572, .F. ) ;
#9402=CARTESIAN_POINT ( 'NONE',  ( -3.735642931251092591, 4.696778275484423837, 12.47408052783099031 ) ) ;
#9406=CARTESIAN_POINT ( 'NONE',  ( -1.000049560716352426, 5.916071405810178874, 24.36967799011533131 ) ) ;
#9407=DIRECTION ( 'NONE',  ( 0.000000000000000000, 1.000000000000000000, 0.000000000000000000 ) ) ;
#9410=B_SPLINE_CURVE_WITH_KNOTS ( 'NONE', 3,
 ( #2501, #1142, #11010, #6172, #2417, #108, #15633, #5929, #7043, #986, #3687, #7357, #4976, #7204, #7283, #14428, #9753, #3532 ),
 .UNSPECIFIED., .F., .F.,
 ( 4, 2, 2, 2, 2, 2, 2, 2, 4 ),
 ( 0.003131918686235973890, 0.003523310662250265894, 0.003914702638264557465, 0.004306094614278849902, 0.004697486590293141473, 0.005088878566307433043, 0.005480270542321723747, 0.005871662518336014450, 0.006263054494350305153 ),
 .UNSPECIFIED. ) ;
#9417=CARTESIAN_POINT ( 'NONE',  ( 4.435347140100914132, 4.403429997944631857, 17.99999999999998934 ) ) ;
#9418=ORIENTED_EDGE ( 'NONE', *, *, #15326, .F. ) ;
#9419=CARTESIAN_POINT ( 'NONE',  ( -5.409007216690624453, 2.598315788643851043, 25.11442521571937547 ) ) ;
#9421=ORIENTED_EDGE ( 'NONE', *, *, #4590, .F. ) ;
#9422=CARTESIAN_POINT ( 'NONE',  ( 0.9999171162589906015, 6.169494774098545520, 30.86722320330672531 ) ) ;
#9424=CARTESIAN_POINT ( 'NONE',  ( -0.1306497350717320538, 6.000000000000001776, 4.000000000000004441 ) ) ;
#9425=ORIENTED_EDGE ( 'NONE', *, *, #1450, .T. ) ;
#9429=CARTESIAN_POINT ( 'NONE',  ( 4.286401442266387640, 4.198423832313340043, 24.63239388001634111 ) ) ;
#9431=CARTESIAN_POINT ( 'NONE',  ( -4.070863287254169016, -4.743975846881727243, 18.87305891554299819 ) ) ;
#9433=CARTESIAN_POINT ( 'NONE',  ( -4.344762547369802164, -4.493114738039127865, 25.00308643866044633 ) ) ;
#9438=CARTESIAN_POINT ( 'NONE',  ( 4.267936573529218514, 4.217499624512227818, 31.26229037835931379 ) ) ;
#9444=CYLINDRICAL_SURFACE ( 'NONE', #3439, 1.000000000000000000 ) ;
#9453=LINE ( 'NONE', #1093, #5012 ) ;
#9455=CARTESIAN_POINT ( 'NONE',  ( 5.570760634536790157, 2.834026536768273541, 11.23774718278288276 ) ) ;
#9459=ORIENTED_EDGE ( 'NONE', *, *, #7284, .F. ) ;
#9463=CARTESIAN_POINT ( 'NONE',  ( -1.000049560716488761, 5.916071405810155781, 11.36967799011531710 ) ) ;
#9465=CARTESIAN_POINT ( 'NONE',  ( -4.143041610105282935, -4.340967609747059086, 4.386022610569177971 ) ) ;
#9467=CYLINDRICAL_SURFACE ( 'NONE', #11627, 1.000000000000000666 ) ;
#9468=CARTESIAN_POINT ( 'NONE',  ( 5.665824935993625466, 1.978765057080873913, 17.00004946353775992 ) ) ;
#9470=CARTESIAN_POINT ( 'NONE',  ( 2.782468714962263334, 5.316055268221493435, 18.50389795015982841 ) ) ;
#9472=CARTESIAN_POINT ( 'NONE',  ( -5.903061651806607024, -2.057626436184781582, 4.000082581897114409 ) ) ;
#9477=DIRECTION ( 'NONE',  ( 0.8090169943749506709, -0.5877852522924689183, 0.000000000000000000 ) ) ;
#9481=CARTESIAN_POINT ( 'NONE',  ( 4.435347140100995844, 4.403429997944549257, 31.00000000000000000 ) ) ;
#9482=CARTESIAN_POINT ( 'NONE',  ( 7.490007020835728113, -2.433650805992114918, 17.99999999999998934 ) ) ;
#9487=CARTESIAN_POINT ( 'NONE',  ( 0.1323933160975658274, -6.000000000000000000, 6.000000000000003553 ) ) ;
#9488=CARTESIAN_POINT ( 'NONE',  ( -2.817313151351109379, -5.579000502529473771, 4.867625892836954904 ) ) ;
#9491=LINE ( 'NONE', #970, #2868 ) ;
#9497=EDGE_LOOP ( 'NONE', ( #5966, #9624 ) ) ;
#9499=CARTESIAN_POINT ( 'NONE',  ( 6.000000000000000888, 7.347880794884120722E-16, 53.67766952966368876 ) ) ;
#9500=ORIENTED_EDGE ( 'NONE', *, *, #4773, .F. ) ;
#9502=CARTESIAN_POINT ( 'NONE',  ( 0.5030929395820508132, 6.230885867001143552, 30.12600319116549485 ) ) ;
#9503=EDGE_CURVE ( 'NONE', #7387, #2947, #940, .T. ) ;
#9504=CARTESIAN_POINT ( 'NONE',  ( 2.668367453516584220, -5.373994336898154422, 17.99999999999998934 ) ) ;
#9505=CARTESIAN_POINT ( 'NONE',  ( -4.196288036172508562, -4.288789315524776491, 25.00312048902377882 ) ) ;
#9507=ADVANCED_FACE ( 'NONE', ( #12715 ), #5176, .F. ) ;
#9508=CARTESIAN_POINT ( 'NONE',  ( -6.081509788407757355, 1.446521464462645401, 31.87381964045071214 ) ) ;
#9509=CARTESIAN_POINT ( 'NONE',  ( 4.286401442266388528, 4.198423832313340043, 24.49999999999999289 ) ) ;
#9510=LINE ( 'NONE', #6969, #12995 ) ;
#9511=CARTESIAN_POINT ( 'NONE',  ( -2.931156713028535865, 5.520271803279187317, 12.00436969680153076 ) ) ;
#9513=CARTESIAN_POINT ( 'NONE',  ( -2.997753866155913549, -5.484939622623791422, 25.11560192892921606 ) ) ;
#9514=EDGE_CURVE ( 'NONE', #13977, #2787, #13906, .T. ) ;
#9518=CARTESIAN_POINT ( 'NONE',  ( 4.005998022989950336, 4.467726698309270716, 31.79931806258174021 ) ) ;
#9520=ORIENTED_EDGE ( 'NONE', *, *, #8312, .T. ) ;
#9521=CARTESIAN_POINT ( 'NONE',  ( -3.107583187530425839, 5.133966411712686195, 4.126193172852896218 ) ) ;
#9522=CYLINDRICAL_SURFACE ( 'NONE', #14272, 1.000000000000000666 ) ;
#9523=DIRECTION ( 'NONE',  ( -0.9510565162951544194, 0.3090169943749447312, 0.000000000000000000 ) ) ;
#9526=DIRECTION ( 'NONE',  ( -0.9510565162951545304, 0.3090169943749447867, 0.000000000000000000 ) ) ;
#9528=CARTESIAN_POINT ( 'NONE',  ( -5.903057025253903412, -1.078199533779516495, 30.38438267301394191 ) ) ;
#9529=VECTOR ( 'NONE', #15365, 1000.000000000000114 ) ;
#9532=CARTESIAN_POINT ( 'NONE',  ( 6.155973317223311092, 1.081218830693581268, 25.00308643866044989 ) ) ;
#9534=DIRECTION ( 'NONE',  ( 0.5877852522924802425, -0.8090169943749422332, 0.000000000000000000 ) ) ;
#9536=CARTESIAN_POINT ( 'NONE',  ( 5.616089948629710449, 2.743103014345580348, 10.99563030319847279 ) ) ;
#9538=CARTESIAN_POINT ( 'NONE',  ( 5.725930890718329280, 2.506952462184043995, 17.20066851092422411 ) ) ;
#9542=CARTESIAN_POINT ( 'NONE',  ( 5.843075991566612615, 1.368655265450926528, 23.62635295315577011 ) ) ;
#9544=ORIENTED_EDGE ( 'NONE', *, *, #582, .T. ) ;
#9545=CARTESIAN_POINT ( 'NONE',  ( -2.849269941561920927, -5.281123252784068356, 4.384806175511482884 ) ) ;
#9546=B_SPLINE_CURVE_WITH_KNOTS ( 'NONE', 3,
 ( #12606, #1704, #6580, #10000, #13638, #8731, #2673, #11415, #516, #7525, #12371, #1469, #7604, #12452, #1552, #5228, #12990, #8076 ),
 .UNSPECIFIED., .F., .F.,
 ( 4, 2, 2, 2, 2, 2, 2, 2, 4 ),
 ( 0.000000000000000000, 0.0003914357524127466724, 0.0007828715048254933449, 0.001174307257238240126, 0.001565743009650986690, 0.001957178762063733254, 0.002348614514476480251, 0.002740050266889226815, 0.003131486019301973379 ),
 .UNSPECIFIED. ) ;
#9547=CARTESIAN_POINT ( 'NONE',  ( 5.409274167810653289, -2.597759609440645878, 5.615193824488510010 ) ) ;
#9548=ADVANCED_FACE ( 'NONE', ( #1581 ), #3966, .F. ) ;
#9550=DIRECTION ( 'NONE',  ( 0.5877852522924802425, -0.8090169943749422332, 0.000000000000000000 ) ) ;
#9552=CARTESIAN_POINT ( 'NONE',  ( 2.668367453516506949, 5.373994336898193502, 18.13064961348854709 ) ) ;
#9554=CARTESIAN_POINT ( 'NONE',  ( 4.286401442266544848, -4.198423832313181059, 11.49999999999998224 ) ) ;
#9556=CARTESIAN_POINT ( 'NONE',  ( 1.000049271338508516, -6.169473353325548359, 30.86969612704550414 ) ) ;
#9557=CARTESIAN_POINT ( 'NONE',  ( -5.726307184802641004, 2.506131700382491445, 10.69973484982323519 ) ) ;
#9558=CARTESIAN_POINT ( 'NONE',  ( 1.354942164306246880E-13, -6.000000000000000888, 16.99999999999998579 ) ) ;
#9562=CARTESIAN_POINT ( 'NONE',  ( 6.176542424588106428, 0.9554180641286317277, 4.869360672457872852 ) ) ;
#9563=ORIENTED_EDGE ( 'NONE', *, *, #1067, .T. ) ;
#9565=CARTESIAN_POINT ( 'NONE',  ( -5.903119516422473012, -1.077859910107510588, 31.61519382448851090 ) ) ;
#9569=SHAPE_REPRESENTATION ( 'strain limiting mesh layer', ( #14201 ), #10667 ) ;
#9570=CARTESIAN_POINT ( 'NONE',  ( -5.558508435838166228, 2.857531096718976649, 17.99999999999998934 ) ) ;
#9572=CARTESIAN_POINT ( 'NONE',  ( 3.159612573729317919, -5.393342049074581368, 4.199734849823245852 ) ) ;
#9578=FACE_OUTER_BOUND ( 'NONE', #3272, .T. ) ;
#9580=ORIENTED_EDGE ( 'NONE', *, *, #8261, .F. ) ;
#9581=CARTESIAN_POINT ( 'NONE',  ( 0.7995524673975824559, 6.199337389817267230, 31.61453679452459653 ) ) ;
#9582=CARTESIAN_POINT ( 'NONE',  ( -4.435347140101154828, -4.403429997944389385, 24.49999999999999289 ) ) ;
#9583=B_SPLINE_CURVE_WITH_KNOTS ( 'NONE', 3,
 ( #3093, #620, #11597, #858, #3168, #11519, #15190, #12864, #9227, #4367, #2124, #9152, #12786, #11826, #5725, #4288, #2048, #13905 ),
 .UNSPECIFIED., .F., .F.,
 ( 4, 2, 2, 2, 2, 2, 2, 2, 4 ),
 ( 0.000000000000000000, 0.0003914357524127480819, 0.0007828715048254961638, 0.001174307257238244246, 0.001565743009650992328, 0.001957178762063741060, 0.002348614514476489792, 0.002740050266889238525, 0.003131486019301987257 ),
 .UNSPECIFIED. ) ;
#9584=CARTESIAN_POINT ( 'NONE',  ( -3.107583187530525315, -5.133966411712624023, 25.37380682714709579 ) ) ;
#9585=CARTESIAN_POINT ( 'NONE',  ( 4.435347140101025154, -4.403429997944519059, 11.49999999999998224 ) ) ;
#9586=CARTESIAN_POINT ( 'NONE',  ( 4.195842658231335065, 4.289229542213299773, 25.00439760644211518 ) ) ;
#9588=CARTESIAN_POINT ( 'NONE',  ( -3.567624405365362072, 5.133384272590696185, 12.49995078984291830 ) ) ;
#9589=CARTESIAN_POINT ( 'NONE',  ( 5.329945432499583191, 2.755769831645226375, 30.73770962164068266 ) ) ;
#9590=DIRECTION ( 'NONE',  ( 0.8090169943749506709, -0.5877852522924686962, 0.000000000000000000 ) ) ;
#9594=EDGE_CURVE ( 'NONE', #5121, #12426, #9228, .T. ) ;
#9596=PRODUCT_DEFINITION_FORMATION_WITH_SPECIFIED_SOURCE ( 'ANY', '', #2311, .NOT_KNOWN. ) ;
#9597=CARTESIAN_POINT ( 'NONE',  ( 5.616116467183692507, -2.743044348085474038, 17.49574050496990907 ) ) ;
#9599=AXIS2_PLACEMENT_3D ( 'NONE', #6411, #14512, #11088 ) ;
#9601=B_SPLINE_CURVE_WITH_KNOTS ( 'NONE', 3,
 ( #11477, #505, #7825, #8882, #7747, #6416, #4324, #13714, #2822, #6568, #12593, #581, #7903, #7670, #5450, #10296, #5374, #12518 ),
 .UNSPECIFIED., .F., .F.,
 ( 4, 2, 2, 2, 2, 2, 2, 2, 4 ),
 ( 0.003131918686235976926, 0.003523310662250266762, 0.003914702638264556597, 0.004306094614278846433, 0.004697486590293136269, 0.005088878566307426105, 0.005480270542321715940, 0.005871662518336004041, 0.006263054494350293010 ),
 .UNSPECIFIED. ) ;
#9602=EDGE_LOOP ( 'NONE', ( #7257, #8889, #13130, #6083 ) ) ;
#9603=LINE ( 'NONE', #15570, #3510 ) ;
#9604=CARTESIAN_POINT ( 'NONE',  ( 1.000049560716623098, -5.916071405810133577, 11.36967799011532598 ) ) ;
#9605=B_SPLINE_CURVE_WITH_KNOTS ( 'NONE', 3,
 ( #12604, #1389, #2671, #15008, #434, #1550, #11102, #10229, #15081, #8656, #204, #5308, #9918, #12528, #7523, #12369, #4098, #13798 ),
 .UNSPECIFIED., .F., .F.,
 ( 4, 2, 2, 2, 2, 2, 2, 2, 4 ),
 ( 0.000000000000000000, 0.0003914357524127471603, 0.0007828715048254943206, 0.001174307257238241644, 0.001565743009650988641, 0.001957178762063735422, 0.002348614514476481552, 0.002740050266889228116, 0.003131486019301974680 ),
 .UNSPECIFIED. ) ;
#9606=CARTESIAN_POINT ( 'NONE',  ( 2.668367453516610865, 5.373994336898140212, 31.00000000000000000 ) ) ;
#9615=CARTESIAN_POINT ( 'NONE',  ( -0.8738239080080079102, -6.188820299975598793, 31.50355795710144946 ) ) ;
#9617=CARTESIAN_POINT ( 'NONE',  ( -3.882673863916280332, 4.899192824800945978, 5.974085423341712442 ) ) ;
#9619=B_SPLINE_CURVE_WITH_KNOTS ( 'NONE', 3,
 ( #5636, #9291, #3233, #8100, #6911, #4511, #11746, #5713, #4595, #10557, #14207, #8177, #13015, #2115, #921, #15499, #3387, #14360 ),
 .UNSPECIFIED., .F., .F.,
 ( 4, 2, 2, 2, 2, 2, 2, 2, 4 ),
 ( 0.003131486019301970777, 0.003522824630466679218, 0.003914163241631387659, 0.004305501852796096533, 0.004696840463960804540, 0.005088179075125513415, 0.005479517686290222289, 0.005870856297454931164, 0.006262194908619639171 ),
 .UNSPECIFIED. ) ;
#9624=ORIENTED_EDGE ( 'NONE', *, *, #5981, .F. ) ;
#9638=CARTESIAN_POINT ( 'NONE',  ( 5.409274167810663947, -2.597759609440622341, 31.61519382448851090 ) ) ;
#9640=CARTESIAN_POINT ( 'NONE',  ( -5.984595133899179409, 1.806709459528658135, 10.50004921015705150 ) ) ;
#9642=ORIENTED_EDGE ( 'NONE', *, *, #12036, .F. ) ;
#9643=EDGE_CURVE ( 'NONE', #7578, #9215, #2470, .T. ) ;
#9644=VERTEX_POINT ( 'NONE', #4606 ) ;
#9646=ORIENTED_EDGE ( 'NONE', *, *, #8965, .F. ) ;
#9647=CARTESIAN_POINT ( 'NONE',  ( -2.849269941562057262, 5.281123252783995525, 12.11519382448850557 ) ) ;
#9652=CARTESIAN_POINT ( 'NONE',  ( 6.176542424588109093, 0.9554180641286111886, 31.00000000000000000 ) ) ;
#9655=CARTESIAN_POINT ( 'NONE',  ( -2.668367453516691690, -5.373994336898102020, 11.49999999999998224 ) ) ;
#9659=LINE ( 'NONE', #15619, #7583 ) ;
#9664=CARTESIAN_POINT ( 'NONE',  ( 4.435347140100961205, 4.403429997944583008, 11.49999999999998224 ) ) ;
#9667=CARTESIAN_POINT ( 'NONE',  ( -5.725684683139557585, 2.507514573674882286, 25.29887838423338309 ) ) ;
#9670=CARTESIAN_POINT ( 'NONE',  ( 0.1323736289504360564, -6.250000000000000000, 6.000000000000007105 ) ) ;
#9672=CARTESIAN_POINT ( 'NONE',  ( -5.558508435838220407, 2.857531096718872732, 31.13060690723498780 ) ) ;
#9674=CYLINDRICAL_SURFACE ( 'NONE', #9599, 1.000000000000000666 ) ;
#9677=CARTESIAN_POINT ( 'NONE',  ( 5.915699123067156506, 1.003533581835566846, 30.49610204984016448 ) ) ;
#9678=CARTESIAN_POINT ( 'NONE',  ( 0.8002302970948492744, -5.947135855825840700, 23.88601773212297630 ) ) ;
#9682=CARTESIAN_POINT ( 'NONE',  ( 3.421280866381124497, 4.930711975950923254, 32.00004932073312602 ) ) ;
#9683=CARTESIAN_POINT ( 'NONE',  ( 5.487097279078418488, 2.429065649168846708, 31.79952054102715309 ) ) ;
#9684=ORIENTED_EDGE ( 'NONE', *, *, #11916, .F. ) ;
#9686=CARTESIAN_POINT ( 'NONE',  ( -1.000079958708067318, -5.916066267613712348, 11.63152738882033965 ) ) ;
#9687=CARTESIAN_POINT ( 'NONE',  ( -4.286401442266737583, 4.198423832312984771, 24.49999999999999289 ) ) ;
#9693=EDGE_CURVE ( 'NONE', #6042, #3644, #2890, .T. ) ;
#9696=CARTESIAN_POINT ( 'NONE',  ( 5.783198643800774086, -1.602922020054686758, 4.026221760567070262 ) ) ;
#9698=CARTESIAN_POINT ( 'NONE',  ( -5.903061651806607912, 2.057626436184776697, 12.49991741810287138 ) ) ;
#9703=CARTESIAN_POINT ( 'NONE',  ( 5.570760634536824796, 2.834026536768204263, 17.73774718278285434 ) ) ;
#9707=AXIS2_PLACEMENT_3D ( 'NONE', #3551, #8421, #12141 ) ;
#9709=CARTESIAN_POINT ( 'NONE',  ( -2.817313151351169775, -5.579000502529442684, 11.63234125634165927 ) ) ;
#9710=EDGE_LOOP ( 'NONE', ( #7991, #10666 ) ) ;
#9715=DIRECTION ( 'NONE',  ( 0.5877852522924802425, -0.8090169943749422332, 0.000000000000000000 ) ) ;
#9717=CARTESIAN_POINT ( 'NONE',  ( 4.286401442266498663, -4.198423832313231685, 18.13236078583909361 ) ) ;
#9721=CARTESIAN_POINT ( 'NONE',  ( 5.317509234263978257, -2.779225709350955587, 31.13239388001635177 ) ) ;
#9723=CARTESIAN_POINT ( 'NONE',  ( -0.1323408341373540076, -6.250000000000002665, 18.99999999999998934 ) ) ;
#9724=CARTESIAN_POINT ( 'NONE',  ( 5.935543223013847403, 0.8771126767607486663, 4.869350386511450246 ) ) ;
#9725=CARTESIAN_POINT ( 'NONE',  ( 5.531757352715589882, 2.326874507723354579, 12.37380682714709401 ) ) ;
#9728=ORIENTED_EDGE ( 'NONE', *, *, #13196, .F. ) ;
#9730=CARTESIAN_POINT ( 'NONE',  ( -5.408775798201078899, -2.598833957129834005, 25.11397738943081848 ) ) ;
#9733=CARTESIAN_POINT ( 'NONE',  ( 0.6144377077729795689, 5.969178481556069116, 4.200339668577359298 ) ) ;
#9734=CARTESIAN_POINT ( 'NONE',  ( 5.616116467183609018, 2.743044348085646789, 31.50425949503011225 ) ) ;
#9736=EDGE_CURVE ( 'NONE', #1036, #1161, #7213, .T. ) ;
#9739=CARTESIAN_POINT ( 'NONE',  ( -5.984595133899110131, -1.806709459528883288, 25.49995078984292363 ) ) ;
#9741=AXIS2_PLACEMENT_3D ( 'NONE', #4479, #1050, #5603 ) ;
#9742=B_SPLINE_CURVE_WITH_KNOTS ( 'NONE', 3,
 ( #619, #12713, #1812, #5412, #10259, #11289, #386, #6684, #5256, #10103, #14957, #8918, #13752, #2860, #7708, #15662, #5958, #2047 ),
 .UNSPECIFIED., .F., .F.,
 ( 4, 2, 2, 2, 2, 2, 2, 2, 4 ),
 ( 0.003131918686235977793, 0.003523310662250268063, 0.003914702638264558332, 0.004306094614278849035, 0.004697486590293138004, 0.005088878566307427839, 0.005480270542321717675, 0.005871662518336007511, 0.006263054494350296479 ),
 .UNSPECIFIED. ) ;
#9747=EDGE_LOOP ( 'NONE', ( #12253, #5437 ) ) ;
#9750=CARTESIAN_POINT ( 'NONE',  ( -5.558508435838179551, -2.857531096718950447, 30.86939309276501220 ) ) ;
#9751=FACE_OUTER_BOUND ( 'NONE', #15213, .T. ) ;
#9753=CARTESIAN_POINT ( 'NONE',  ( 4.286401442266547512, -4.198423832313182835, 11.63236078583908473 ) ) ;
#9754=CARTESIAN_POINT ( 'NONE',  ( 4.290381260516203277, -4.545736887716273600, 23.88482219624157210 ) ) ;
#9756=EDGE_CURVE ( 'NONE', #1036, #4730, #2531, .T. ) ;
#9758=CARTESIAN_POINT ( 'NONE',  ( -5.570820891630690497, -2.833901239560547403, 24.23763026556123279 ) ) ;
#9759=CARTESIAN_POINT ( 'NONE',  ( -4.435347140101107755, -4.403429997944436458, 17.99999999999998934 ) ) ;
#9764=CARTESIAN_POINT ( 'NONE',  ( -5.770167736194645514, -2.404664418229290224, 18.87367328635991726 ) ) ;
#9766=CARTESIAN_POINT ( 'NONE',  ( 5.843318061569038768, 1.367618216965670541, 31.87303779027051576 ) ) ;
#9768=DIRECTION ( 'NONE',  ( 0.8090169943749421222, 0.5877852522924802425, 0.000000000000000000 ) ) ;
#9769=CARTESIAN_POINT ( 'NONE',  ( 0.5044069930203958219, -5.979990686694987900, 12.37335743227902718 ) ) ;
#9772=DIRECTION ( 'NONE',  ( -0.3090169943749446202, -0.9510565162951544194, 0.000000000000000000 ) ) ;
#9773=LINE ( 'NONE', #212, #13513 ) ;
#9781=CARTESIAN_POINT ( 'NONE',  ( 5.616089948629818807, -2.743103014345361856, 25.00436969680152544 ) ) ;
#9782=ORIENTED_EDGE ( 'NONE', *, *, #10649, .F. ) ;
#9789=DIRECTION ( 'NONE',  ( -1.000000000000000000, 0.000000000000000000, 0.000000000000000000 ) ) ;
#9791=CARTESIAN_POINT ( 'NONE',  ( -0.9737725088281561359, -6.173885267451830750, 11.23735758726563994 ) ) ;
#9792=CARTESIAN_POINT ( 'NONE',  ( -7.799024015210622274, -1.482594289697344969, 17.99999999999998934 ) ) ;
#9794=CARTESIAN_POINT ( 'NONE',  ( -2.817313151351311884, 5.579000502529370742, 17.99999999999998934 ) ) ;
#9795=CARTESIAN_POINT ( 'NONE',  ( -6.176542424588072677, -0.9554180641288341214, 24.49999999999999289 ) ) ;
#9796=CARTESIAN_POINT ( 'NONE',  ( -2.931212650151679533, 5.520239928492807202, 30.49574050496989130 ) ) ;
#9797=CARTESIAN_POINT ( 'NONE',  ( -5.615973259022320363, 2.743340227996172942, 10.99610786875028801 ) ) ;
#9798=CARTESIAN_POINT ( 'NONE',  ( 2.848727059635853376, 5.281416301279955761, 23.88557478428062453 ) ) ;
#9800=ORIENTED_EDGE ( 'NONE', *, *, #9036, .T. ) ;
#9801=EDGE_CURVE ( 'NONE', #13214, #3990, #14617, .T. ) ;
#9802=VERTEX_POINT ( 'NONE', #13499 ) ;
#9808=AXIS2_PLACEMENT_3D ( 'NONE', #853, #5638, #6839 ) ;
#9815=CARTESIAN_POINT ( 'NONE',  ( 3.736691294293439825, 4.695920479336362696, 5.973585954366940065 ) ) ;
#9817=CARTESIAN_POINT ( 'NONE',  ( 2.930922878467578929, -5.520395124723519231, 4.496107868750327974 ) ) ;
#9819=CARTESIAN_POINT ( 'NONE',  ( 5.571002711501371607, 2.833546409886354311, 5.263796168408044096 ) ) ;
#9820=ORIENTED_EDGE ( 'NONE', *, *, #4528, .F. ) ;
#9822=ORIENTED_EDGE ( 'NONE', *, *, #10472, .T. ) ;
#9823=CARTESIAN_POINT ( 'NONE',  ( 5.409423237179028732, -2.597448116730994627, 30.38438267301393836 ) ) ;
#9825=CARTESIAN_POINT ( 'NONE',  ( 1.000082492230716769, 6.169467968613709274, 5.131525381053923418 ) ) ;
#9826=DIRECTION ( 'NONE',  ( 0.9510565162951499785, 0.3090169943749582204, 0.000000000000000000 ) ) ;
#9827=B_SPLINE_CURVE_WITH_KNOTS ( 'NONE', 3,
 ( #12273, #3912, #13618, #12351, #3760, #6482, #3838, #12507, #10134, #11162, #8711, #8788, #2730, #9823, #7506, #262, #1445, #1373 ),
 .UNSPECIFIED., .F., .F.,
 ( 4, 2, 2, 2, 2, 2, 2, 2, 4 ),
 ( 0.003131918686235979528, 0.003523310662250269364, 0.003914702638264559199, 0.004306094614278849035, 0.004697486590293139738, 0.005088878566307429574, 0.005480270542321720277, 0.005871662518336010980, 0.006263054494350301683 ),
 .UNSPECIFIED. ) ;
#9829=LINE ( 'NONE', #11963, #8707 ) ;
#9830=CARTESIAN_POINT ( 'NONE',  ( -6.081509788407761796, 1.446521464462625639, 5.873819640450719248 ) ) ;
#9831=CARTESIAN_POINT ( 'NONE',  ( 0.5044069930205320462, -5.979990686694976354, 25.37335743227903251 ) ) ;
#9837=EDGE_CURVE ( 'NONE', #10924, #4625, #8166, .T. ) ;
#9839=CARTESIAN_POINT ( 'NONE',  ( -5.984595133899159869, 1.806709459528722528, 17.00004921015705861 ) ) ;
#9840=CARTESIAN_POINT ( 'NONE',  ( -0.8730424326980312788, -5.936362132114472168, 10.99500690218562937 ) ) ;
#9842=CARTESIAN_POINT ( 'NONE',  ( 2.817313151351171552, -5.579000502529439132, 31.13060690723500201 ) ) ;
#9845=CARTESIAN_POINT ( 'NONE',  ( -2.668367453516768517, 5.373994336898062052, 11.49999999999998224 ) ) ;
#9847=CYLINDRICAL_SURFACE ( 'NONE', #4900, 1.000000000000000666 ) ;
#9849=CARTESIAN_POINT ( 'NONE',  ( -5.570820891630792637, 2.833901239560350671, 11.76236973443871925 ) ) ;
#9855=CARTESIAN_POINT ( 'NONE',  ( 0.1323602877612372886, 6.000000000000000000, 32.00000000000000000 ) ) ;
#9856=EDGE_LOOP ( 'NONE', ( #1335, #11214 ) ) ;
#9859=CARTESIAN_POINT ( 'NONE',  ( -3.781065399485981526, -4.978303713186466695, 12.49991741810287316 ) ) ;
#9861=CARTESIAN_POINT ( 'NONE',  ( 3.158296126777810464, 5.394094919772101981, 30.20112161576661336 ) ) ;
#9864=AXIS2_PLACEMENT_3D ( 'NONE', #12083, #1182, #10898 ) ;
#9865=CARTESIAN_POINT ( 'NONE',  ( 0.9740856415302890925, -6.173834621338562201, 24.23852653055532258 ) ) ;
#9867=CARTESIAN_POINT ( 'NONE',  ( 0.1323408341374891495, 6.250000000000001776, 12.49999999999999289 ) ) ;
#9869=CARTESIAN_POINT ( 'NONE',  ( 5.620786884546368434, -2.102685372472677727, 25.47358595436692852 ) ) ;
#9871=CARTESIAN_POINT ( 'NONE',  ( -0.5042987395407539930, -5.979983180450077818, 31.87329304179976930 ) ) ;
#9872=CARTESIAN_POINT ( 'NONE',  ( 5.531796221294883686, -2.326749136277200147, 31.87378430870261425 ) ) ;
#9873=VECTOR ( 'NONE', #3892, 1000.000000000000114 ) ;
#9874=CARTESIAN_POINT ( 'NONE',  ( -3.255013540813658679, 5.336859797930821436, 30.12618035954927009 ) ) ;
#9875=DIRECTION ( 'NONE',  ( 0.000000000000000000, 0.000000000000000000, -1.000000000000000000 ) ) ;
#9877=ORIENTED_EDGE ( 'NONE', *, *, #11085, .T. ) ;
#9880=CARTESIAN_POINT ( 'NONE',  ( -3.107688324358885090, 5.133887830459729962, 25.37378430870261781 ) ) ;
#9882=AXIS2_PLACEMENT_3D ( 'NONE', #1120, #3271, #2147 ) ;
#9884=AXIS2_PLACEMENT_3D ( 'NONE', #4071, #3754, #8629 ) ;
#9886=DIRECTION ( 'NONE',  ( 0.9510565162951500895, 0.3090169943749582204, 0.000000000000000000 ) ) ;
#9889=EDGE_CURVE ( 'NONE', #471, #15059, #14405, .T. ) ;
#9891=CYLINDRICAL_SURFACE ( 'NONE', #4187, 1.000000000000000666 ) ;
#9893=CARTESIAN_POINT ( 'NONE',  ( 5.985119669071130133, -1.805077827356517117, 10.50008258189709132 ) ) ;
#9896=AXIS2_PLACEMENT_3D ( 'NONE', #6771, #13093, #11450 ) ;
#9897=EDGE_LOOP ( 'NONE', ( #6423, #3776, #12040, #3023 ) ) ;
#9899=DIRECTION ( 'NONE',  ( -0.3090169943749584425, 0.9510565162951498674, 0.000000000000000000 ) ) ;
#9901=CARTESIAN_POINT ( 'NONE',  ( -5.725684683139550479, -2.507514573674904934, 17.20112161576660981 ) ) ;
#9902=CARTESIAN_POINT ( 'NONE',  ( 0.1323933160975826473, -5.999999999999999112, 32.00000000000000000 ) ) ;
#9903=EDGE_CURVE ( 'NONE', #12866, #12482, #12130, .T. ) ;
#9907=CARTESIAN_POINT ( 'NONE',  ( 5.317509234264001350, -2.779225709350913398, 11.63239388001634289 ) ) ;
#9908=CARTESIAN_POINT ( 'NONE',  ( -2.817313151351312328, 5.579000502529370742, 18.13237410716305220 ) ) ;
#9912=EDGE_CURVE ( 'NONE', #4153, #478, #8542, .T. ) ;
#9917=CARTESIAN_POINT ( 'NONE',  ( 0.000000000000000000, 0.000000000000000000, 0.000000000000000000 ) ) ;
#9918=CARTESIAN_POINT ( 'NONE',  ( -5.726307184802593930, 2.506131700382597582, 23.69973484982322987 ) ) ;
#9919=CARTESIAN_POINT ( 'NONE',  ( 0.6151877315910523336, -6.220340188096010081, 12.29906673469668021 ) ) ;
#9922=CARTESIAN_POINT ( 'NONE',  ( 3.882809187878787593, 4.899079348630168695, 23.52599901976669727 ) ) ;
#9924=CARTESIAN_POINT ( 'NONE',  ( 5.940390500375550609, 6.474944468551622201, 5.000000000000004441 ) ) ;
#9932=CARTESIAN_POINT ( 'NONE',  ( 4.153663429050711287, 4.670992970568434544, 12.29933148907576346 ) ) ;
#9939=CARTESIAN_POINT ( 'NONE',  ( -2.849269941562089681, -5.281123252783978650, 23.88480617551149265 ) ) ;
#9940=DIRECTION ( 'NONE',  ( 0.8090169943749421222, 0.5877852522924802425, 0.000000000000000000 ) ) ;
#9943=CARTESIAN_POINT ( 'NONE',  ( -5.621278735166254314, 2.101423246382402521, 4.025919472168996371 ) ) ;
#9944=CARTESIAN_POINT ( 'NONE',  ( -0.9740012993919509032, -6.173846968979653127, 11.76164920628437649 ) ) ;
#9949=CARTESIAN_POINT ( 'NONE',  ( -0.6156133477425491662, -6.220296490279956458, 18.79872387345510276 ) ) ;
#9950=EDGE_CURVE ( 'NONE', #4648, #6307, #8092, .T. ) ;
#9951=CARTESIAN_POINT ( 'NONE',  ( -5.531623157106135835, -2.327208526676509237, 12.37364704684421568 ) ) ;
#9952=CARTESIAN_POINT ( 'NONE',  ( 5.330189595673637371, 2.755293208590243292, 11.76382603205595956 ) ) ;
#9953=ORIENTED_EDGE ( 'NONE', *, *, #3508, .T. ) ;
#9955=VERTEX_POINT ( 'NONE', #2030 ) ;
#9958=CARTESIAN_POINT ( 'NONE',  ( -3.922672396097227399, 4.541739265057554320, 25.37364704684422634 ) ) ;
#9959=EDGE_LOOP ( 'NONE', ( #551, #3522, #6621, #10170 ) ) ;
#9962=CARTESIAN_POINT ( 'NONE',  ( 5.616116467183658756, 2.743044348085541539, 18.50425949503010159 ) ) ;
#9967=EDGE_CURVE ( 'NONE', #3666, #5746, #4156, .T. ) ;
#9969=CARTESIAN_POINT ( 'NONE',  ( 2.668367453516689469, -5.373994336898103796, 31.13061695532139339 ) ) ;
#9971=CARTESIAN_POINT ( 'NONE',  ( 6.172614129015244977, -0.9817721000788082186, 11.23763026556121503 ) ) ;
#9974=VERTEX_POINT ( 'NONE', #841 ) ;
#9976=CARTESIAN_POINT ( 'NONE',  ( 0.6144377077731314474, 5.969178481556053129, 17.20033966857735663 ) ) ;
#9979=CARTESIAN_POINT ( 'NONE',  ( 0.000000000000000000, 6.250000000000000888, 6.000000000000005329 ) ) ;
#9980=CARTESIAN_POINT ( 'NONE',  ( -4.286401442266626560, -4.198423832313095794, 18.13061695532137207 ) ) ;
#9981=B_SPLINE_CURVE_WITH_KNOTS ( 'NONE', 3,
 ( #11726, #8078, #14188, #12919, #10540, #3065, #15398, #4493, #9348, #2096, #15478, #14261, #12758, #3371, #8238, #11569, #10933, #13154 ),
 .UNSPECIFIED., .F., .F.,
 ( 4, 2, 2, 2, 2, 2, 2, 2, 4 ),
 ( 0.000000000000000000, 0.0003914898357794974410, 0.0007829796715589948820, 0.001174469507338492215, 0.001565959343117989764, 0.001957449178897485795, 0.002348939014676982261, 0.002740428850456478726, 0.003131918686235975191 ),
 .UNSPECIFIED. ) ;
#9982=CARTESIAN_POINT ( 'NONE',  ( 2.930922878467408843, -5.520395124723609825, 23.99610786875029333 ) ) ;
#9983=CARTESIAN_POINT ( 'NONE',  ( 0.6144300524835216715, 6.220417338033038313, 17.20033372175934616 ) ) ;
#9985=VECTOR ( 'NONE', #11945, 1000.000000000000114 ) ;
#9986=CARTESIAN_POINT ( 'NONE',  ( -6.172552660730998397, 0.9821660343537570448, 5.263796168408045872 ) ) ;
#9987=CARTESIAN_POINT ( 'NONE',  ( 0.6139908388542947293, -5.969238533166593363, 23.69977627912011897 ) ) ;
#9992=EDGE_CURVE ( 'NONE', #1161, #11432, #5706, .T. ) ;
#9996=EDGE_CURVE ( 'NONE', #4594, #2495, #15350, .T. ) ;
#9998=CARTESIAN_POINT ( 'NONE',  ( 2.840966774240241577, -5.567223638426863630, 11.23809786915986741 ) ) ;
#9999=CARTESIAN_POINT ( 'NONE',  ( -3.634089073485594401, 4.776071126502567488, 23.50007997643738378 ) ) ;
#10000=CARTESIAN_POINT ( 'NONE',  ( 5.616089948629698014, 2.743103014345608326, 30.49563030319847101 ) ) ;
#10002=EDGE_CURVE ( 'NONE', #4668, #7716, #12492, .T. ) ;
#10003=CARTESIAN_POINT ( 'NONE',  ( 4.195842658231396349, -4.289229542213240265, 23.99560239355786351 ) ) ;
#10005=CARTESIAN_POINT ( 'NONE',  ( 5.935543223013858949, -0.8771126767606638452, 5.000000000000004441 ) ) ;
#10007=LINE ( 'NONE', #13882, #7730 ) ;
#10009=FACE_BOUND ( 'NONE', #7875, .T. ) ;
#10012=CARTESIAN_POINT ( 'NONE',  ( 4.069684453406249958, 4.744965295353598123, 12.37380055247394672 ) ) ;
#10015=CARTESIAN_POINT ( 'NONE',  ( 6.143143148203078496, -1.154591847827606488, 18.61396179408071205 ) ) ;
#10020=CARTESIAN_POINT ( 'NONE',  ( 5.725930890718349708, -2.506952462184002250, 12.29933148907576523 ) ) ;
#10021=CARTESIAN_POINT ( 'NONE',  ( 6.780834054130108014E-14, -6.250000000000000888, 10.49999999999998224 ) ) ;
#10022=CARTESIAN_POINT ( 'NONE',  ( 4.141923667210556381, 4.342011609040548947, 17.38438267301393481 ) ) ;
#10026=CARTESIAN_POINT ( 'NONE',  ( -5.487348639458876853, 2.428538342494443114, 10.69977782616119732 ) ) ;
#10027=CARTESIAN_POINT ( 'NONE',  ( -5.487348639458853761, -2.428538342494495961, 12.30022217383879202 ) ) ;
#10032=ORIENTED_EDGE ( 'NONE', *, *, #7354, .T. ) ;
#10033=CARTESIAN_POINT ( 'NONE',  ( -5.531209434046251872, -2.328189801702823303, 23.62696220972947359 ) ) ;
#10034=VECTOR ( 'NONE', #15016, 1000.000000000000000 ) ;
#10035=EDGE_LOOP ( 'NONE', ( #2275, #13523, #1060, #1932 ) ) ;
#10037=CARTESIAN_POINT ( 'NONE',  ( -5.783239563508360881, -1.602707436861348311, 25.47358595436692852 ) ) ;
#10038=VERTEX_POINT ( 'NONE', #11473 ) ;
#10040=CARTESIAN_POINT ( 'NONE',  ( -3.255013540813639139, 5.336859797930833871, 4.126180359549289633 ) ) ;
#10042=CYLINDRICAL_SURFACE ( 'NONE', #2323, 1.000000000000000888 ) ;
#10044=AXIS2_PLACEMENT_3D ( 'NONE', #12658, #7727, #10434 ) ;
#10045=FACE_OUTER_BOUND ( 'NONE', #8129, .T. ) ;
#10047=CARTESIAN_POINT ( 'NONE',  ( 2.692335458626958999, -5.362264153667180011, 31.26239891805598248 ) ) ;
#10050=CARTESIAN_POINT ( 'NONE',  ( 3.312524433819759917, 5.004191858254014136, 12.47408052783098853 ) ) ;
#10051=VERTEX_POINT ( 'NONE', #1613 ) ;
#10052=ORIENTED_EDGE ( 'NONE', *, *, #2821, .F. ) ;
#10053=ORIENTED_EDGE ( 'NONE', *, *, #2416, .T. ) ;
#10054=CARTESIAN_POINT ( 'NONE',  ( 1.353717517954364224E-13, 6.000000000000000888, 18.99999999999998934 ) ) ;
#10055=CARTESIAN_POINT ( 'NONE',  ( 3.458623254138723624, 5.207221900902812450, 4.026227171247320769 ) ) ;
#10056=ORIENTED_EDGE ( 'NONE', *, *, #3583, .T. ) ;
#10058=CARTESIAN_POINT ( 'NONE',  ( -6.176542424588085112, -0.9554180641287668418, 17.86765874365829632 ) ) ;
#10059=CARTESIAN_POINT ( 'NONE',  ( 0.5039079366032624963, -5.980031194523149907, 30.12637068109813043 ) ) ;
#10060=CARTESIAN_POINT ( 'NONE',  ( -3.779082820360686323, 4.979770177899256467, 32.00004906876533539 ) ) ;
#10064=DIRECTION ( 'NONE',  ( -1.000000000000000000, 0.000000000000000000, 0.000000000000000000 ) ) ;
#10065=CYLINDRICAL_SURFACE ( 'NONE', #1587, 1.000000000000000666 ) ;
#10072=CARTESIAN_POINT ( 'NONE',  ( -5.570722351696237418, 2.834100162822021929, 17.73809786915987274 ) ) ;
#10073=CARTESIAN_POINT ( 'NONE',  ( 4.069684453406335223, -4.744965295353526180, 10.62619944752603374 ) ) ;
#10074=CARTESIAN_POINT ( 'NONE',  ( -0.9999505860953411540, 6.169489349035806924, 5.131059031658106839 ) ) ;
#10075=CARTESIAN_POINT ( 'NONE',  ( 6.176542424588115310, 0.9554180641285648923, 11.49999999999998224 ) ) ;
#10077=CARTESIAN_POINT ( 'NONE',  ( 4.005998022989880170, -4.467726698309333777, 23.70068193741825624 ) ) ;
#10079=DIRECTION ( 'NONE',  ( 0.5877852522924802425, -0.8090169943749422332, 0.000000000000000000 ) ) ;
#10080=CARTESIAN_POINT ( 'NONE',  ( -3.158825713737467122, -5.393784879207181859, 30.20066851092422411 ) ) ;
#10083=FACE_BOUND ( 'NONE', #15591, .T. ) ;
#10090=CARTESIAN_POINT ( 'NONE',  ( 5.903596343266337421, -2.055998103990466230, 18.99995078984292007 ) ) ;
#10093=DIRECTION ( 'NONE',  ( 0.9510565162951500895, 0.3090169943749582204, 0.000000000000000000 ) ) ;
#10095=CARTESIAN_POINT ( 'NONE',  ( 6.176542424588130409, -0.9554180641284772957, 11.63063932754212892 ) ) ;
#10099=CARTESIAN_POINT ( 'NONE',  ( 2.848727059635912884, 5.281416301279922898, 17.38557478428061387 ) ) ;
#10101=DIRECTION ( 'NONE',  ( -0.9510565162951544194, 0.3090169943749447312, 0.000000000000000000 ) ) ;
#10102=CARTESIAN_POINT ( 'NONE',  ( 3.010624175978056538, -5.190832888732173522, 5.798882422479413101 ) ) ;
#10103=CARTESIAN_POINT ( 'NONE',  ( -3.420311045507836045, 4.931422832349298346, 29.99992038825523011 ) ) ;
#10106=EDGE_LOOP ( 'NONE', ( #378, #13928, #7278, #5649 ) ) ;
#10109=ORIENTED_EDGE ( 'NONE', *, *, #6800, .T. ) ;
#10112=ORIENTED_EDGE ( 'NONE', *, *, #734, .F. ) ;
#10114=DIRECTION ( 'NONE',  ( 0.000000000000000000, 0.000000000000000000, 1.000000000000000000 ) ) ;
#10115=ORIENTED_EDGE ( 'NONE', *, *, #9207, .T. ) ;
#10117=CARTESIAN_POINT ( 'NONE',  ( -0.8737888311108684691, 5.936248257219528313, 18.50344185141215547 ) ) ;
#10124=DIRECTION ( 'NONE',  ( 0.000000000000000000, 0.000000000000000000, 1.000000000000000000 ) ) ;
#10127=EDGE_CURVE ( 'NONE', #11745, #3914, #8908, .T. ) ;
#10128=CARTESIAN_POINT ( 'NONE',  ( 7.799024015210637373, -1.482594289697068746, 31.00000000000000000 ) ) ;
#10130=ORIENTED_EDGE ( 'NONE', *, *, #15184, .T. ) ;
#10131=ORIENTED_EDGE ( 'NONE', *, *, #11259, .T. ) ;
#10132=EDGE_CURVE ( 'NONE', #6522, #478, #13054, .T. ) ;
#10133=ORIENTED_EDGE ( 'NONE', *, *, #160, .F. ) ;
#10134=CARTESIAN_POINT ( 'NONE',  ( 5.747343991580196487, -1.727858744772237332, 30.00007997643738022 ) ) ;
#10135=CARTESIAN_POINT ( 'NONE',  ( 3.882809187878947021, 4.899079348630040798, 4.025999019766705267 ) ) ;
#10136=VERTEX_POINT ( 'NONE', #14091 ) ;
#10137=CARTESIAN_POINT ( 'NONE',  ( -0.1306171417088603792, -6.000000000000000000, 4.000000000000004441 ) ) ;
#10138=CARTESIAN_POINT ( 'NONE',  ( 0.1323736289505711150, -6.249999999999999112, 18.99999999999998934 ) ) ;
#10139=CARTESIAN_POINT ( 'NONE',  ( 1.354942165116848791E-13, 6.250000000000000888, 16.99999999999998579 ) ) ;
#10142=CARTESIAN_POINT ( 'NONE',  ( 5.935543223013871383, -0.8771126767605965657, 11.63064961348853465 ) ) ;
#10145=VECTOR ( 'NONE', #13837, 1000.000000000000000 ) ;
#10152=CARTESIAN_POINT ( 'NONE',  ( -5.935543223013850955, 0.8771126767607326791, 11.63236078583908650 ) ) ;
#10153=CARTESIAN_POINT ( 'NONE',  ( 2.930922878467525194, -5.520395124723545877, 10.99610786875028445 ) ) ;
#10155=CARTESIAN_POINT ( 'NONE',  ( -0.2622538972264160106, 6.245673238944475791, 5.973859943692001906 ) ) ;
#10158=CARTESIAN_POINT ( 'NONE',  ( -4.070863287254081087, -4.743975846881804515, 31.87305891554300530 ) ) ;
#10161=CARTESIAN_POINT ( 'NONE',  ( -4.435347140101025154, -4.403429997944519947, 30.86936067245787996 ) ) ;
#10165=CARTESIAN_POINT ( 'NONE',  ( 4.344313232727052387, 4.493553492990165488, 12.00436969680152721 ) ) ;
#10168=CARTESIAN_POINT ( 'NONE',  ( 5.725930890718373689, -2.506952462183944075, 18.79933148907576523 ) ) ;
#10170=ORIENTED_EDGE ( 'NONE', *, *, #13518, .T. ) ;
#10176=CARTESIAN_POINT ( 'NONE',  ( -5.531623157106191790, 2.327208526676369349, 4.126352953155773662 ) ) ;
#10180=CARTESIAN_POINT ( 'NONE',  ( 6.172651332693093629, -0.9815532474593722245, 5.261902130840119263 ) ) ;
#10181=CARTESIAN_POINT ( 'NONE',  ( -5.558508435838135142, 2.857531096719037489, 24.49999999999999289 ) ) ;
#10182=CARTESIAN_POINT ( 'NONE',  ( -5.931734679891438766, -0.9039278060244803070, 11.23617396794405288 ) ) ;
#10183=VERTEX_POINT ( 'NONE', #10677 ) ;
#10185=EDGE_LOOP ( 'NONE', ( #12095, #14166, #1293, #1700 ) ) ;
#10186=CARTESIAN_POINT ( 'NONE',  ( -5.935543223013832304, 0.8771126767608681263, 24.63236078583910071 ) ) ;
#10188=ORIENTED_EDGE ( 'NONE', *, *, #14060, .T. ) ;
#10189=CARTESIAN_POINT ( 'NONE',  ( -5.131373506000715068, 7.062729720844030723, 5.000000000000004441 ) ) ;
#10191=CARTESIAN_POINT ( 'NONE',  ( 5.558508435838229289, -2.857531096718853192, 5.000000000000004441 ) ) ;
#10193=B_SPLINE_CURVE_WITH_KNOTS ( 'NONE', 3,
 ( #3104, #12873, #7146, #3029, #8338, #2276, #8037, #5349, #12797, #15122, #4138, #14069, #6773, #7881, #13840, #3178, #2950, #12722 ),
 .UNSPECIFIED., .F., .F.,
 ( 4, 2, 2, 2, 2, 2, 2, 2, 4 ),
 ( 0.003131918686235972155, 0.003523310662250261557, 0.003914702638264551393, 0.004306094614278841229, 0.004697486590293131065, 0.005088878566307420900, 0.005480270542321711603, 0.005871662518336002307, 0.006263054494350292142 ),
 .UNSPECIFIED. ) ;
#10194=CARTESIAN_POINT ( 'NONE',  ( -5.317509234263920526, -2.779225709351067053, 31.00000000000000000 ) ) ;
#10199=CARTESIAN_POINT ( 'NONE',  ( -5.648559266344516772, -2.676764518775952784, 5.613961794080713830 ) ) ;
#10200=CARTESIAN_POINT ( 'NONE',  ( -2.782769401326322001, 5.315896561274772836, 17.49571079637979309 ) ) ;
#10202=CARTESIAN_POINT ( 'NONE',  ( 2.082642335314403343E-14, -6.250000000000000888, 31.00000000000000000 ) ) ;
#10204=CARTESIAN_POINT ( 'NONE',  ( -0.2619041840694728007, 6.245686665308502583, 30.02605849433794916 ) ) ;
#10206=EDGE_LOOP ( 'NONE', ( #14009, #13520, #1256, #1058 ) ) ;
#10207=ORIENTED_EDGE ( 'NONE', *, *, #13868, .F. ) ;
#10208=CARTESIAN_POINT ( 'NONE',  ( 4.069800786343747312, -4.744882212776869501, 18.87381964045070859 ) ) ;
#10209=CARTESIAN_POINT ( 'NONE',  ( 6.020822430078776044, 1.681351817312468633, 4.025914576658297328 ) ) ;
#10210=ORIENTED_EDGE ( 'NONE', *, *, #11796, .T. ) ;
#10211=CARTESIAN_POINT ( 'NONE',  ( 5.746619684944318962, -1.730157667110693298, 19.00004932073311181 ) ) ;
#10213=CARTESIAN_POINT ( 'NONE',  ( 0.8736772044961308437, -6.188841968496043400, 17.49611573292809652 ) ) ;
#10214=CARTESIAN_POINT ( 'NONE',  ( -0.8738043859789770273, 6.188821459035891870, 18.50341560223740700 ) ) ;
#10220=EDGE_CURVE ( 'NONE', #4806, #15370, #10978, .T. ) ;
#10227=ORIENTED_EDGE ( 'NONE', *, *, #1127, .T. ) ;
#10228=CARTESIAN_POINT ( 'NONE',  ( 3.253823204785213807, -5.337590213880445411, 5.873058915543009739 ) ) ;
#10229=CARTESIAN_POINT ( 'NONE',  ( -6.021167129161029585, 1.680051667990390074, 23.52640428276697904 ) ) ;
#10230=CARTESIAN_POINT ( 'NONE',  ( 0.5043776560898024508, -6.230795654995834987, 12.37337476296010230 ) ) ;
#10231=CARTESIAN_POINT ( 'NONE',  ( 0.8738118504727695468, 5.936246475285000379, 25.00357242174242245 ) ) ;
#10232=EDGE_CURVE ( 'NONE', #7970, #3737, #13354, .T. ) ;
#10235=CARTESIAN_POINT ( 'NONE',  ( 2.817313151351107159, 5.579000502529474659, 5.130639327542138695 ) ) ;
#10236=CARTESIAN_POINT ( 'NONE',  ( 4.290381260516251238, -4.545736887716230967, 17.38482219624156855 ) ) ;
#10238=CARTESIAN_POINT ( 'NONE',  ( -3.923477796648506377, -4.541042560386491012, 31.87303779027052286 ) ) ;
#10243=FACE_BOUND ( 'NONE', #12506, .T. ) ;
#10244=VECTOR ( 'NONE', #4903, 1000.000000000000000 ) ;
#10245=CARTESIAN_POINT ( 'NONE',  ( 5.903596343266361401, -2.055998103990403170, 25.49995078984292718 ) ) ;
#10248=CARTESIAN_POINT ( 'NONE',  ( -5.783239563508375092, -1.602707436861291246, 18.97358595436693207 ) ) ;
#10250=ORIENTED_EDGE ( 'NONE', *, *, #9912, .F. ) ;
#10251=CARTESIAN_POINT ( 'NONE',  ( -4.416837305303536354, -4.422286678978971430, 17.73809786915987630 ) ) ;
#10252=CARTESIAN_POINT ( 'NONE',  ( 5.915755444410828012, -1.003187219519705353, 17.49687951097622474 ) ) ;
#10256=CARTESIAN_POINT ( 'NONE',  ( -5.131373506000715068, 7.062729720844030723, 5.000000000000004441 ) ) ;
#10259=CARTESIAN_POINT ( 'NONE',  ( -4.142620314836367612, 4.341347824677513678, 30.38557478428061032 ) ) ;
#10265=CARTESIAN_POINT ( 'NONE',  ( -5.486741141153698820, -2.429871531109943028, 23.70111757752058068 ) ) ;
#10270=CARTESIAN_POINT ( 'NONE',  ( -5.746996058422763731, -1.729015645941962775, 29.99992038825523721 ) ) ;
#10271=CARTESIAN_POINT ( 'NONE',  ( -0.2619456584320733472, 5.995505046955622142, 17.02607193928647078 ) ) ;
#10272=CARTESIAN_POINT ( 'NONE',  ( 5.317509234264066187, -2.779225709350791274, 24.36763921416088863 ) ) ;
#10275=CARTESIAN_POINT ( 'NONE',  ( -3.107688324358672372, -5.133887830459857859, 10.62621569129737331 ) ) ;
#10277=CARTESIAN_POINT ( 'NONE',  ( -5.558508435838095174, -2.857531096719115649, 24.49999999999999289 ) ) ;
#10279=CARTESIAN_POINT ( 'NONE',  ( 4.286401442266483564, 4.198423832313243231, 11.49999999999998224 ) ) ;
#10283=EDGE_CURVE ( 'NONE', #7176, #4447, #12003, .T. ) ;
#10285=CARTESIAN_POINT ( 'NONE',  ( 3.458623254138677883, -5.207221900902841760, 18.97377282875267568 ) ) ;
#10288=CARTESIAN_POINT ( 'NONE',  ( 5.317509234264033324, -2.779225709350852114, 17.99999999999998934 ) ) ;
#10291=CARTESIAN_POINT ( 'NONE',  ( -5.866923913994661177, 1.260079467906454198, 5.799520541027148646 ) ) ;
#10294=B_SPLINE_CURVE_WITH_KNOTS ( 'NONE', 3,
 ( #9417, #4485, #10377, #10686, #11792, #820, #10607, #9188, #15546, #6728, #7035, #12909, #12827, #13947, #657, #11865, #8149, #3056 ),
 .UNSPECIFIED., .F., .F.,
 ( 4, 2, 2, 2, 2, 2, 2, 2, 4 ),
 ( 0.000000000000000000, 0.0003914357524127495998, 0.0007828715048254991996, 0.001174307257238248799, 0.001565743009650997315, 0.001957178762063746264, 0.002348614514476494563, 0.002740050266889243295, 0.003131486019301992028 ),
 .UNSPECIFIED. ) ;
#10296=CARTESIAN_POINT ( 'NONE',  ( 4.267558728637154353, 4.217879122113844303, 11.23617396794405465 ) ) ;
#10297=EDGE_CURVE ( 'NONE', #11831, #11875, #8525, .T. ) ;
#10304=ORIENTED_EDGE ( 'NONE', *, *, #7177, .F. ) ;
#10305=CARTESIAN_POINT ( 'NONE',  ( -0.6151877315909501931, 6.220340188096019851, 12.29906673469665712 ) ) ;
#10310=CARTESIAN_POINT ( 'NONE',  ( 4.286401442266448036, -4.198423832313277870, 24.49999999999999289 ) ) ;
#10314=CARTESIAN_POINT ( 'NONE',  ( -2.817313151351126255, -5.579000502529464001, 31.00000000000000000 ) ) ;
#10317=FACE_BOUND ( 'NONE', #12175, .T. ) ;
#10319=CARTESIAN_POINT ( 'NONE',  ( -5.330004929009555248, 2.755647751839462423, 18.26239891805597537 ) ) ;
#10327=CARTESIAN_POINT ( 'NONE',  ( -4.143041610105390404, -4.340967609746952505, 17.38602261056918152 ) ) ;
#10328=FACE_OUTER_BOUND ( 'NONE', #318, .T. ) ;
#10329=CARTESIAN_POINT ( 'NONE',  ( -5.317509234263873452, 2.779225709351155871, 24.36935038651144581 ) ) ;
#10335=CARTESIAN_POINT ( 'NONE',  ( 5.859155363331463917, -2.178872204144761682, 23.52599901976669727 ) ) ;
#10336=CARTESIAN_POINT ( 'NONE',  ( 5.558508435838199979, 2.857531096718914476, 31.00000000000000000 ) ) ;
#10340=CARTESIAN_POINT ( 'NONE',  ( -0.6139908388540374906, 5.969238533166618232, 10.69977627912011364 ) ) ;
#10341=ORIENTED_EDGE ( 'NONE', *, *, #2616, .T. ) ;
#10346=CARTESIAN_POINT ( 'NONE',  ( -3.567258970015968256, 5.133675764669679786, 3.999917806784441865 ) ) ;
#10348=CARTESIAN_POINT ( 'NONE',  ( 5.531757352715673370, -2.326874507723157848, 23.62619317285289000 ) ) ;
#10354=CARTESIAN_POINT ( 'NONE',  ( 3.459597053047831494, 5.206576120509754269, 31.97408542334170178 ) ) ;
#10355=CARTESIAN_POINT ( 'NONE',  ( -0.5043776560897315075, 6.230795654995839428, 31.87337476296010053 ) ) ;
#10358=ORIENTED_EDGE ( 'NONE', *, *, #12029, .F. ) ;
#10359=ORIENTED_EDGE ( 'NONE', *, *, #586, .T. ) ;
#10360=CARTESIAN_POINT ( 'NONE',  ( 4.435347140100977192, -4.403429997944567020, 17.99999999999998934 ) ) ;
#10363=VECTOR ( 'NONE', #12547, 1000.000000000000114 ) ;
#10365=EDGE_CURVE ( 'NONE', #2495, #4594, #2636, .T. ) ;
#10367=CARTESIAN_POINT ( 'NONE',  ( -5.915641100987839351, 1.003868594704703021, 5.504289203620185589 ) ) ;
#10368=CARTESIAN_POINT ( 'NONE',  ( -4.291255145203995980, -4.544933371694754420, 4.386038205919295940 ) ) ;
#10372=CARTESIAN_POINT ( 'NONE',  ( 5.915755444410811137, 1.003187219519795725, 18.50312048902376461 ) ) ;
#10377=CARTESIAN_POINT ( 'NONE',  ( 4.416779112813551400, 4.422345839825900349, 18.26225281721714921 ) ) ;
#10382=CARTESIAN_POINT ( 'NONE',  ( -0.5043776560897083039, 6.230795654995842980, 12.37337476296007743 ) ) ;
#10384=LINE ( 'NONE', #12989, #1229 ) ;
#10385=CARTESIAN_POINT ( 'NONE',  ( 6.143143148203074055, 1.154591847827623141, 23.88603820591927729 ) ) ;
#10386=EDGE_LOOP ( 'NONE', ( #1103, #8432 ) ) ;
#10387=CARTESIAN_POINT ( 'NONE',  ( 4.344265632482074757, 4.493596842504970823, 10.99574050496990196 ) ) ;
#10388=AXIS2_PLACEMENT_3D ( 'NONE', #10189, #8927, #13760 ) ;
#10389=CARTESIAN_POINT ( 'NONE',  ( -0.2623718222033166181, -6.245654667075793753, 23.52627829713834728 ) ) ;
#10390=AXIS2_PLACEMENT_3D ( 'NONE', #2870, #3026, #7718 ) ;
#10391=CARTESIAN_POINT ( 'NONE',  ( 4.153663429050745037, -4.670992970568404345, 17.20066851092423121 ) ) ;
#10392=B_SPLINE_CURVE_WITH_KNOTS ( 'NONE', 3,
 ( #10975, #5815, #13038, #13205, #3494, #8445, #8528, #7007, #14477, #13281, #15518, #14301, #74, #5892, #8365, #12166, #9717, #2298 ),
 .UNSPECIFIED., .F., .F.,
 ( 4, 2, 2, 2, 2, 2, 2, 2, 4 ),
 ( 0.003131918686235972155, 0.003523310662250263292, 0.003914702638264554863, 0.004306094614278846433, 0.004697486590293137136, 0.005088878566307428707, 0.005480270542321718542, 0.005871662518336009245, 0.006263054494350299081 ),
 .UNSPECIFIED. ) ;
#10398=CARTESIAN_POINT ( 'NONE',  ( -2.668367453516752974, -5.373994336898072710, 17.99999999999998934 ) ) ;
#10399=CARTESIAN_POINT ( 'NONE',  ( 0.2637975869348134772, 6.245592211692891027, 25.47332839949195460 ) ) ;
#10402=DIRECTION ( 'NONE',  ( 0.000000000000000000, 1.000000000000000000, 0.000000000000000000 ) ) ;
#10405=CYLINDRICAL_SURFACE ( 'NONE', #13991, 1.000000000000000666 ) ;
#10409=CARTESIAN_POINT ( 'NONE',  ( 5.935543223013866942, 0.8771126767606117758, 17.99999999999998934 ) ) ;
#10412=CARTESIAN_POINT ( 'NONE',  ( 2.668367453516524268, -5.373994336898184621, 24.49999999999999289 ) ) ;
#10413=CARTESIAN_POINT ( 'NONE',  ( -5.746837578676003311, -1.729433780394259879, 5.999950536462232087 ) ) ;
#10415=CARTESIAN_POINT ( 'NONE',  ( 5.903596343266293012, -2.055998103990597681, 5.999950789842938725 ) ) ;
#10420=CARTESIAN_POINT ( 'NONE',  ( 4.267558728637180998, 4.217879122113815882, 30.73617396794403689 ) ) ;
#10422=AXIS2_PLACEMENT_3D ( 'NONE', #3954, #10093, #6523 ) ;
#10423=CARTESIAN_POINT ( 'NONE',  ( 5.317509234264033324, -2.779225709350852114, 17.99999999999998934 ) ) ;
#10424=CARTESIAN_POINT ( 'NONE',  ( -2.692215568229726852, -5.362327947133653794, 4.737709621640688873 ) ) ;
#10425=CARTESIAN_POINT ( 'NONE',  ( -7.180990026460726483, -3.384707322287581199, 11.49999999999998224 ) ) ;
#10427=CARTESIAN_POINT ( 'NONE',  ( 4.435347140100914132, 4.403429997944631857, 17.99999999999998934 ) ) ;
#10429=EDGE_CURVE ( 'NONE', #642, #3364, #2438, .T. ) ;
#10430=CARTESIAN_POINT ( 'NONE',  ( -4.154121946520847430, -4.670585111242995247, 5.798878384233395522 ) ) ;
#10432=CARTESIAN_POINT ( 'NONE',  ( -5.725684683139609099, -2.507514573674767266, 4.201121615766616024 ) ) ;
#10434=DIRECTION ( 'NONE',  ( -0.3090169943749579429, 0.9510565162951502005, 0.000000000000000000 ) ) ;
#10435=CARTESIAN_POINT ( 'NONE',  ( 4.286401442266437378, 4.198423832313292081, 17.99999999999998934 ) ) ;
#10436=FACE_OUTER_BOUND ( 'NONE', #5824, .T. ) ;
#10438=ORIENTED_EDGE ( 'NONE', *, *, #12522, .T. ) ;
#10439=ORIENTED_EDGE ( 'NONE', *, *, #993, .T. ) ;
#10440=CARTESIAN_POINT ( 'NONE',  ( 4.290130679986521756, -4.545972905167772637, 18.61560192892921606 ) ) ;
#10441=CARTESIAN_POINT ( 'NONE',  ( 6.123233995736766282E-16, -6.250000000000000888, 5.000000000000004441 ) ) ;
#10442=ORIENTED_EDGE ( 'NONE', *, *, #4773, .T. ) ;
#10445=CARTESIAN_POINT ( 'NONE',  ( 6.143020266950989239, 1.155160780047645552, 18.61441947245482709 ) ) ;
#10446=CARTESIAN_POINT ( 'NONE',  ( -4.344502777243494762, -4.493369211529300244, 4.496107868750330638 ) ) ;
#10449=APPLICATION_CONTEXT ( 'automotive_design' ) ;
#10453=CARTESIAN_POINT ( 'NONE',  ( -5.915641100987822476, -1.003868594704795836, 4.495710796379801977 ) ) ;
#10459=ORIENTED_EDGE ( 'NONE', *, *, #10132, .F. ) ;
#10460=CARTESIAN_POINT ( 'NONE',  ( -0.8002720181890271567, 6.199262377003415203, 10.88606262465555119 ) ) ;
#10461=DIRECTION ( 'NONE',  ( -0.9510565162951545304, 0.3090169943749447867, 0.000000000000000000 ) ) ;
#10462=CARTESIAN_POINT ( 'NONE',  ( -6.176542424588117974, 0.9554180641285661135, 31.00000000000000000 ) ) ;
#10463=EDGE_LOOP ( 'NONE', ( #2811, #4465, #3197, #8482 ) ) ;
#10464=CARTESIAN_POINT ( 'NONE',  ( -4.435347140101154828, -4.403429997944389385, 24.49999999999999289 ) ) ;
#10465=CARTESIAN_POINT ( 'NONE',  ( 2.094888803305876858E-14, -6.250000000000000888, 30.00000000000000000 ) ) ;
#10468=CARTESIAN_POINT ( 'NONE',  ( -7.490007020835642848, -2.433650805992559896, 24.49999999999999289 ) ) ;
#10469=PRESENTATION_STYLE_ASSIGNMENT (( #8163 ) ) ;
#10472=EDGE_CURVE ( 'NONE', #8099, #13328, #14013, .T. ) ;
#10474=CARTESIAN_POINT ( 'NONE',  ( 6.143020266951007002, -1.155160780047555180, 17.38558052754515160 ) ) ;
#10475=CARTESIAN_POINT ( 'NONE',  ( -5.931734679891438766, 0.9039278060244781976, 18.26382603205596311 ) ) ;
#10480=CARTESIAN_POINT ( 'NONE',  ( 2.817313151351005462, -5.579000502529526173, 24.63060690723498070 ) ) ;
#10490=CARTESIAN_POINT ( 'NONE',  ( -5.131373506000823426, 7.062729720843950787, 17.99999999999998934 ) ) ;
#10491=CARTESIAN_POINT ( 'NONE',  ( -0.9735856429312665927, 5.920699391845031023, 31.26285283906726775 ) ) ;
#10493=FACE_BOUND ( 'NONE', #9497, .T. ) ;
#10498=CARTESIAN_POINT ( 'NONE',  ( -0.1323933160974937739, 6.000000000000002665, 12.49999999999998757 ) ) ;
#10500=DIRECTION ( 'NONE',  ( 0.5877852522924802425, -0.8090169943749422332, 0.000000000000000000 ) ) ;
#10503=CARTESIAN_POINT ( 'NONE',  ( 5.931828553037980178, 0.9033193133618800941, 17.73805675996853637 ) ) ;
#10505=DIRECTION ( 'NONE',  ( -0.9510565162951545304, 0.3090169943749447867, 0.000000000000000000 ) ) ;
#10508=CARTESIAN_POINT ( 'NONE',  ( -6.172552660730982410, -0.9821660343538520799, 4.736203831591939917 ) ) ;
#10510=DIRECTION ( 'NONE',  ( -0.5877852522924685852, -0.8090169943749507819, 0.000000000000000000 ) ) ;
#10511=CARTESIAN_POINT ( 'NONE',  ( 4.290381260516270778, 4.545736887716210539, 31.61517780375841369 ) ) ;
#10513=CARTESIAN_POINT ( 'NONE',  ( -0.7995298244853260572, -5.947211616899265252, 18.61456014619857058 ) ) ;
#10514=EDGE_LOOP ( 'NONE', ( #11565, #6366 ) ) ;
#10516=EDGE_LOOP ( 'NONE', ( #10874, #13153, #12448, #829 ) ) ;
#10517=ORIENTED_EDGE ( 'NONE', *, *, #3570, .T. ) ;
#10518=CARTESIAN_POINT ( 'NONE',  ( 2.996920846510537473, -5.485395142346763286, 12.11441947245483064 ) ) ;
#10519=DIRECTION ( 'NONE',  ( 0.000000000000000000, 0.000000000000000000, -1.000000000000000000 ) ) ;
#10520=ORIENTED_EDGE ( 'NONE', *, *, #11555, .T. ) ;
#10521=CARTESIAN_POINT ( 'NONE',  ( 5.409274167810711909, -2.597759609440523754, 18.61519382448850024 ) ) ;
#10523=CARTESIAN_POINT ( 'NONE',  ( 0.6139908388541017725, -5.969238533166612015, 4.199776279120133182 ) ) ;
#10527=CARTESIAN_POINT ( 'NONE',  ( -7.490007020835684592, -2.433650805992431110, 11.49999999999998224 ) ) ;
#10530=DIRECTION ( 'NONE',  ( 0.9510565162951499785, 0.3090169943749582204, 0.000000000000000000 ) ) ;
#10535=EDGE_LOOP ( 'NONE', ( #5789, #3527 ) ) ;
#10536=CARTESIAN_POINT ( 'NONE',  ( 3.780072143464286771, -4.979057943639690897, 6.000082193215566129 ) ) ;
#10537=DIRECTION ( 'NONE',  ( -0.9510565162951545304, 0.3090169943749447867, 0.000000000000000000 ) ) ;
#10538=CARTESIAN_POINT ( 'NONE',  ( 5.649053410273122466, 2.675685104943152481, 23.88482219624157210 ) ) ;
#10540=CARTESIAN_POINT ( 'NONE',  ( -5.903119516422468571, 1.077859910107537678, 17.38480617551147844 ) ) ;
#10541=CYLINDRICAL_SURFACE ( 'NONE', #7672, 6.250000000000000888 ) ;
#10549=FACE_BOUND ( 'NONE', #4709, .T. ) ;
#10550=CARTESIAN_POINT ( 'NONE',  ( 2.082642335314403343E-14, -6.250000000000000888, 32.00000000000000000 ) ) ;
#10552=B_SPLINE_CURVE_WITH_KNOTS ( 'NONE', 3,
 ( #8409, #14116, #15323, #9433, #6972, #10701, #1071, #9278, #4662, #2102, #15639, #14266, #11730, #9513, #11805, #9352, #2260, #7130 ),
 .UNSPECIFIED., .F., .F.,
 ( 4, 2, 2, 2, 2, 2, 2, 2, 4 ),
 ( 0.003131486019301972078, 0.003522824630466680519, 0.003914163241631389394, 0.004305501852796097401, 0.004696840463960806275, 0.005088179075125516017, 0.005479517686290224891, 0.005870856297454934633, 0.006262194908619643507 ),
 .UNSPECIFIED. ) ;
#10554=CARTESIAN_POINT ( 'NONE',  ( -5.131373506000731055, 7.062729720844018289, 31.00000000000000000 ) ) ;
#10555=DIRECTION ( 'NONE',  ( -0.9510565162951544194, 0.3090169943749447312, 0.000000000000000000 ) ) ;
#10556=ORIENTED_EDGE ( 'NONE', *, *, #15433, .T. ) ;
#10557=CARTESIAN_POINT ( 'NONE',  ( -5.984759433606986256, 1.806271833852362008, 19.00008219321555103 ) ) ;
#10559=EDGE_CURVE ( 'NONE', #1584, #2087, #8709, .T. ) ;
#10564=CARTESIAN_POINT ( 'NONE',  ( -5.621278735166225893, -2.101423246382475352, 5.974080527831013399 ) ) ;
#10566=FACE_BOUND ( 'NONE', #1527, .T. ) ;
#10568=CARTESIAN_POINT ( 'NONE',  ( 0.7988914244718454682, 5.947301735519280541, 30.38456289168619051 ) ) ;
#10571=CARTESIAN_POINT ( 'NONE',  ( -0.5039079366031817830, 5.980031194523157012, 10.62637068109811622 ) ) ;
#10573=ORIENTED_EDGE ( 'NONE', *, *, #2981, .F. ) ;
#10574=FACE_OUTER_BOUND ( 'NONE', #10035, .T. ) ;
#10579=CARTESIAN_POINT ( 'NONE',  ( -0.8736772044957569205, 6.188841968496095802, 23.99611573292804678 ) ) ;
#10581=CARTESIAN_POINT ( 'NONE',  ( 2.668367453516645504, -5.373994336898123336, 11.49999999999998224 ) ) ;
#10583=CARTESIAN_POINT ( 'NONE',  ( 0.8738043859790958212, -6.188821459035875883, 31.50341560223748161 ) ) ;
#10585=CARTESIAN_POINT ( 'NONE',  ( 6.000000000000000888, 7.347880794884120722E-16, 36.00000000000000711 ) ) ;
#10590=CARTESIAN_POINT ( 'NONE',  ( 4.069800786343767740, 4.744882212776853514, 30.12618035954928430 ) ) ;
#10596=CARTESIAN_POINT ( 'NONE',  ( 0.1306497350717338857, -6.000000000000001776, 4.000000000000004441 ) ) ;
#10597=CARTESIAN_POINT ( 'NONE',  ( 3.568242062701365125, 5.132954954975621931, 25.50004906876533184 ) ) ;
#10599=EDGE_CURVE ( 'NONE', #2087, #1584, #6431, .T. ) ;
#10606=EDGE_CURVE ( 'NONE', #3644, #6042, #5740, .T. ) ;
#10607=CARTESIAN_POINT ( 'NONE',  ( 4.069684453406205549, 4.744965295353637202, 18.87380055247394850 ) ) ;
#10608=ORIENTED_EDGE ( 'NONE', *, *, #6498, .F. ) ;
#10611=ORIENTED_EDGE ( 'NONE', *, *, #10220, .F. ) ;
#10614=CYLINDRICAL_SURFACE ( 'NONE', #714, 1.000000000000000666 ) ;
#10615=CARTESIAN_POINT ( 'NONE',  ( -0.7993282387951125001, 5.947240459526509149, 5.614843582169575242 ) ) ;
#10616=ORIENTED_EDGE ( 'NONE', *, *, #2375, .T. ) ;
#10617=CARTESIAN_POINT ( 'NONE',  ( 5.131373506000584506, 7.062729720844102665, 31.00000000000000000 ) ) ;
#10618=UNCERTAINTY_MEASURE_WITH_UNIT (LENGTH_MEASURE( 1.000000000000000082E-05 ), #14072, 'distance_accuracy_value', 'NONE');
#10619=CARTESIAN_POINT ( 'NONE',  ( 5.409423237179077582, -2.597448116730894263, 17.38438267301393481 ) ) ;
#10620=DIRECTION ( 'NONE',  ( 0.5877852522924802425, -0.8090169943749422332, 0.000000000000000000 ) ) ;
#10623=CARTESIAN_POINT ( 'NONE',  ( -6.176542424588095770, -0.9554180641287001174, 11.49999999999998224 ) ) ;
#10624=( NAMED_UNIT ( * ) PLANE_ANGLE_UNIT ( ) SI_UNIT ( $, .RADIAN. ) );
#10625=VECTOR ( 'NONE', #2709, 1000.000000000000000 ) ;
#10626=DIRECTION ( 'NONE',  ( -0.3090169943749579429, 0.9510565162951502005, 0.000000000000000000 ) ) ;
#10628=AXIS2_PLACEMENT_3D ( 'NONE', #2296, #9715, #149 ) ;
#10630=CARTESIAN_POINT ( 'NONE',  ( 5.746619684944269224, 1.730157667110847397, 10.49995067926686154 ) ) ;
#10631=CARTESIAN_POINT ( 'NONE',  ( 5.931793676715084729, 0.9035324301689270365, 31.26239891805597537 ) ) ;
#10637=AXIS2_PLACEMENT_3D ( 'NONE', #14212, #8105, #692 ) ;
#10642=CARTESIAN_POINT ( 'NONE',  ( -4.435347140101077557, 4.403429997944469321, 5.130639327542137806 ) ) ;
#10644=FACE_BOUND ( 'NONE', #8926, .T. ) ;
#10649=EDGE_CURVE ( 'NONE', #8460, #9974, #1112, .T. ) ;
#10653=MECHANICAL_DESIGN_GEOMETRIC_PRESENTATION_REPRESENTATION('',(#3282),#1508);
#10656=CARTESIAN_POINT ( 'NONE',  ( 2.817313151350985034, 5.579000502529534167, 17.99999999999998934 ) ) ;
#10658=CARTESIAN_POINT ( 'NONE',  ( 4.286401442266576822, -4.198423832313147308, 30.86760611998364112 ) ) ;
#10660=CARTESIAN_POINT ( 'NONE',  ( 3.107278289587213749, -5.134157760522037428, 10.62635295315575767 ) ) ;
#10664=CARTESIAN_POINT ( 'NONE',  ( 5.665707375537457402, 1.979196487016721573, 12.50007961174474858 ) ) ;
#10666=ORIENTED_EDGE ( 'NONE', *, *, #9996, .T. ) ;
#10667=( GEOMETRIC_REPRESENTATION_CONTEXT ( 3 ) GLOBAL_UNCERTAINTY_ASSIGNED_CONTEXT ( ( #675 ) ) GLOBAL_UNIT_ASSIGNED_CONTEXT ( ( #4499, #10624, #8322 ) ) REPRESENTATION_CONTEXT ( 'NONE', 'WORKASPACE' ) );
#10668=ADVANCED_FACE ( 'NONE', ( #6254 ), #2741, .F. ) ;
#10671=CARTESIAN_POINT ( 'NONE',  ( 4.195795028114968517, -4.289273350251384898, 25.00428920362019625 ) ) ;
#10676=CARTESIAN_POINT ( 'NONE',  ( -5.746837578675995317, -1.729433780394289188, 31.99995053646223653 ) ) ;
#10677=CARTESIAN_POINT ( 'NONE',  ( 4.286401442266388528, 4.198423832313340043, 24.49999999999999289 ) ) ;
#10683=B_SPLINE_CURVE_WITH_KNOTS ( 'NONE', 3,
 ( #12785, #13827, #695, #5337, #11364, #1734, #15111, #4209, #10415, #15265, #9079, #6609, #4366, #2781, #2940, #10180, #4047, #11442 ),
 .UNSPECIFIED., .F., .F.,
 ( 4, 2, 2, 2, 2, 2, 2, 2, 4 ),
 ( 0.000000000000000000, 0.0003914357524127484072, 0.0007828715048254968143, 0.001174307257238245330, 0.001565743009650993629, 0.001957178762063741927, 0.002348614514476490660, 0.002740050266889238959, 0.003131486019301987257 ),
 .UNSPECIFIED. ) ;
#10686=CARTESIAN_POINT ( 'NONE',  ( 4.344313232727004426, 4.493553492990209897, 18.50436969680152899 ) ) ;
#10687=ORIENTED_EDGE ( 'NONE', *, *, #10232, .T. ) ;
#10689=ORIENTED_EDGE ( 'NONE', *, *, #12897, .T. ) ;
#10691=CARTESIAN_POINT ( 'NONE',  ( -6.081509788407712058, 1.446521464462830142, 25.37381964045071214 ) ) ;
#10692=CARTESIAN_POINT ( 'NONE',  ( 3.011899281037397458, -5.190111395030288399, 17.19977782616120265 ) ) ;
#10693=CARTESIAN_POINT ( 'NONE',  ( 0.1306394121199382363, -6.250000000000000888, 4.000000000000005329 ) ) ;
#10694=ORIENTED_EDGE ( 'NONE', *, *, #8523, .T. ) ;
#10695=CARTESIAN_POINT ( 'NONE',  ( -5.570820891630815730, 2.833901239560305818, 31.26236973443877076 ) ) ;
#10697=EDGE_CURVE ( 'NONE', #7319, #1678, #4728, .T. ) ;
#10698=CARTESIAN_POINT ( 'NONE',  ( -0.9737725088280243524, -6.173885267451852954, 24.23735758726565592 ) ) ;
#10699=CARTESIAN_POINT ( 'NONE',  ( -4.344502777243604896, 4.493369211529193663, 12.00389213124967114 ) ) ;
#10700=CARTESIAN_POINT ( 'NONE',  ( 0.9999502950803423884, -5.916088184763861335, 18.13108149190010465 ) ) ;
#10701=CARTESIAN_POINT ( 'NONE',  ( -4.154121946521006414, -4.670585111242854914, 25.29887838423338309 ) ) ;
#10704=ADVANCED_FACE ( 'NONE', ( #1690 ), #13940, .F. ) ;
#10707=CARTESIAN_POINT ( 'NONE',  ( 5.571002711501477300, -2.833546409886150030, 17.73620383159192571 ) ) ;
#10709=EDGE_CURVE ( 'NONE', #1252, #28, #580, .T. ) ;
#10711=CARTESIAN_POINT ( 'NONE',  ( -4.286401442266592809, 4.198423832313131321, 5.000000000000004441 ) ) ;
#10712=CYLINDRICAL_SURFACE ( 'NONE', #12254, 1.000000000000000888 ) ;
#10725=CARTESIAN_POINT ( 'NONE',  ( 0.000000000000000000, 0.000000000000000000, 53.67766952966368876 ) ) ;
#10727=CARTESIAN_POINT ( 'NONE',  ( 6.143143148203063397, 1.154591847827682871, 17.38603820591927729 ) ) ;
#10728=EDGE_LOOP ( 'NONE', ( #3232, #14293 ) ) ;
#10732=CYLINDRICAL_SURFACE ( 'NONE', #11883, 1.000000000000000888 ) ;
#10733=ORIENTED_EDGE ( 'NONE', *, *, #8936, .T. ) ;
#10735=CARTESIAN_POINT ( 'NONE',  ( -4.435347140101121965, 4.403429997944421359, 11.49999999999998224 ) ) ;
#10736=CARTESIAN_POINT ( 'NONE',  ( -3.735642931251060617, 4.696778275484448706, 31.97408052783100985 ) ) ;
#10739=CARTESIAN_POINT ( 'NONE',  ( 4.286401442266577710, -4.198423832313146420, 31.00000000000000000 ) ) ;
#10743=CARTESIAN_POINT ( 'NONE',  ( -5.931817299736853677, 0.9033986943601943764, 11.23770962164068976 ) ) ;
#10745=CARTESIAN_POINT ( 'NONE',  ( -0.2624013748571840110, -5.995472630654527180, 17.02628559691081733 ) ) ;
#10746=ORIENTED_EDGE ( 'NONE', *, *, #14068, .F. ) ;
#10748=ORIENTED_EDGE ( 'NONE', *, *, #7650, .T. ) ;
#10750=B_SPLINE_CURVE_WITH_KNOTS ( 'NONE', 3,
 ( #3373, #8240, #10389, #13074, #11879, #989, #5853, #10698, #7916, #4340, #4659, #9197, #6093, #15636, #5052, #112, #8406, #13394 ),
 .UNSPECIFIED., .F., .F.,
 ( 4, 2, 2, 2, 2, 2, 2, 2, 4 ),
 ( 0.003131490185286093120, 0.003522829482338693183, 0.003914168779391293679, 0.004305508076443894175, 0.004696847373496493804, 0.005088186670549094300, 0.005479525967601693928, 0.005870865264654294424, 0.006262204561706894920 ),
 .UNSPECIFIED. ) ;
#10751=CARTESIAN_POINT ( 'NONE',  ( -2.668367453516768517, 5.373994336898062052, 11.49999999999998224 ) ) ;
#10752=EDGE_LOOP ( 'NONE', ( #8850, #12971 ) ) ;
#10755=LINE ( 'NONE', #5675, #8846 ) ;
#10761=CARTESIAN_POINT ( 'NONE',  ( 5.649200442566173486, -2.675373855294116865, 4.384398071070796377 ) ) ;
#10764=CARTESIAN_POINT ( 'NONE',  ( 2.930922878467574488, -5.520395124723521896, 30.49610786875030044 ) ) ;
#10766=CARTESIAN_POINT ( 'NONE',  ( 5.558508435838189321, 2.857531096718932240, 5.000000000000004441 ) ) ;
#10768=VERTEX_POINT ( 'NONE', #7902 ) ;
#10772=CARTESIAN_POINT ( 'NONE',  ( -6.176542424588101987, -0.9554180641286524889, 31.00000000000000000 ) ) ;
#10773=CARTESIAN_POINT ( 'NONE',  ( -3.255128505894383739, -5.336774832660674761, 23.62619944752604439 ) ) ;
#10775=CARTESIAN_POINT ( 'NONE',  ( -5.558508435838179551, -2.857531096718951336, 31.00000000000000000 ) ) ;
#10777=CARTESIAN_POINT ( 'NONE',  ( -0.8738239080080343335, -6.188820299975591688, 5.503557957101422815 ) ) ;
#10780=CARTESIAN_POINT ( 'NONE',  ( 5.531796221294850824, 2.326749136277279639, 30.12621569129737864 ) ) ;
#10781=CARTESIAN_POINT ( 'NONE',  ( 0.1323933160977649182, -5.999999999999995559, 25.49999999999999289 ) ) ;
#10785=CARTESIAN_POINT ( 'NONE',  ( -5.570722351696197450, -2.834100162822098756, 18.26190213084011660 ) ) ;
#10787=EDGE_LOOP ( 'NONE', ( #2557, #324 ) ) ;
#10789=CARTESIAN_POINT ( 'NONE',  ( -0.7988914244717549851, -5.947301735519293864, 10.88456289168616742 ) ) ;
#10790=ORIENTED_EDGE ( 'NONE', *, *, #12054, .T. ) ;
#10793=CARTESIAN_POINT ( 'NONE',  ( 4.344265632481963735, 4.493596842505074740, 23.99574050496988775 ) ) ;
#10794=VECTOR ( 'NONE', #10510, 1000.000000000000114 ) ;
#10800=CARTESIAN_POINT ( 'NONE',  ( -3.458467055437274063, 5.207305717053841043, 5.973595717233013858 ) ) ;
#10802=CARTESIAN_POINT ( 'NONE',  ( 5.984377695197225400, 1.807429553002283029, 10.49995093123465217 ) ) ;
#10806=VERTEX_POINT ( 'NONE', #13514 ) ;
#10809=CARTESIAN_POINT ( 'NONE',  ( 5.935543223013877601, 0.8771126767605439412, 24.36935038651144581 ) ) ;
#10810=B_SPLINE_CURVE_WITH_KNOTS ( 'NONE', 3,
 ( #8689, #157, #5020, #2469, #12091, #2386, #8372, #14483, #4867, #1269, #4, #14561, #8613, #3657, #3736, #10823, #1116, #6296 ),
 .UNSPECIFIED., .F., .F.,
 ( 4, 2, 2, 2, 2, 2, 2, 2, 4 ),
 ( 0.000000000000000000, 0.0003914898357794965736, 0.0007829796715589933641, 0.001174469507338490046, 0.001565959343117987162, 0.001957449178897483627, 0.002348939014676980092, 0.002740428850456476557, 0.003131918686235973456 ),
 .UNSPECIFIED. ) ;
#10812=VERTEX_POINT ( 'NONE', #4780 ) ;
#10813=CARTESIAN_POINT ( 'NONE',  ( 1.000049271338691481, -6.169473353325520826, 24.36969612704551125 ) ) ;
#10814=CARTESIAN_POINT ( 'NONE',  ( -4.322356511625772058, 7.650514973136511188, 5.000000000000004441 ) ) ;
#10815=CYLINDRICAL_SURFACE ( 'NONE', #13416, 1.000000000000000888 ) ;
#10817=CARTESIAN_POINT ( 'NONE',  ( 2.668367453516690357, -5.373994336898101132, 31.00000000000000000 ) ) ;
#10819=CARTESIAN_POINT ( 'NONE',  ( 5.935543223013876712, 0.8771126767605440522, 24.49999999999999289 ) ) ;
#10820=CARTESIAN_POINT ( 'NONE',  ( 5.935543223013864278, -0.8771126767606430841, 31.13064961348856130 ) ) ;
#10823=CARTESIAN_POINT ( 'NONE',  ( -5.329907877631385738, 2.755840666746196543, 30.73805675996854703 ) ) ;
#10826=ORIENTED_EDGE ( 'NONE', *, *, #11157, .F. ) ;
#10829=PRODUCT_DEFINITION_SHAPE ( 'NONE', 'NONE',  #2335 ) ;
#10831=CARTESIAN_POINT ( 'NONE',  ( 5.558508435838253270, 2.857531096718811892, 17.99999999999998934 ) ) ;
#10832=CARTESIAN_POINT ( 'NONE',  ( 6.143020266950968811, 1.155160780047759683, 31.61441947245484485 ) ) ;
#10838=CYLINDRICAL_SURFACE ( 'NONE', #2512, 1.000000000000000666 ) ;
#10840=CARTESIAN_POINT ( 'NONE',  ( 6.155973317223274677, 1.081218830693777777, 5.503086438660448998 ) ) ;
#10841=EDGE_LOOP ( 'NONE', ( #15498, #1174 ) ) ;
#10847=CARTESIAN_POINT ( 'NONE',  ( -5.984759433606997803, -1.806271833852329145, 29.99991780678443476 ) ) ;
#10849=CARTESIAN_POINT ( 'NONE',  ( 6.176542424588136626, 0.9554180641284277797, 24.49999999999999289 ) ) ;
#10851=CARTESIAN_POINT ( 'NONE',  ( -5.558508435838219519, 2.857531096718872732, 31.00000000000000000 ) ) ;
#10853=CARTESIAN_POINT ( 'NONE',  ( -3.736532060717985715, -4.696070028785973349, 12.47377823943291908 ) ) ;
#10855=CARTESIAN_POINT ( 'NONE',  ( -5.858813228503575665, -2.179803269293471679, 23.52622717124730656 ) ) ;
#10856=FACE_OUTER_BOUND ( 'NONE', #8635, .T. ) ;
#10862=CARTESIAN_POINT ( 'NONE',  ( 5.317509234263964046, 2.779225709350989337, 11.36760611998364823 ) ) ;
#10867=ORIENTED_EDGE ( 'NONE', *, *, #6103, .T. ) ;
#10868=CARTESIAN_POINT ( 'NONE',  ( -4.006441409774724960, 4.467329318258222770, 4.201117577520601998 ) ) ;
#10874=ORIENTED_EDGE ( 'NONE', *, *, #11819, .F. ) ;
#10877=VECTOR ( 'NONE', #11672, 1000.000000000000114 ) ;
#10881=CARTESIAN_POINT ( 'NONE',  ( -1.000082492230699671, -6.169467968613712827, 31.13152538105391542 ) ) ;
#10883=DIRECTION ( 'NONE',  ( 0.000000000000000000, 1.000000000000000000, 0.000000000000000000 ) ) ;
#10888=ORIENTED_EDGE ( 'NONE', *, *, #3118, .T. ) ;
#10890=VECTOR ( 'NONE', #5515, 1000.000000000000114 ) ;
#10892=CARTESIAN_POINT ( 'NONE',  ( 5.317509234264027107, 2.779225709350867213, 24.49999999999999289 ) ) ;
#10894=ADVANCED_FACE ( 'NONE', ( #3320 ), #14285, .F. ) ;
#10897=CARTESIAN_POINT ( 'NONE',  ( 5.558508435838239059, -2.857531096718835428, 31.00000000000000000 ) ) ;
#10898=DIRECTION ( 'NONE',  ( -0.3090169943749579429, 0.9510565162951502005, 0.000000000000000000 ) ) ;
#10900=CARTESIAN_POINT ( 'NONE',  ( 3.922288969639839085, -4.542045818322474560, 30.12621569129737864 ) ) ;
#10905=CARTESIAN_POINT ( 'NONE',  ( -0.8738239080078950005, -6.188820299975613004, 18.50355795710142104 ) ) ;
#10906=CARTESIAN_POINT ( 'NONE',  ( 5.843075991566563765, 1.368655265451134140, 4.126352953155773662 ) ) ;
#10907=CARTESIAN_POINT ( 'NONE',  ( 5.317509234263963158, 2.779225709350988449, 11.49999999999998224 ) ) ;
#10909=EDGE_LOOP ( 'NONE', ( #4412, #5714, #4568, #7969 ) ) ;
#10912=DIRECTION ( 'NONE',  ( -0.9510565162951545304, 0.3090169943749447867, 0.000000000000000000 ) ) ;
#10917=CARTESIAN_POINT ( 'NONE',  ( 5.985119669071097270, 1.805077827356622588, 31.99991741810289625 ) ) ;
#10920=CARTESIAN_POINT ( 'NONE',  ( -5.782947755040681592, 1.603807858343930137, 31.97398020122239259 ) ) ;
#10924=VERTEX_POINT ( 'NONE', #6916 ) ;
#10925=ORIENTED_EDGE ( 'NONE', *, *, #7022, .F. ) ;
#10926=LINE ( 'NONE', #15040, #10625 ) ;
#10928=ORIENTED_EDGE ( 'NONE', *, *, #11585, .F. ) ;
#10929=CARTESIAN_POINT ( 'NONE',  ( -6.176542424588088664, 0.9554180641287480791, 24.49999999999999289 ) ) ;
#10930=CARTESIAN_POINT ( 'NONE',  ( 2.782468714962326395, -5.316055268221460572, 17.49610204984018225 ) ) ;
#10931=( GEOMETRIC_REPRESENTATION_CONTEXT ( 3 ) GLOBAL_UNCERTAINTY_ASSIGNED_CONTEXT ( ( #8006 ) ) GLOBAL_UNIT_ASSIGNED_CONTEXT ( ( #8244, #13078, #3148 ) ) REPRESENTATION_CONTEXT ( 'NONE', 'WORKASPACE' ) );
#10932=CARTESIAN_POINT ( 'NONE',  ( -4.286401442266677186, -4.198423832313046944, 24.63061695532137918 ) ) ;
#10933=CARTESIAN_POINT ( 'NONE',  ( -5.317509234263907203, 2.779225709351096807, 17.86935038651143159 ) ) ;
#10934=B_SPLINE_CURVE_WITH_KNOTS ( 'NONE', 3,
 ( #11433, #8992, #8828, #7544, #6598, #5483, #1571, #1801, #13894, #13581, #303, #610, #12626, #10327, #1724, #1489, #535, #15103 ),
 .UNSPECIFIED., .F., .F.,
 ( 4, 2, 2, 2, 2, 2, 2, 2, 4 ),
 ( 0.000000000000000000, 0.0003914898357794968447, 0.0007829796715589936893, 0.001174469507338490480, 0.001565959343117987379, 0.001957449178897484061, 0.002348939014676980960, 0.002740428850456477858, 0.003131918686235974757 ),
 .UNSPECIFIED. ) ;
#10935=CARTESIAN_POINT ( 'NONE',  ( 3.779681992289718906, -4.979315417303956437, 23.50004921015706216 ) ) ;
#10937=CARTESIAN_POINT ( 'NONE',  ( -5.558508435838229289, 2.857531096718854524, 5.000000000000004441 ) ) ;
#10938=CARTESIAN_POINT ( 'NONE',  ( -5.558508435838094286, -2.857531096719115205, 24.36939309276500154 ) ) ;
#10939=DIRECTION ( 'NONE',  ( 0.9510565162951499785, 0.3090169943749582204, 0.000000000000000000 ) ) ;
#10943=CARTESIAN_POINT ( 'NONE',  ( 5.375886393124366336, 2.665038680141326832, 10.99560239355786528 ) ) ;
#10947=CARTESIAN_POINT ( 'NONE',  ( 6.780834053290958173E-14, -6.000000000000000888, 10.49999999999998224 ) ) ;
#10949=CARTESIAN_POINT ( 'NONE',  ( 4.416397290909964468, -4.422724436066375553, 31.26379616840806008 ) ) ;
#10950=B_SPLINE_CURVE_WITH_KNOTS ( 'NONE', 3,
 ( #868, #12959, #15361, #4457, #1903, #11531, #12724, #12652, #13919, #4302, #712, #10348, #9164, #8041, #3107, #3183, #10272, #559 ),
 .UNSPECIFIED., .F., .F.,
 ( 4, 2, 2, 2, 2, 2, 2, 2, 4 ),
 ( 0.003131918686235979094, 0.003523310662250268930, 0.003914702638264559199, 0.004306094614278849035, 0.004697486590293138871, 0.005088878566307429574, 0.005480270542321719410, 0.005871662518336009245, 0.006263054494350299081 ),
 .UNSPECIFIED. ) ;
#10952=CARTESIAN_POINT ( 'NONE',  ( -3.736532060718054993, 4.696070028785918282, 10.52622176056704895 ) ) ;
#10955=EDGE_CURVE ( 'NONE', #11668, #5344, #3196, .T. ) ;
#10956=CARTESIAN_POINT ( 'NONE',  ( 2.094888799673178700E-14, -6.250000000000000888, 30.00000000000000000 ) ) ;
#10958=CARTESIAN_POINT ( 'NONE',  ( -2.817313151351189315, 5.579000502529433803, 5.132374107163055754 ) ) ;
#10962=CARTESIAN_POINT ( 'NONE',  ( 5.558508435838253270, 2.857531096718811892, 17.86762589283693359 ) ) ;
#10967=DIRECTION ( 'NONE',  ( 0.000000000000000000, 1.000000000000000000, 0.000000000000000000 ) ) ;
#10968=CARTESIAN_POINT ( 'NONE',  ( 4.286401442266448036, -4.198423832313277870, 24.49999999999999289 ) ) ;
#10969=EDGE_LOOP ( 'NONE', ( #5288, #7016 ) ) ;
#10972=CARTESIAN_POINT ( 'NONE',  ( 4.322356511625649489, 7.650514973136559149, 5.000000000000004441 ) ) ;
#10973=CARTESIAN_POINT ( 'NONE',  ( 0.8738239080080689725, 6.188820299975588135, 12.00355795710146012 ) ) ;
#10975=CARTESIAN_POINT ( 'NONE',  ( 2.668367453516584220, -5.373994336898154422, 17.99999999999998934 ) ) ;
#10977=CARTESIAN_POINT ( 'NONE',  ( -0.8730424326980719130, -5.936362132114466839, 30.49500690218564358 ) ) ;
#10978=B_SPLINE_CURVE_WITH_KNOTS ( 'NONE', 3,
 ( #8140, #5832, #7978, #12819, #12975, #8297, #14319, #13135, #11783, #10597, #15458, #11552, #1923, #4559, #6796, #11632, #14717, #71 ),
 .UNSPECIFIED., .F., .F.,
 ( 4, 2, 2, 2, 2, 2, 2, 2, 4 ),
 ( 0.000000000000000000, 0.0003914357524127492203, 0.0007828715048254984406, 0.001174307257238247715, 0.001565743009650996014, 0.001957178762063745397, 0.002348614514476494129, 0.002740050266889243729, 0.003131486019301992895 ),
 .UNSPECIFIED. ) ;
#10979=CARTESIAN_POINT ( 'NONE',  ( 5.843318061569068966, -1.367618216965539979, 10.62696220972947003 ) ) ;
#10980=CARTESIAN_POINT ( 'NONE',  ( 6.176542424588149949, -0.9554180641283412934, 24.49999999999999289 ) ) ;
#10981=CARTESIAN_POINT ( 'NONE',  ( -6.155867707731114358, 1.081837891425874831, 10.99563030319846924 ) ) ;
#10983=ORIENTED_EDGE ( 'NONE', *, *, #11076, .F. ) ;
#10984=VERTEX_POINT ( 'NONE', #11986 ) ;
#10985=EDGE_LOOP ( 'NONE', ( #10130, #7995, #2070, #15469 ) ) ;
#10987=CARTESIAN_POINT ( 'NONE',  ( -4.286401442266737583, 4.198423832312984771, 24.49999999999999289 ) ) ;
#10989=EDGE_CURVE ( 'NONE', #8520, #15586, #4330, .T. ) ;
#10997=CARTESIAN_POINT ( 'NONE',  ( 3.632753594129320085, 4.777047695050985254, 5.999950536462231199 ) ) ;
#10999=EDGE_CURVE ( 'NONE', #13850, #10806, #132, .T. ) ;
#11001=CARTESIAN_POINT ( 'NONE',  ( 4.290381260516340056, -4.545736887716145702, 4.384822196241565884 ) ) ;
#11004=EDGE_LOOP ( 'NONE', ( #2865, #13270 ) ) ;
#11005=ORIENTED_EDGE ( 'NONE', *, *, #1450, .F. ) ;
#11006=ORIENTED_EDGE ( 'NONE', *, *, #3939, .F. ) ;
#11008=CARTESIAN_POINT ( 'NONE',  ( 2.996920846510521930, 5.485395142346772168, 4.385580527545153373 ) ) ;
#11010=CARTESIAN_POINT ( 'NONE',  ( 2.692335458626911482, -5.362264153667202216, 11.76239891805595938 ) ) ;
#11012=CARTESIAN_POINT ( 'NONE',  ( -2.668367453516692134, -5.373994336898101132, 11.63236078583908473 ) ) ;
#11013=CARTESIAN_POINT ( 'NONE',  ( -5.648794263291788909, 2.676232015153523935, 5.614419472454846627 ) ) ;
#11014=CARTESIAN_POINT ( 'NONE',  ( -6.020865209844544097, -1.681180471732322435, 23.52599901976669727 ) ) ;
#11020=CARTESIAN_POINT ( 'NONE',  ( 5.843075991566577088, 1.368655265451070413, 10.62635295315575057 ) ) ;
#11023=B_SPLINE_CURVE_WITH_KNOTS ( 'NONE', 3,
 ( #2724, #14822, #9971, #14979, #8704, #2647, #8940, #7653, #9893, #8862, #7423, #14897, #7576, #3984, #334, #12423, #3907, #1523 ),
 .UNSPECIFIED., .F., .F.,
 ( 4, 2, 2, 2, 2, 2, 2, 2, 4 ),
 ( 0.003131486019302005472, 0.003522824630466710009, 0.003914163241631414547, 0.004305501852796119952, 0.004696840463960824490, 0.005088179075125529027, 0.005479517686290232698, 0.005870856297454936368, 0.006262194908619640905 ),
 .UNSPECIFIED. ) ;
#11024=EDGE_LOOP ( 'NONE', ( #5646, #3853, #13559, #4391 ) ) ;
#11026=CARTESIAN_POINT ( 'NONE',  ( -7.490007020835699691, -2.433650805992386701, 31.00000000000000000 ) ) ;
#11027=CARTESIAN_POINT ( 'NONE',  ( 5.783198643800800731, 1.602922020054582397, 25.47377823943293151 ) ) ;
#11028=CARTESIAN_POINT ( 'NONE',  ( 0.2624013748575224625, 5.995472630654511192, 23.52628559691082799 ) ) ;
#11030=CARTESIAN_POINT ( 'NONE',  ( 3.780072143464055401, 4.979057943639872974, 23.49991780678443476 ) ) ;
#11032=CARTESIAN_POINT ( 'NONE',  ( -2.817313151351372724, 5.579000502529338767, 24.49999999999999289 ) ) ;
#11034=CARTESIAN_POINT ( 'NONE',  ( -7.799024015210642702, -1.482594289697281020, 11.49999999999998224 ) ) ;
#11036=DIRECTION ( 'NONE',  ( 0.000000000000000000, 0.000000000000000000, -1.000000000000000000 ) ) ;
#11043=CARTESIAN_POINT ( 'NONE',  ( 5.746619684944315409, 1.730157667110706399, 23.49995067926686687 ) ) ;
#11047=CARTESIAN_POINT ( 'NONE',  ( -2.782713018890741186, -5.315928322779106097, 23.99560239355786351 ) ) ;
#11048=CARTESIAN_POINT ( 'NONE',  ( 2.031800923367348393E-13, -6.250000000000000888, 23.49999999999999289 ) ) ;
#11054=CARTESIAN_POINT ( 'NONE',  ( -0.9999196734182431712, -5.916093360767519016, 30.86725955955067136 ) ) ;
#11055=CARTESIAN_POINT ( 'NONE',  ( 5.665707375537482271, -1.979196487016652961, 10.49992038825522123 ) ) ;
#11057=CARTESIAN_POINT ( 'NONE',  ( -5.935543223013816316, -0.8771126767609508379, 24.49999999999999289 ) ) ;
#11059=ORIENTED_EDGE ( 'NONE', *, *, #15431, .T. ) ;
#11064=CARTESIAN_POINT ( 'NONE',  ( -5.935543223013816316, -0.8771126767609506159, 24.63239388001634111 ) ) ;
#11065=ORIENTED_EDGE ( 'NONE', *, *, #51, .F. ) ;
#11073=CARTESIAN_POINT ( 'NONE',  ( 2.668367453516568677, 5.373994336898162416, 11.49999999999998224 ) ) ;
#11076=EDGE_CURVE ( 'NONE', #8963, #902, #2597, .T. ) ;
#11077=LINE ( 'NONE', #10128, #4033 ) ;
#11079=ORIENTED_EDGE ( 'NONE', *, *, #13770, .F. ) ;
#11082=CARTESIAN_POINT ( 'NONE',  ( -2.668367453516725885, 5.373994336898083368, 31.00000000000000000 ) ) ;
#11084=CARTESIAN_POINT ( 'NONE',  ( -0.6156307853269508135, -5.969051238897255196, 5.798705734106810894 ) ) ;
#11085=EDGE_CURVE ( 'NONE', #14733, #5534, #13526, .T. ) ;
#11086=CARTESIAN_POINT ( 'NONE',  ( -2.668367453516630849, -5.373994336898132218, 5.000000000000004441 ) ) ;
#11088=DIRECTION ( 'NONE',  ( 0.8090169943749421222, 0.5877852522924802425, 0.000000000000000000 ) ) ;
#11089=CARTESIAN_POINT ( 'NONE',  ( -4.267838854167138152, -4.217593933790373839, 11.76239891805595761 ) ) ;
#11091=B_SPLINE_CURVE_WITH_KNOTS ( 'NONE', 3,
 ( #3043, #15374, #4470, #13780, #2887, #7737, #6639, #12666, #497, #5365, #10209, #15062, #7815, #11469, #572, #7896, #9562, #14314 ),
 .UNSPECIFIED., .F., .F.,
 ( 4, 2, 2, 2, 2, 2, 2, 2, 4 ),
 ( 0.000000000000000000, 0.0003914357524127484072, 0.0007828715048254968143, 0.001174307257238245330, 0.001565743009650993629, 0.001957178762063741927, 0.002348614514476490660, 0.002740050266889238959, 0.003131486019301987257 ),
 .UNSPECIFIED. ) ;
#11094=LINE ( 'NONE', #191, #13787 ) ;
#11101=CARTESIAN_POINT ( 'NONE',  ( -3.420659742068370424, 4.931142898501745364, 5.999950536462232087 ) ) ;
#11102=CARTESIAN_POINT ( 'NONE',  ( -6.081464507797602614, 1.446657058464316359, 23.62619944752603374 ) ) ;
#11103=CARTESIAN_POINT ( 'NONE',  ( -2.692693252389773306, 5.362085866495016617, 24.23617396794404044 ) ) ;
#11104=CARTESIAN_POINT ( 'NONE',  ( 6.106056299406742660, 1.336851112280702747, 12.29887838423337953 ) ) ;
#11107=DIRECTION ( 'NONE',  ( -0.9510565162951545304, 0.3090169943749447867, 0.000000000000000000 ) ) ;
#11109=CARTESIAN_POINT ( 'NONE',  ( -2.841519077896339951, 5.566940434249915803, 24.23620383159193636 ) ) ;
#11111=CARTESIAN_POINT ( 'NONE',  ( -6.176542424588110869, 0.9554180641286129649, 11.49999999999998224 ) ) ;
#11117=CARTESIAN_POINT ( 'NONE',  ( -4.435347140101057128, -4.403429997944487084, 11.49999999999998224 ) ) ;
#11118=ORIENTED_EDGE ( 'NONE', *, *, #12425, .F. ) ;
#11124=CARTESIAN_POINT ( 'NONE',  ( 6.780834057763294634E-14, -6.250000000000000888, 10.49999999999998224 ) ) ;
#11127=CARTESIAN_POINT ( 'NONE',  ( 5.984377695197257374, -1.807429553002170897, 12.50004906876531052 ) ) ;
#11129=CYLINDRICAL_SURFACE ( 'NONE', #9864, 0.9999999999999998890 ) ;
#11130=CARTESIAN_POINT ( 'NONE',  ( -0.2623718222034516212, -6.245654667075786648, 10.52627829713833485 ) ) ;
#11131=CARTESIAN_POINT ( 'NONE',  ( 5.903347812666392080, -1.076697810262364552, 25.11397738943081848 ) ) ;
#11134=CARTESIAN_POINT ( 'NONE',  ( 3.735808404765066371, -4.696639218303072738, 5.973980201222398811 ) ) ;
#11136=CARTESIAN_POINT ( 'NONE',  ( -5.903119516422478341, 1.077859910107469288, 10.88480617551147134 ) ) ;
#11137=DIRECTION ( 'NONE',  ( 0.000000000000000000, 1.000000000000000000, 0.000000000000000000 ) ) ;
#11141=ORIENTED_EDGE ( 'NONE', *, *, #14453, .F. ) ;
#11142=EDGE_LOOP ( 'NONE', ( #12330, #3909 ) ) ;
#11143=CARTESIAN_POINT ( 'NONE',  ( -5.842945980534610229, -1.369128644669114658, 25.37378430870261781 ) ) ;
#11144=ORIENTED_EDGE ( 'NONE', *, *, #7017, .T. ) ;
#11149=CARTESIAN_POINT ( 'NONE',  ( 5.131373506000491247, 7.062729720844170167, 17.99999999999998934 ) ) ;
#11151=CARTESIAN_POINT ( 'NONE',  ( -5.903057025253917622, 1.078199533779433450, 31.61561732698606164 ) ) ;
#11152=ADVANCED_FACE ( 'NONE', ( #5392 ), #8899, .F. ) ;
#11155=CARTESIAN_POINT ( 'NONE',  ( -6.172639027853125349, 0.9816353142770998241, 30.73774718278283302 ) ) ;
#11157=EDGE_CURVE ( 'NONE', #5982, #1760, #8983, .T. ) ;
#11160=ORIENTED_EDGE ( 'NONE', *, *, #5363, .F. ) ;
#11161=B_SPLINE_CURVE_WITH_KNOTS ( 'NONE', 3,
 ( #3668, #8773, #13604, #4958, #1357, #2479, #3824, #13530, #8621, #8697, #12023, #7185, #1123, #13456, #7339, #4797, #2637, #1279 ),
 .UNSPECIFIED., .F., .F.,
 ( 4, 2, 2, 2, 2, 2, 2, 2, 4 ),
 ( 0.000000000000000000, 0.0003914357524127512261, 0.0007828715048255024522, 0.001174307257238253570, 0.001565743009651004904, 0.001957178762063754504, 0.002348614514476504538, 0.002740050266889254137, 0.003131486019302004171 ),
 .UNSPECIFIED. ) ;
#11162=CARTESIAN_POINT ( 'NONE',  ( 5.665707375537464507, -1.979196487016696482, 29.99992038825522656 ) ) ;
#11164=EDGE_LOOP ( 'NONE', ( #8153, #14234, #9425, #10733 ) ) ;
#11165=CARTESIAN_POINT ( 'NONE',  ( -5.858813228503601422, -2.179803269293405066, 17.02622717124729945 ) ) ;
#11166=CARTESIAN_POINT ( 'NONE',  ( -2.817313151351126255, -5.579000502529464001, 31.00000000000000000 ) ) ;
#11167=CARTESIAN_POINT ( 'NONE',  ( 0.1323602877612839734, 6.000000000000000888, 12.49999999999998401 ) ) ;
#11170=CARTESIAN_POINT ( 'NONE',  ( -2.931212650151706622, 5.520239928492792991, 10.99574050496989841 ) ) ;
#11171=CARTESIAN_POINT ( 'NONE',  ( -3.255128505894417490, 5.336774832660654333, 18.87380055247395205 ) ) ;
#11180=CARTESIAN_POINT ( 'NONE',  ( -5.558508435838167117, 2.857531096718976205, 17.86936067245787285 ) ) ;
#11181=LINE ( 'NONE', #13561, #13200 ) ;
#11182=CARTESIAN_POINT ( 'NONE',  ( -3.923477796648708882, 4.541042560386316040, 23.62696220972947359 ) ) ;
#11183=DIRECTION ( 'NONE',  ( 0.9510565162951500895, 0.3090169943749582204, 0.000000000000000000 ) ) ;
#11188=CARTESIAN_POINT ( 'NONE',  ( -3.459447313392021162, 5.206669755180872272, 23.52599901976669727 ) ) ;
#11190=CARTESIAN_POINT ( 'NONE',  ( -4.286401442266675410, -4.198423832313046944, 24.49999999999999289 ) ) ;
#11194=DIRECTION ( 'NONE',  ( 0.5877852522924802425, -0.8090169943749422332, 0.000000000000000000 ) ) ;
#11197=CARTESIAN_POINT ( 'NONE',  ( 2.996417732210512330, 5.485687819086936479, 12.11396179408069607 ) ) ;
#11202=ORIENTED_EDGE ( 'NONE', *, *, #2807, .F. ) ;
#11204=CARTESIAN_POINT ( 'NONE',  ( 5.131373506000584506, 7.062729720844102665, 31.00000000000000000 ) ) ;
#11205=CARTESIAN_POINT ( 'NONE',  ( -5.317509234263969375, 2.779225709350972906, 4.869350386511451134 ) ) ;
#11206=CARTESIAN_POINT ( 'NONE',  ( -0.1323408341374213426, -6.250000000000003553, 12.49999999999998401 ) ) ;
#11207=CARTESIAN_POINT ( 'NONE',  ( 3.311576095066468106, 5.004818610361379427, 17.02622176056705783 ) ) ;
#11210=CARTESIAN_POINT ( 'NONE',  ( 2.668367453516705012, -5.373994336898094026, 5.130616955321390726 ) ) ;
#11211=CARTESIAN_POINT ( 'NONE',  ( -2.817313151351206635, 5.579000502529421368, 31.00000000000000000 ) ) ;
#11212=CARTESIAN_POINT ( 'NONE',  ( -5.317509234263900098, -2.779225709351108797, 11.49999999999998224 ) ) ;
#11213=CARTESIAN_POINT ( 'NONE',  ( -5.903057025253897194, -1.078199533779561348, 10.88438267301392948 ) ) ;
#11214=ORIENTED_EDGE ( 'NONE', *, *, #11920, .T. ) ;
#11216=B_SPLINE_CURVE_WITH_KNOTS ( 'NONE', 3,
 ( #5810, #5732, #15515, #4380, #4697, #708, #1025, #6932, #6854, #789, #10736, #1980, #8277, #15596, #2132, #14385, #11834, #944 ),
 .UNSPECIFIED., .F., .F.,
 ( 4, 2, 2, 2, 2, 2, 2, 2, 4 ),
 ( 0.000000000000000000, 0.0003914898357794972241, 0.0007829796715589944483, 0.001174469507338491564, 0.001565959343117988897, 0.001957449178897486229, 0.002348939014676983128, 0.002740428850456480461, 0.003131918686235977793 ),
 .UNSPECIFIED. ) ;
#11218=CARTESIAN_POINT ( 'NONE',  ( -5.620879908643893863, -2.102487719022092527, 23.52622176056705783 ) ) ;
#11221=LINE ( 'NONE', #12568, #467 ) ;
#11222=ORIENTED_EDGE ( 'NONE', *, *, #4548, .F. ) ;
#11224=CARTESIAN_POINT ( 'NONE',  ( -4.070863287254132601, 4.743975846881758329, 4.126941084456993813 ) ) ;
#11226=DIRECTION ( 'NONE',  ( 0.8090169943749421222, 0.5877852522924802425, 0.000000000000000000 ) ) ;
#11230=CARTESIAN_POINT ( 'NONE',  ( 2.782468714962392564, 5.316055268221427710, 5.503897950159861274 ) ) ;
#11232=FACE_OUTER_BOUND ( 'NONE', #15477, .T. ) ;
#11233=CARTESIAN_POINT ( 'NONE',  ( -0.2622538972264072954, 6.245673238944477568, 31.97385994369199125 ) ) ;
#11236=VERTEX_POINT ( 'NONE', #11190 ) ;
#11237=CARTESIAN_POINT ( 'NONE',  ( 0.5042987395409009865, 5.979983180450066271, 18.87329304179975864 ) ) ;
#11239=ORIENTED_EDGE ( 'NONE', *, *, #4466, .F. ) ;
#11240=CARTESIAN_POINT ( 'NONE',  ( -0.1323602877612193029, -6.000000000000001776, 6.000000000000007105 ) ) ;
#11241=EDGE_CURVE ( 'NONE', #8921, #15586, #13569, .T. ) ;
#11242=CARTESIAN_POINT ( 'NONE',  ( 0.6152055445546492640, -5.969096820685154015, 31.79904968670267706 ) ) ;
#11243=CARTESIAN_POINT ( 'NONE',  ( 0.8738118504726281044, 5.936246475285022584, 12.00357242174242423 ) ) ;
#11244=CARTESIAN_POINT ( 'NONE',  ( 0.2637975869347971014, 6.245592211692895468, 18.97332839949193684 ) ) ;
#11246=CYLINDRICAL_SURFACE ( 'NONE', #12436, 0.9999999999999998890 ) ;
#11248=CARTESIAN_POINT ( 'NONE',  ( -5.615811513735041949, 2.743665920700387062, 5.503086438660449886 ) ) ;
#11254=ADVANCED_FACE ( 'NONE', ( #1477 ), #2842, .F. ) ;
#11257=VERTEX_POINT ( 'NONE', #11345 ) ;
#11258=CARTESIAN_POINT ( 'NONE',  ( -3.011139120916522138, 5.190534000030338824, 5.799318062581744648 ) ) ;
#11259=EDGE_CURVE ( 'NONE', #13429, #15355, #10007, .T. ) ;
#11260=LINE ( 'NONE', #7758, #2532 ) ;
#11261=CARTESIAN_POINT ( 'NONE',  ( -0.6151877315909838329, 6.220340188096016298, 5.799066734696703307 ) ) ;
#11262=CARTESIAN_POINT ( 'NONE',  ( 6.155973317223288888, 1.081218830693715161, 12.00308643866043568 ) ) ;
#11264=CARTESIAN_POINT ( 'NONE',  ( 3.736691294293340793, -4.695920479336442632, 23.52641404563306082 ) ) ;
#11266=CARTESIAN_POINT ( 'NONE',  ( -3.883588957979381640, 4.898466244118830915, 23.52622717124730656 ) ) ;
#11268=CARTESIAN_POINT ( 'NONE',  ( -4.344502777243497427, -4.493369211529297580, 30.49610786875029689 ) ) ;
#11270=FACE_BOUND ( 'NONE', #13190, .T. ) ;
#11273=EDGE_CURVE ( 'NONE', #15318, #9802, #7848, .T. ) ;
#11274=CARTESIAN_POINT ( 'NONE',  ( 5.984377695197293789, -1.807429553002048994, 25.50004906876532473 ) ) ;
#11277=CARTESIAN_POINT ( 'NONE',  ( -4.267992336621287741, 4.217442018459910180, 18.26194324003146008 ) ) ;
#11282=EDGE_CURVE ( 'NONE', #278, #11793, #3264, .T. ) ;
#11285=CARTESIAN_POINT ( 'NONE',  ( 3.419318284370122196, 4.932111238568230860, 17.00007997643736957 ) ) ;
#11289=CARTESIAN_POINT ( 'NONE',  ( -4.006441409774732954, 4.467329318258217441, 30.20111757752059489 ) ) ;
#11290=CARTESIAN_POINT ( 'NONE',  ( -5.746837578675981995, -1.729433780394334930, 12.49995053646221166 ) ) ;
#11292=ORIENTED_EDGE ( 'NONE', *, *, #5722, .F. ) ;
#11297=B_SPLINE_CURVE_WITH_KNOTS ( 'NONE', 3,
 ( #11398, #10138, #15065, #14907, #14757, #4160, #5290, #8875, #13547, #12277, #11322, #10213, #6329, #6562, #2891, #9030, #186, #500 ),
 .UNSPECIFIED., .F., .F.,
 ( 4, 2, 2, 2, 2, 2, 2, 2, 4 ),
 ( 0.000000000000000000, 0.0003914362731607615316, 0.0007828725463215230633, 0.001174308819482284541, 0.001565745092643046127, 0.001957181365803807496, 0.002348617638964569081, 0.002740053912125330667, 0.003131490185286092253 ),
 .UNSPECIFIED. ) ;
#11298=ORIENTED_EDGE ( 'NONE', *, *, #5914, .F. ) ;
#11301=ORIENTED_EDGE ( 'NONE', *, *, #10599, .F. ) ;
#11303=CARTESIAN_POINT ( 'NONE',  ( -0.8002302970945222027, 5.947135855825885109, 17.38601773212298696 ) ) ;
#11307=CLOSED_SHELL ( 'NONE', ( #15667, #8641, #8346, #11564, #12013, #3274, #8389, #15606, #1234, #4149, #4585, #9507, #5125, #6831, #6695, #4346, #3000, #2130, #11669, #14662, #5625, #5449, #12885, #7933, #13685, #2109, #12536, #8033, #5559, #5045, #5691, #7397, #6930, #11436, #4436, #3983, #5718, #7951, #14792, #11761, #8725, #14402, #7175, #1697, #14490, #4883, #10668, #8575, #3661, #11735, #12127, #6394, #2042, #1918, #1409, #1366, #14756, #14704, #5172, #4993, #13585, #1399, #13428, #14548, #395, #4377, #11152, #10894, #3955, #6213, #14695, #12225, #14881, #976, #7280, #5036, #2331, #7606, #13387, #11603, #1555, #8182, #6, #9548, #14052, #4934, #6699, #4637, #11254, #253, #5261, #5434, #5457, #14499, #15118, #13006, #10704, #9204, #9219, #2989, #3024, #4103, #4280, #5656, #4144, #4746 ) ) ;
#11309=CARTESIAN_POINT ( 'NONE',  ( 7.799024015210672900, -1.482594289696959944, 17.99999999999998934 ) ) ;
#11311=DIRECTION ( 'NONE',  ( 0.9510565162951500895, 0.3090169943749582204, 0.000000000000000000 ) ) ;
#11312=CARTESIAN_POINT ( 'NONE',  ( 4.267936573529180322, 4.217499624512267786, 11.76229037835932800 ) ) ;
#11314=VERTEX_POINT ( 'NONE', #2103 ) ;
#11316=CARTESIAN_POINT ( 'NONE',  ( 0.5031281619709130348, 5.980084330432656969, 17.12602272744524257 ) ) ;
#11319=EDGE_LOOP ( 'NONE', ( #10227, #1662 ) ) ;
#11320=VECTOR ( 'NONE', #12673, 1000.000000000000000 ) ;
#11321=CARTESIAN_POINT ( 'NONE',  ( -6.176542424588083335, -0.9554180641287667308, 17.99999999999998934 ) ) ;
#11322=CARTESIAN_POINT ( 'NONE',  ( 0.9740856415302261428, -6.173834621338571083, 17.73852653055532969 ) ) ;
#11324=CARTESIAN_POINT ( 'NONE',  ( -2.841041022017402273, 5.567186575787253844, 31.26225281721713145 ) ) ;
#11325=CARTESIAN_POINT ( 'NONE',  ( 0.6156133477427198075, 6.220296490279940471, 18.79872387345518447 ) ) ;
#11327=FACE_OUTER_BOUND ( 'NONE', #7018, .T. ) ;
#11328=CARTESIAN_POINT ( 'NONE',  ( 5.903230462362969000, 1.077253041748798212, 18.61442521571936837 ) ) ;
#11335=ORIENTED_EDGE ( 'NONE', *, *, #4948, .F. ) ;
#11336=CARTESIAN_POINT ( 'NONE',  ( -5.558508435838166228, 2.857531096718976649, 17.99999999999998934 ) ) ;
#11338=CARTESIAN_POINT ( 'NONE',  ( 0.1323736289505031416, -6.249999999999999112, 12.49999999999998579 ) ) ;
#11339=CARTESIAN_POINT ( 'NONE',  ( 6.021135683317699439, 1.680226122398216226, 12.47377282875266502 ) ) ;
#11341=CARTESIAN_POINT ( 'NONE',  ( 2.930922878467498993, 5.520395124723560976, 5.503892131249680908 ) ) ;
#11345=CARTESIAN_POINT ( 'NONE',  ( 2.082642335314403343E-14, -6.000000000000000888, 32.00000000000000000 ) ) ;
#11347=EDGE_CURVE ( 'NONE', #8051, #12191, #15244, .T. ) ;
#11350=CARTESIAN_POINT ( 'NONE',  ( 4.435347140100961205, 4.403429997944583008, 11.49999999999998224 ) ) ;
#11351=CIRCLE ( 'NONE', #14386, 6.000000000000000888 ) ;
#11354=CARTESIAN_POINT ( 'NONE',  ( 6.105747081304200741, -1.338335777572131624, 18.80026515017675592 ) ) ;
#11356=ORIENTED_EDGE ( 'NONE', *, *, #2610, .F. ) ;
#11357=CARTESIAN_POINT ( 'NONE',  ( -4.435347140101107755, -4.403429997944435570, 17.86936067245787996 ) ) ;
#11358=FACE_OUTER_BOUND ( 'NONE', #9602, .T. ) ;
#11362=CARTESIAN_POINT ( 'NONE',  ( -5.940390500375766436, 6.474944468551470322, 17.99999999999998934 ) ) ;
#11364=CARTESIAN_POINT ( 'NONE',  ( 5.649053410273073617, -2.675685104943254178, 5.615177803758428787 ) ) ;
#11367=ORIENTED_EDGE ( 'NONE', *, *, #12836, .T. ) ;
#11370=EDGE_CURVE ( 'NONE', #1119, #8460, #12845, .T. ) ;
#11376=ORIENTED_EDGE ( 'NONE', *, *, #10220, .T. ) ;
#11378=CARTESIAN_POINT ( 'NONE',  ( -0.6139908388539705442, 5.969238533166628002, 17.19977627912012252 ) ) ;
#11379=AXIS2_PLACEMENT_3D ( 'NONE', #6084, #3526, #8396 ) ;
#11382=CARTESIAN_POINT ( 'NONE',  ( 0.2619456584323444082, -5.995505046955608819, 17.02607193928646012 ) ) ;
#11383=CYLINDRICAL_SURFACE ( 'NONE', #4920, 1.000000000000000000 ) ;
#11390=EDGE_LOOP ( 'NONE', ( #8113, #13697 ) ) ;
#11392=ORIENTED_EDGE ( 'NONE', *, *, #15078, .F. ) ;
#11394=CARTESIAN_POINT ( 'NONE',  ( 2.848727059635939973, -5.281416301279907799, 25.11442521571938613 ) ) ;
#11397=CARTESIAN_POINT ( 'NONE',  ( -6.020865209844566301, -1.681180471732242943, 17.02599901976669017 ) ) ;
#11398=CARTESIAN_POINT ( 'NONE',  ( 1.353717517954364224E-13, -6.250000000000000888, 18.99999999999998934 ) ) ;
#11399=CARTESIAN_POINT ( 'NONE',  ( -4.416837305303518590, 4.422286678978986529, 31.26190213084010239 ) ) ;
#11400=CARTESIAN_POINT ( 'NONE',  ( 0.7988860301923814689, 6.199427171881318088, 17.38455580536196265 ) ) ;
#11403=CARTESIAN_POINT ( 'NONE',  ( -3.567624405365413143, 5.133384272590665098, 18.99995078984292363 ) ) ;
#11408=ORIENTED_EDGE ( 'NONE', *, *, #6498, .T. ) ;
#11411=CARTESIAN_POINT ( 'NONE',  ( 3.158296126777914825, -5.394094919772040697, 5.798878384233398187 ) ) ;
#11412=CARTESIAN_POINT ( 'NONE',  ( 2.817313151351127587, -5.579000502529462224, 11.49999999999998224 ) ) ;
#11414=CARTESIAN_POINT ( 'NONE',  ( -0.2619041840694833478, 6.245686665308502583, 4.026058494337954485 ) ) ;
#11415=CARTESIAN_POINT ( 'NONE',  ( 5.858736126997126981, 2.179962889277081040, 30.02640428276699325 ) ) ;
#11417=CARTESIAN_POINT ( 'NONE',  ( 4.286401442266448925, -4.198423832313278758, 24.36760611998364467 ) ) ;
#11427=CARTESIAN_POINT ( 'NONE',  ( 2.840966774240165194, 5.567223638426907151, 11.76190213084010239 ) ) ;
#11430=CARTESIAN_POINT ( 'NONE',  ( 6.176542424588141955, -0.9554180641284083508, 18.13063932754212004 ) ) ;
#11432=VERTEX_POINT ( 'NONE', #4500 ) ;
#11433=CARTESIAN_POINT ( 'NONE',  ( -2.668367453516752974, -5.373994336898072710, 17.99999999999998934 ) ) ;
#11435=CARTESIAN_POINT ( 'NONE',  ( 5.935543223013879377, -0.8771126767605279539, 17.99999999999998934 ) ) ;
#11436=ADVANCED_FACE ( 'NONE', ( #4584 ), #5778, .F. ) ;
#11439=CARTESIAN_POINT ( 'NONE',  ( 4.322356511625485176, 7.650514973136679941, 24.49999999999999289 ) ) ;
#11440=CARTESIAN_POINT ( 'NONE',  ( -5.935543223013847403, -0.8771126767607488883, 5.132393880016354437 ) ) ;
#11441=CARTESIAN_POINT ( 'NONE',  ( 3.633127580202335505, -4.776802569231014317, 6.000079611744768115 ) ) ;
#11442=CARTESIAN_POINT ( 'NONE',  ( 6.176542424588118863, -0.9554180641285446862, 5.000000000000004441 ) ) ;
#11443=CARTESIAN_POINT ( 'NONE',  ( -5.940390500375711369, 6.474944468551510290, 11.49999999999998224 ) ) ;
#11445=ORIENTED_EDGE ( 'NONE', *, *, #8740, .T. ) ;
#11447=ORIENTED_EDGE ( 'NONE', *, *, #5811, .T. ) ;
#11448=CARTESIAN_POINT ( 'NONE',  ( -5.866923913994616768, 1.260079467906669137, 25.29952054102715664 ) ) ;
#11449=ORIENTED_EDGE ( 'NONE', *, *, #9889, .F. ) ;
#11450=DIRECTION ( 'NONE',  ( 0.000000000000000000, 0.000000000000000000, 1.000000000000000000 ) ) ;
#11455=CARTESIAN_POINT ( 'NONE',  ( -0.7993282387949770529, 5.947240459526529577, 18.61484358216956991 ) ) ;
#11456=CARTESIAN_POINT ( 'NONE',  ( -4.070863287254068652, -4.743975846881813396, 5.873058915543009739 ) ) ;
#11458=CARTESIAN_POINT ( 'NONE',  ( -6.105925084677690684, -1.337450587213149467, 5.799331489075775004 ) ) ;
#11466=ORIENTED_EDGE ( 'NONE', *, *, #11347, .F. ) ;
#11468=CARTESIAN_POINT ( 'NONE',  ( 4.435347140101025154, -4.403429997944519059, 11.49999999999998224 ) ) ;
#11469=CARTESIAN_POINT ( 'NONE',  ( 6.143143148203035864, 1.154591847827815654, 4.386038205919295940 ) ) ;
#11472=CARTESIAN_POINT ( 'NONE',  ( -0.8002720181889466655, 6.199262377003425861, 17.38606262465554053 ) ) ;
#11473=CARTESIAN_POINT ( 'NONE',  ( -6.176542424588083335, -0.9554180641287667308, 17.99999999999998934 ) ) ;
#11477=CARTESIAN_POINT ( 'NONE',  ( 2.668367453516568677, 5.373994336898162416, 11.49999999999998224 ) ) ;
#11479=VECTOR ( 'NONE', #9826, 1000.000000000000114 ) ;
#11484=EDGE_LOOP ( 'NONE', ( #13124, #2069, #12503, #3326 ) ) ;
#11485=CARTESIAN_POINT ( 'NONE',  ( 3.107278289587274589, -5.134157760521997460, 4.126352953155772774 ) ) ;
#11487=CARTESIAN_POINT ( 'NONE',  ( -2.817313151351311884, 5.579000502529370742, 17.99999999999998934 ) ) ;
#11489=LINE ( 'NONE', #13954, #1173 ) ;
#11492=DIRECTION ( 'NONE',  ( -0.9510565162951545304, 0.3090169943749447867, 0.000000000000000000 ) ) ;
#11494=CARTESIAN_POINT ( 'NONE',  ( 4.435347140100977192, -4.403429997944567020, 17.99999999999998934 ) ) ;
#11497=CARTESIAN_POINT ( 'NONE',  ( 5.867109477881220059, 1.259218163101030186, 5.798882422479413101 ) ) ;
#11501=CARTESIAN_POINT ( 'NONE',  ( 0.000000000000000000, 0.000000000000000000, 36.00000000000000711 ) ) ;
#11503=CARTESIAN_POINT ( 'NONE',  ( 6.176542424588121527, -0.9554180641285241471, 30.86939309276501575 ) ) ;
#11506=CARTESIAN_POINT ( 'NONE',  ( 4.435347140100929231, -4.403429997944614982, 24.63234125634167526 ) ) ;
#11508=ORIENTED_EDGE ( 'NONE', *, *, #14007, .F. ) ;
#11509=CARTESIAN_POINT ( 'NONE',  ( -2.817313151351230172, -5.579000502529412486, 17.99999999999998934 ) ) ;
#11510=CARTESIAN_POINT ( 'NONE',  ( 2.692143549875217978, 5.362363179736568952, 24.76194324003146008 ) ) ;
#11512=CARTESIAN_POINT ( 'NONE',  ( -5.903119516422490776, 1.077859910107415331, 4.384806175511481996 ) ) ;
#11513=DIRECTION ( 'NONE',  ( 0.000000000000000000, 0.000000000000000000, 1.000000000000000000 ) ) ;
#11515=CARTESIAN_POINT ( 'NONE',  ( 2.082642335314403343E-14, -6.250000000000000888, 32.00000000000000000 ) ) ;
#11516=CARTESIAN_POINT ( 'NONE',  ( -5.375763363753442547, -2.665284979407549049, 5.503897950159861274 ) ) ;
#11518=CARTESIAN_POINT ( 'NONE',  ( 5.770288754215199489, -2.404361317819788901, 23.62618035954928786 ) ) ;
#11519=CARTESIAN_POINT ( 'NONE',  ( -6.105925084677707559, 1.337450587213069753, 4.200668510924230326 ) ) ;
#11520=CARTESIAN_POINT ( 'NONE',  ( -5.842988226680550845, -1.369004370660760861, 10.62619317285287934 ) ) ;
#11521=EDGE_LOOP ( 'NONE', ( #7336, #12954 ) ) ;
#11524=EDGE_CURVE ( 'NONE', #11793, #2012, #14744, .T. ) ;
#11525=ORIENTED_EDGE ( 'NONE', *, *, #13524, .F. ) ;
#11526=CARTESIAN_POINT ( 'NONE',  ( 4.286401442266518202, 4.198423832313208592, 31.00000000000000000 ) ) ;
#11527=ORIENTED_EDGE ( 'NONE', *, *, #13420, .T. ) ;
#11528=FACE_OUTER_BOUND ( 'NONE', #8577, .T. ) ;
#11529=CARTESIAN_POINT ( 'NONE',  ( -5.330004929009570347, -2.755647751839434445, 30.73760108194403173 ) ) ;
#11531=CARTESIAN_POINT ( 'NONE',  ( 5.867109477881279567, -1.259218163100750854, 23.70111757752058068 ) ) ;
#11533=CARTESIAN_POINT ( 'NONE',  ( 0.5039079366033875074, -5.980031194523140137, 17.12637068109812333 ) ) ;
#11536=CARTESIAN_POINT ( 'NONE',  ( -5.915641100987802048, -1.003868594704925510, 17.49571079637980020 ) ) ;
#11539=EDGE_CURVE ( 'NONE', #12035, #727, #817, .T. ) ;
#11541=ORIENTED_EDGE ( 'NONE', *, *, #12054, .F. ) ;
#11542=ORIENTED_EDGE ( 'NONE', *, *, #13770, .T. ) ;
#11543=CARTESIAN_POINT ( 'NONE',  ( 2.782156709077311163, -5.316215864844103578, 25.00312048902378237 ) ) ;
#11546=VERTEX_POINT ( 'NONE', #7574 ) ;
#11547=CARTESIAN_POINT ( 'NONE',  ( 5.531796221294931648, -2.326749136277085128, 18.87378430870261781 ) ) ;
#11548=B_SPLINE_CURVE_WITH_KNOTS ( 'NONE', 3,
 ( #15479, #13240, #11878, #4279, #1066, #11801, #15718, #4737, #9144, #5930, #1803, #10777, #5852, #15635, #8317, #15557, #2173, #4657 ),
 .UNSPECIFIED., .F., .F.,
 ( 4, 2, 2, 2, 2, 2, 2, 2, 4 ),
 ( 0.003131490185286087483, 0.003522829482338687979, 0.003914168779391288475, 0.004305508076443888971, 0.004696847373496489467, 0.005088186670549089963, 0.005479525967601690459, 0.005870865264654290955, 0.006262204561706891451 ),
 .UNSPECIFIED. ) ;
#11552=CARTESIAN_POINT ( 'NONE',  ( 3.254737477227823472, 5.337033878705316425, 25.37367328635992081 ) ) ;
#11555=EDGE_CURVE ( 'NONE', #5302, #4447, #5198, .T. ) ;
#11560=CYLINDRICAL_SURFACE ( 'NONE', #2666, 0.9999999999999998890 ) ;
#11564=ADVANCED_FACE ( 'NONE', ( #20 ), #9891, .F. ) ;
#11565=ORIENTED_EDGE ( 'NONE', *, *, #13222, .F. ) ;
#11568=CARTESIAN_POINT ( 'NONE',  ( 5.984377695197266256, 1.807429553002144917, 23.49995093123466461 ) ) ;
#11569=CARTESIAN_POINT ( 'NONE',  ( -5.329907877631334223, 2.755840666746301348, 17.73805675996853637 ) ) ;
#11570=FACE_BOUND ( 'NONE', #14731, .T. ) ;
#11571=CARTESIAN_POINT ( 'NONE',  ( 6.105747081304183865, -1.338335777572222440, 31.80026515017675592 ) ) ;
#11572=VECTOR ( 'NONE', #9523, 1000.000000000000114 ) ;
#11580=DIRECTION ( 'NONE',  ( 0.000000000000000000, 0.000000000000000000, 1.000000000000000000 ) ) ;
#11581=CARTESIAN_POINT ( 'NONE',  ( 0.9999171162591851125, 6.169494774098513545, 24.36722320330680347 ) ) ;
#11584=CARTESIAN_POINT ( 'NONE',  ( -2.817313151351373168, 5.579000502529340544, 24.63237410716306286 ) ) ;
#11585=EDGE_CURVE ( 'NONE', #8963, #12601, #8036, .T. ) ;
#11586=CARTESIAN_POINT ( 'NONE',  ( 2.030576276931546336E-13, -6.000000000000000888, 25.49999999999999645 ) ) ;
#11588=DIRECTION ( 'NONE',  ( 0.8090169943749506709, -0.5877852522924689183, 0.000000000000000000 ) ) ;
#11593=CARTESIAN_POINT ( 'NONE',  ( -0.1323933160975409862, 6.000000000000000000, 32.00000000000000000 ) ) ;
#11594=VECTOR ( 'NONE', #14958, 1000.000000000000114 ) ;
#11597=CARTESIAN_POINT ( 'NONE',  ( -6.172639027853131566, 0.9816353142770681828, 4.737747182782872990 ) ) ;
#11598=CARTESIAN_POINT ( 'NONE',  ( -2.668367453516648169, -5.373994336898123336, 31.00000000000000000 ) ) ;
#11602=CARTESIAN_POINT ( 'NONE',  ( 6.780834062235653815E-14, 6.000000000000000888, 10.49999999999998224 ) ) ;
#11603=ADVANCED_FACE ( 'NONE', ( #15131 ), #4306, .F. ) ;
#11606=CYLINDRICAL_SURFACE ( 'NONE', #6349, 1.000000000000000666 ) ;
#11608=CARTESIAN_POINT ( 'NONE',  ( -5.620879908643956924, -2.102487719021920221, 30.02622176056706138 ) ) ;
#11610=CARTESIAN_POINT ( 'NONE',  ( 3.253823204785017964, 5.337590213880564427, 17.12694108445698404 ) ) ;
#11612=CARTESIAN_POINT ( 'NONE',  ( 7.490007020835686369, -2.433650805992243260, 5.000000000000004441 ) ) ;
#11619=CYLINDRICAL_SURFACE ( 'NONE', #4404, 1.000000000000000888 ) ;
#11621=EDGE_LOOP ( 'NONE', ( #12348, #15192 ) ) ;
#11622=ORIENTED_EDGE ( 'NONE', *, *, #2090, .F. ) ;
#11623=ORIENTED_EDGE ( 'NONE', *, *, #8439, .T. ) ;
#11624=CARTESIAN_POINT ( 'NONE',  ( 3.780072143464169976, -4.979057943639785933, 19.00008219321555814 ) ) ;
#11625=CYLINDRICAL_SURFACE ( 'NONE', #12400, 1.000000000000000000 ) ;
#11626=ORIENTED_EDGE ( 'NONE', *, *, #11524, .F. ) ;
#11627=AXIS2_PLACEMENT_3D ( 'NONE', #14070, #15358, #7958 ) ;
#11629=AXIS2_PLACEMENT_3D ( 'NONE', #11695, #795, #5661 ) ;
#11631=CARTESIAN_POINT ( 'NONE',  ( -0.8737888311108027439, 5.936248257219539859, 25.00344185141216613 ) ) ;
#11632=CARTESIAN_POINT ( 'NONE',  ( 2.840966774240040404, 5.567223638426967547, 24.76190213084013081 ) ) ;
#11634=DIRECTION ( 'NONE',  ( 0.5877852522924802425, -0.8090169943749422332, 0.000000000000000000 ) ) ;
#11638=CARTESIAN_POINT ( 'NONE',  ( -5.409007216690671527, -2.598315788643751123, 4.385574784280630745 ) ) ;
#11641=AXIS2_PLACEMENT_3D ( 'NONE', #14885, #6229, #3972 ) ;
#11644=EDGE_LOOP ( 'NONE', ( #9953, #10517 ) ) ;
#11645=CARTESIAN_POINT ( 'NONE',  ( -3.567258970016075725, 5.133675764669605179, 16.99991780678442410 ) ) ;
#11646=EDGE_CURVE ( 'NONE', #3666, #8289, #6550, .T. ) ;
#11648=CARTESIAN_POINT ( 'NONE',  ( -0.2619456584322020221, 5.995505046955617701, 4.026071939286482326 ) ) ;
#11650=CARTESIAN_POINT ( 'NONE',  ( 4.435347140100961205, 4.403429997944583008, 11.36765874365829099 ) ) ;
#11654=CARTESIAN_POINT ( 'NONE',  ( 3.633127580202256457, 4.776802569231072049, 3.999920388255240322 ) ) ;
#11659=B_SPLINE_CURVE_WITH_KNOTS ( 'NONE', 3,
 ( #6143, #15683, #13210, #1033, #8451, #13286, #7252, #1189, #8533, #7092, #2222, #10906, #3, #4946, #2467, #4866, #9724, #7330 ),
 .UNSPECIFIED., .F., .F.,
 ( 4, 2, 2, 2, 2, 2, 2, 2, 4 ),
 ( 0.000000000000000000, 0.0003914898357794964652, 0.0007829796715589929304, 0.001174469507338489396, 0.001565959343117985861, 0.001957449178897482326, 0.002348939014676978791, 0.002740428850456475256, 0.003131918686235971722 ),
 .UNSPECIFIED. ) ;
#11662=CARTESIAN_POINT ( 'NONE',  ( 0.9740012993921920437, 6.173846968979613159, 24.76164920628449906 ) ) ;
#11667=CARTESIAN_POINT ( 'NONE',  ( -0.8730424326978892813, -5.936362132114493484, 23.99500690218563292 ) ) ;
#11668=VERTEX_POINT ( 'NONE', #9019 ) ;
#11669=ADVANCED_FACE ( 'NONE', ( #13923 ), #14003, .F. ) ;
#11672=DIRECTION ( 'NONE',  ( 0.9510565162951499785, 0.3090169943749582204, 0.000000000000000000 ) ) ;
#11679=CARTESIAN_POINT ( 'NONE',  ( -0.8736516769106569269, 5.936271176698238783, 30.49606771578675080 ) ) ;
#11681=FACE_BOUND ( 'NONE', #3528, .T. ) ;
#11686=CARTESIAN_POINT ( 'NONE',  ( 1.354942165200771727E-13, 6.000000000000000888, 16.99999999999998579 ) ) ;
#11688=EDGE_LOOP ( 'NONE', ( #2018, #9400, #15352, #7793 ) ) ;
#11689=CARTESIAN_POINT ( 'NONE',  ( -4.286401442266531525, -4.198423832313195270, 5.000000000000004441 ) ) ;
#11691=CARTESIAN_POINT ( 'NONE',  ( 5.409274167810672829, 2.597759609440601913, 17.38480617551147844 ) ) ;
#11693=CARTESIAN_POINT ( 'NONE',  ( 2.031800924094035195E-13, 6.250000000000000888, 23.49999999999999289 ) ) ;
#11695=CARTESIAN_POINT ( 'NONE',  ( 2.082642335314403343E-14, -6.250000000000000888, 31.00000000000000000 ) ) ;
#11699=CARTESIAN_POINT ( 'NONE',  ( 5.131373506000491247, 7.062729720844170167, 17.99999999999998934 ) ) ;
#11702=ORIENTED_EDGE ( 'NONE', *, *, #5743, .T. ) ;
#11703=CARTESIAN_POINT ( 'NONE',  ( 2.692335458626790690, -5.362264153667266164, 24.76239891805597537 ) ) ;
#11704=CARTESIAN_POINT ( 'NONE',  ( -6.250000000000000888, 0.000000000000000000, 53.67766952966368876 ) ) ;
#11708=CARTESIAN_POINT ( 'NONE',  ( 0.7993282387951129442, -5.947240459526509149, 5.614843582169577019 ) ) ;
#11709=CARTESIAN_POINT ( 'NONE',  ( -4.070051655338043695, -4.744673454622527764, 4.126326713640078303 ) ) ;
#11712=FACE_OUTER_BOUND ( 'NONE', #7731, .T. ) ;
#11717=FACE_OUTER_BOUND ( 'NONE', #806, .T. ) ;
#11720=ORIENTED_EDGE ( 'NONE', *, *, #1525, .T. ) ;
#11722=CARTESIAN_POINT ( 'NONE',  ( -0.9999505860952755398, 6.169489349035817582, 11.63105903165808108 ) ) ;
#11723=CYLINDRICAL_SURFACE ( 'NONE', #6361, 1.000000000000000222 ) ;
#11724=CARTESIAN_POINT ( 'NONE',  ( -0.1323933160975646617, 6.000000000000000000, 6.000000000000003553 ) ) ;
#11725=ORIENTED_EDGE ( 'NONE', *, *, #1525, .F. ) ;
#11726=CARTESIAN_POINT ( 'NONE',  ( -5.935543223013841185, 0.8771126767608004027, 17.99999999999998934 ) ) ;
#11728=CARTESIAN_POINT ( 'NONE',  ( 3.883716939929057421, -4.898343590941192538, 17.02640428276698259 ) ) ;
#11730=CARTESIAN_POINT ( 'NONE',  ( -3.159082487394891281, -5.393634094348267460, 25.29954462468842635 ) ) ;
#11731=SURFACE_STYLE_FILL_AREA ( #8084 ) ;
#11735=ADVANCED_FACE ( 'NONE', ( #1909 ), #5587, .F. ) ;
#11737=CARTESIAN_POINT ( 'NONE',  ( 7.180990026460747799, -3.384707322287378695, 31.00000000000000000 ) ) ;
#11738=CARTESIAN_POINT ( 'NONE',  ( -5.782947755040646953, 1.603807858344055370, 18.97398020122238194 ) ) ;
#11741=VECTOR ( 'NONE', #3863, 1000.000000000000114 ) ;
#11743=CARTESIAN_POINT ( 'NONE',  ( -3.567624405365465101, 5.133384272590623354, 25.49995078984292007 ) ) ;
#11744=CARTESIAN_POINT ( 'NONE',  ( 2.031800923283433283E-13, -6.000000000000000888, 23.49999999999999289 ) ) ;
#11745=VERTEX_POINT ( 'NONE', #12805 ) ;
#11746=CARTESIAN_POINT ( 'NONE',  ( -5.769755079862278535, 2.405651898699073588, 18.87305891554299464 ) ) ;
#11747=VERTEX_POINT ( 'NONE', #6782 ) ;
#11748=DIRECTION ( 'NONE',  ( 0.5877852522924802425, -0.8090169943749422332, 0.000000000000000000 ) ) ;
#11752=CARTESIAN_POINT ( 'NONE',  ( -5.531623157106165145, -2.327208526676436851, 5.873647046844243214 ) ) ;
#11754=CARTESIAN_POINT ( 'NONE',  ( 6.020822430078789367, 1.681351817312415564, 10.52591457665827335 ) ) ;
#11755=FACE_OUTER_BOUND ( 'NONE', #9897, .T. ) ;
#11759=CARTESIAN_POINT ( 'NONE',  ( 3.735808404764985546, 4.696639218303137575, 30.02601979877761451 ) ) ;
#11760=EDGE_LOOP ( 'NONE', ( #7566, #4987, #11141, #11626 ) ) ;
#11761=ADVANCED_FACE ( 'NONE', ( #7807 ), #717, .F. ) ;
#11764=CARTESIAN_POINT ( 'NONE',  ( 2.930600586412840602, 5.520563544161817937, 17.49691356133953946 ) ) ;
#11766=CARTESIAN_POINT ( 'NONE',  ( -3.567258970015892761, -5.133675764669733965, 6.000082193215567905 ) ) ;
#11768=CARTESIAN_POINT ( 'NONE',  ( 2.692143549875417374, -5.362363179736472141, 11.23805675996853104 ) ) ;
#11770=CARTESIAN_POINT ( 'NONE',  ( 2.082642335314403343E-14, -6.250000000000000888, 32.00000000000000000 ) ) ;
#11773=LINE ( 'NONE', #14308, #1599 ) ;
#11774=EDGE_LOOP ( 'NONE', ( #11447, #641, #7897, #821 ) ) ;
#11776=ORIENTED_EDGE ( 'NONE', *, *, #14856, .F. ) ;
#11779=VERTEX_POINT ( 'NONE', #12578 ) ;
#11782=CARTESIAN_POINT ( 'NONE',  ( 0.6152055445546467105, -5.969096820685153126, 5.799049686702669071 ) ) ;
#11783=CARTESIAN_POINT ( 'NONE',  ( 3.779681992289640302, 4.979315417304017721, 25.49995078984292718 ) ) ;
#11786=AXIS2_PLACEMENT_3D ( 'NONE', #758, #13001, #10626 ) ;
#11787=CARTESIAN_POINT ( 'NONE',  ( 6.176542424588118863, -0.9554180641285446862, 4.869393092765015751 ) ) ;
#11790=CARTESIAN_POINT ( 'NONE',  ( -5.531209434046327367, -2.328189801702647443, 4.126962209729496678 ) ) ;
#11792=CARTESIAN_POINT ( 'NONE',  ( 4.290381260516173967, 4.545736887716300245, 18.61517780375843145 ) ) ;
#11793=VERTEX_POINT ( 'NONE', #9316 ) ;
#11795=CARTESIAN_POINT ( 'NONE',  ( 0.6156133477426980471, 6.220296490279942248, 31.79872387345512053 ) ) ;
#11796=EDGE_CURVE ( 'NONE', #12482, #8538, #11842, .T. ) ;
#11797=CARTESIAN_POINT ( 'NONE',  ( 6.176542424588149949, -0.9554180641283412934, 24.49999999999999289 ) ) ;
#11798=CARTESIAN_POINT ( 'NONE',  ( 6.768587589771821120E-14, -6.250000000000000888, 12.49999999999998401 ) ) ;
#11800=CARTESIAN_POINT ( 'NONE',  ( 2.996920846510460201, 5.485395142346805031, 10.88558052754513383 ) ) ;
#11801=CARTESIAN_POINT ( 'NONE',  ( -0.7988860301922200424, -6.199427171881335852, 4.384555805361945779 ) ) ;
#11802=FACE_BOUND ( 'NONE', #11319, .T. ) ;
#11805=CARTESIAN_POINT ( 'NONE',  ( -2.931212650151761245, -5.520239928492765458, 25.00425949503010514 ) ) ;
#11806=CARTESIAN_POINT ( 'NONE',  ( 5.487097279078403389, 2.429065649168880014, 5.799520541027148646 ) ) ;
#11810=CARTESIAN_POINT ( 'NONE',  ( 5.665824935993602374, 1.978765057080938528, 10.50004946353775281 ) ) ;
#11813=CARTESIAN_POINT ( 'NONE',  ( 3.158296126777728752, -5.394094919772149055, 25.29887838423338309 ) ) ;
#11815=ORIENTED_EDGE ( 'NONE', *, *, #11085, .F. ) ;
#11817=DIRECTION ( 'NONE',  ( 0.8090169943749421222, 0.5877852522924802425, 0.000000000000000000 ) ) ;
#11819=EDGE_CURVE ( 'NONE', #7314, #1678, #3259, .T. ) ;
#11822=CARTESIAN_POINT ( 'NONE',  ( -4.152999119457993160, 4.671604476854340326, 5.800265150176763918 ) ) ;
#11825=FACE_BOUND ( 'NONE', #1309, .T. ) ;
#11826=CARTESIAN_POINT ( 'NONE',  ( -5.648559266344554075, 2.676764518775872848, 4.386038205919296828 ) ) ;
#11827=CARTESIAN_POINT ( 'NONE',  ( -2.849269941561927588, -5.281123252784065691, 30.38480617551148910 ) ) ;
#11831=VERTEX_POINT ( 'NONE', #3338 ) ;
#11833=B_SPLINE_CURVE_WITH_KNOTS ( 'NONE', 3,
 ( #13068, #8311, #15627, #9502, #13149, #7200, #2251, #2328, #9422, #15473, #4893, #1138, #9581, #11795, #12041, #4650, #14508, #982 ),
 .UNSPECIFIED., .F., .F.,
 ( 4, 2, 2, 2, 2, 2, 2, 2, 4 ),
 ( 0.003131490185286055824, 0.003522829482338662825, 0.003914168779391269393, 0.004305508076443876828, 0.004696847373496483395, 0.005088186670549079554, 0.005479525967601676581, 0.005870865264654273608, 0.006262204561706869767 ),
 .UNSPECIFIED. ) ;
#11834=CARTESIAN_POINT ( 'NONE',  ( -4.286401442266607908, 4.198423832313116222, 31.13064961348856130 ) ) ;
#11836=CARTESIAN_POINT ( 'NONE',  ( 0.5030929395821142069, 6.230885867001139999, 10.62600319116548597 ) ) ;
#11838=CARTESIAN_POINT ( 'NONE',  ( 3.736691294293485566, -4.695920479336326281, 30.02641404563305372 ) ) ;
#11842=LINE ( 'NONE', #13119, #10794 ) ;
#11848=CARTESIAN_POINT ( 'NONE',  ( 4.267558728637114385, -4.217879122113883383, 24.76382603205594179 ) ) ;
#11850=ORIENTED_EDGE ( 'NONE', *, *, #12219, .F. ) ;
#11854=CARTESIAN_POINT ( 'NONE',  ( -0.6139908388538884987, 5.969238533166634220, 23.69977627912011897 ) ) ;
#11858=CARTESIAN_POINT ( 'NONE',  ( 5.985119669071112369, -1.805077827356573517, 4.000082581897114409 ) ) ;
#11859=SHAPE_DEFINITION_REPRESENTATION ( #10829, #9569 ) ;
#11861=EDGE_CURVE ( 'NONE', #5534, #14733, #3664, .T. ) ;
#11862=B_SPLINE_CURVE_WITH_KNOTS ( 'NONE', 3,
 ( #1617, #425, #9183, #10372, #11328, #15150, #4243, #9112, #14997, #13941, #3052, #12745, #1849, #3279, #3204, #12822, #14247, #5835 ),
 .UNSPECIFIED., .F., .F.,
 ( 4, 2, 2, 2, 2, 2, 2, 2, 4 ),
 ( 0.003131918686235958711, 0.003523310662250251149, 0.003914702638264542719, 0.004306094614278835157, 0.004697486590293127595, 0.005088878566307419166, 0.005480270542321710736, 0.005871662518336002307, 0.006263054494350293877 ),
 .UNSPECIFIED. ) ;
#11865=CARTESIAN_POINT ( 'NONE',  ( 2.840966774240103465, 5.567223638426939125, 18.26190213084012015 ) ) ;
#11867=CARTESIAN_POINT ( 'NONE',  ( -5.665308849928780255, 1.980336949702632632, 25.49992002356261622 ) ) ;
#11868=CARTESIAN_POINT ( 'NONE',  ( 4.416397290909769069, 4.422724436066569176, 24.23620383159193636 ) ) ;
#11871=CARTESIAN_POINT ( 'NONE',  ( -5.648794263291742723, -2.676232015153619415, 30.38558052754516225 ) ) ;
#11875=VERTEX_POINT ( 'NONE', #15522 ) ;
#11876=CARTESIAN_POINT ( 'NONE',  ( -5.984759433607027113, 1.806271833852240105, 32.00008219321556169 ) ) ;
#11878=CARTESIAN_POINT ( 'NONE',  ( -0.2623718222035099079, -6.245654667075784872, 4.026278297138354390 ) ) ;
#11879=CARTESIAN_POINT ( 'NONE',  ( -0.6144300524831621813, -6.220417338033072951, 23.70033372175933550 ) ) ;
#11883=AXIS2_PLACEMENT_3D ( 'NONE', #7317, #10967, #1255 ) ;
#11888=CARTESIAN_POINT ( 'NONE',  ( 5.531796221294864147, 2.326749136277247221, 10.62621569129737331 ) ) ;
#11890=ORIENTED_EDGE ( 'NONE', *, *, #4392, .F. ) ;
#11894=CARTESIAN_POINT ( 'NONE',  ( -0.5042987395405625906, -5.979983180450094693, 25.37329304179976930 ) ) ;
#11898=B_SPLINE_CURVE_WITH_KNOTS ( 'NONE', 3,
 ( #10310, #11417, #4104, #10003, #518, #10077, #4180, #11264, #2912, #7684, #12532, #8974, #14850, #365, #13877, #9051, #7762, #7843 ),
 .UNSPECIFIED., .F., .F.,
 ( 4, 2, 2, 2, 2, 2, 2, 2, 4 ),
 ( 0.000000000000000000, 0.0003914898357794980915, 0.0007829796715589961830, 0.001174469507338494166, 0.001565959343117991282, 0.001957449178897488831, 0.002348939014676985730, 0.002740428850456482629, 0.003131918686235979962 ),
 .UNSPECIFIED. ) ;
#11899=CARTESIAN_POINT ( 'NONE',  ( -5.131373506000878493, 7.062729720843910819, 24.49999999999999289 ) ) ;
#11903=CARTESIAN_POINT ( 'NONE',  ( 5.616116467183688954, 2.743044348085479367, 25.00425949503011225 ) ) ;
#11908=CARTESIAN_POINT ( 'NONE',  ( 5.725930890718300859, 2.506952462184107500, 10.70066851092422411 ) ) ;
#11910=CARTESIAN_POINT ( 'NONE',  ( -2.668367453516648613, -5.373994336898124224, 30.86760611998365178 ) ) ;
#11916=EDGE_CURVE ( 'NONE', #8921, #13014, #12956, .T. ) ;
#11918=CARTESIAN_POINT ( 'NONE',  ( 0.000000000000000000, 6.250000000000000888, 6.000000000000005329 ) ) ;
#11920=EDGE_CURVE ( 'NONE', #7970, #9955, #5760, .T. ) ;
#11921=CARTESIAN_POINT ( 'NONE',  ( 5.782895619916181396, 1.604017620857993709, 17.02591947216898305 ) ) ;
#11923=CARTESIAN_POINT ( 'NONE',  ( 3.421280866381030350, 4.930711975950989867, 19.00004932073311181 ) ) ;
#11925=CARTESIAN_POINT ( 'NONE',  ( -6.176542424588106428, -0.9554180641286325049, 4.867658743658319409 ) ) ;
#11929=CARTESIAN_POINT ( 'NONE',  ( 1.353717517954364224E-13, -6.000000000000000888, 18.99999999999998934 ) ) ;
#11930=ORIENTED_EDGE ( 'NONE', *, *, #10002, .F. ) ;
#11932=ORIENTED_EDGE ( 'NONE', *, *, #8439, .F. ) ;
#11934=ORIENTED_EDGE ( 'NONE', *, *, #7561, .F. ) ;
#11936=CARTESIAN_POINT ( 'NONE',  ( 6.768587589771821120E-14, -6.250000000000000888, 11.49999999999998224 ) ) ;
#11938=EDGE_CURVE ( 'NONE', #7643, #1252, #12202, .T. ) ;
#11940=CARTESIAN_POINT ( 'NONE',  ( 6.176542424588125080, 0.9554180641284967246, 18.13060690723496649 ) ) ;
#11943=VECTOR ( 'NONE', #2191, 1000.000000000000114 ) ;
#11945=DIRECTION ( 'NONE',  ( 0.9510565162951499785, 0.3090169943749582204, 0.000000000000000000 ) ) ;
#11948=CARTESIAN_POINT ( 'NONE',  ( 2.817313151351169331, -5.579000502529441796, 31.00000000000000000 ) ) ;
#11950=CARTESIAN_POINT ( 'NONE',  ( 5.726049995854432417, 2.506679546901958489, 5.799544624688433458 ) ) ;
#11954=ORIENTED_EDGE ( 'NONE', *, *, #2508, .T. ) ;
#11956=CARTESIAN_POINT ( 'NONE',  ( -6.081509788407734263, -1.446521464462734885, 30.12618035954928075 ) ) ;
#11957=CARTESIAN_POINT ( 'NONE',  ( -3.158825713737613228, -5.393784879207096594, 23.70066851092423477 ) ) ;
#11958=CARTESIAN_POINT ( 'NONE',  ( -4.286401442266675410, -4.198423832313046944, 24.49999999999999289 ) ) ;
#11960=EDGE_LOOP ( 'NONE', ( #7711, #5284 ) ) ;
#11961=CARTESIAN_POINT ( 'NONE',  ( -6.081464507797624819, -1.446657058464231538, 31.87380055247395561 ) ) ;
#11962=CARTESIAN_POINT ( 'NONE',  ( 5.747343991580227573, -1.727858744772131194, 17.00007997643736957 ) ) ;
#11963=CARTESIAN_POINT ( 'NONE',  ( -4.322356511625935482, 7.650514973136391284, 24.49999999999999289 ) ) ;
#11964=CARTESIAN_POINT ( 'NONE',  ( -3.459447313391904366, -5.206669755180949544, 18.97400098023329562 ) ) ;
#11965=EDGE_CURVE ( 'NONE', #4625, #10924, #7840, .T. ) ;
#11966=CARTESIAN_POINT ( 'NONE',  ( 5.486982057989157724, 2.429327048029951364, 30.20068193741824913 ) ) ;
#11971=CARTESIAN_POINT ( 'NONE',  ( 2.782468714962362366, 5.316055268221441032, 31.50389795015983552 ) ) ;
#11974=CARTESIAN_POINT ( 'NONE',  ( -4.286401442266593698, 4.198423832313130433, 4.869383044678627925 ) ) ;
#11975=CARTESIAN_POINT ( 'NONE',  ( 2.817313151351108047, 5.579000502529472882, 5.000000000000004441 ) ) ;
#11976=LINE ( 'NONE', #47, #11572 ) ;
#11978=CARTESIAN_POINT ( 'NONE',  ( 2.996920846510581438, -5.485395142346740194, 31.61441947245485196 ) ) ;
#11981=ORIENTED_EDGE ( 'NONE', *, *, #4036, .F. ) ;
#11982=CARTESIAN_POINT ( 'NONE',  ( -4.267838854167198548, 4.217593933790310778, 11.23760108194401042 ) ) ;
#11986=CARTESIAN_POINT ( 'NONE',  ( 2.031800923367348393E-13, -6.250000000000000888, 23.49999999999999289 ) ) ;
#11990=CARTESIAN_POINT ( 'NONE',  ( 6.143143148203048298, 1.154591847827755702, 10.88603820591926841 ) ) ;
#11994=ORIENTED_EDGE ( 'NONE', *, *, #10999, .T. ) ;
#11998=CARTESIAN_POINT ( 'NONE',  ( -3.459447313391845746, -5.206669755180986847, 12.47400098023328674 ) ) ;
#11999=VERTEX_POINT ( 'NONE', #7945 ) ;
#12000=CARTESIAN_POINT ( 'NONE',  ( -2.692215568229910705, -5.362327947133556982, 24.23770962164066844 ) ) ;
#12001=CARTESIAN_POINT ( 'NONE',  ( 0.5043776560899378980, -6.230795654995822552, 25.37337476296011118 ) ) ;
#12003=LINE ( 'NONE', #10972, #6716 ) ;
#12004=FACE_OUTER_BOUND ( 'NONE', #9266, .T. ) ;
#12006=CARTESIAN_POINT ( 'NONE',  ( 2.848235266351056616, -5.281699484015630830, 30.38602261056917442 ) ) ;
#12010=CARTESIAN_POINT ( 'NONE',  ( 0.9740856415301060167, -6.173834621338590622, 30.73852653055532969 ) ) ;
#12011=CARTESIAN_POINT ( 'NONE',  ( -5.770167736194707686, 2.404664418229138345, 10.62632671364005255 ) ) ;
#12013=ADVANCED_FACE ( 'NONE', ( #15033 ), #465, .F. ) ;
#12016=EDGE_CURVE ( 'NONE', #3268, #15268, #8999, .T. ) ;
#12018=B_SPLINE_CURVE_WITH_KNOTS ( 'NONE', 3,
 ( #12603, #13486, #1625, #2750, #6503, #11258, #6577, #2589, #11101, #8890, #123, #14688, #279, #3777, #14769, #2831, #7678, #12527 ),
 .UNSPECIFIED., .F., .F.,
 ( 4, 2, 2, 2, 2, 2, 2, 2, 4 ),
 ( 0.000000000000000000, 0.0003914898357794944594, 0.0007829796715589889189, 0.001174469507338483324, 0.001565959343117977838, 0.001957449178897472351, 0.002348939014676967516, 0.002740428850456463113, 0.003131918686235958278 ),
 .UNSPECIFIED. ) ;
#12019=ORIENTED_EDGE ( 'NONE', *, *, #10132, .T. ) ;
#12020=CARTESIAN_POINT ( 'NONE',  ( -5.317509234263959605, 2.779225709350992002, 31.00000000000000000 ) ) ;
#12023=CARTESIAN_POINT ( 'NONE',  ( -5.859221468178942516, -2.178708437343244597, 12.47408542334169113 ) ) ;
#12028=DIRECTION ( 'NONE',  ( -0.9510565162951544194, 0.3090169943749447312, 0.000000000000000000 ) ) ;
#12029=EDGE_CURVE ( 'NONE', #5008, #15704, #10683, .T. ) ;
#12035=VERTEX_POINT ( 'NONE', #12478 ) ;
#12036=EDGE_CURVE ( 'NONE', #9644, #3914, #543, .T. ) ;
#12038=ORIENTED_EDGE ( 'NONE', *, *, #3989, .F. ) ;
#12040=ORIENTED_EDGE ( 'NONE', *, *, #7132, .T. ) ;
#12041=CARTESIAN_POINT ( 'NONE',  ( 0.5042675786779335922, 6.230788509548837339, 31.87331068310448501 ) ) ;
#12042=CARTESIAN_POINT ( 'NONE',  ( -4.435347140101157493, -4.403429997944390273, 24.36936067245787285 ) ) ;
#12043=CARTESIAN_POINT ( 'NONE',  ( -2.692693252389695147, -5.362085866495053921, 24.76382603205594535 ) ) ;
#12044=CARTESIAN_POINT ( 'NONE',  ( -5.903843691985217745, -2.055287728870688113, 32.00004906876532118 ) ) ;
#12045=CARTESIAN_POINT ( 'NONE',  ( 4.005998022989810892, 4.467726698309398614, 25.29931806258175087 ) ) ;
#12048=CARTESIAN_POINT ( 'NONE',  ( 5.746619684944259454, 1.730157667110885367, 29.99995067926688108 ) ) ;
#12049=CARTESIAN_POINT ( 'NONE',  ( 2.031800923283433283E-13, -6.000000000000000888, 23.49999999999999289 ) ) ;
#12054=EDGE_CURVE ( 'NONE', #14650, #28, #9742, .T. ) ;
#12055=CARTESIAN_POINT ( 'NONE',  ( 5.621197618055683520, 2.101623592078498692, 31.97398020122239259 ) ) ;
#12056=EDGE_LOOP ( 'NONE', ( #5287, #13913 ) ) ;
#12058=CARTESIAN_POINT ( 'NONE',  ( 0.6152055445546975587, -5.969096820685146909, 12.29904968670265930 ) ) ;
#12060=EDGE_LOOP ( 'NONE', ( #2472, #14504, #7468, #2230 ) ) ;
#12063=CARTESIAN_POINT ( 'NONE',  ( -4.196288036172476588, 4.288789315524806689, 10.99687951097621230 ) ) ;
#12064=VECTOR ( 'NONE', #9094, 1000.000000000000114 ) ;
#12074=CARTESIAN_POINT ( 'NONE',  ( 0.8730424326981129912, 5.936362132114460621, 30.49500690218564358 ) ) ;
#12075=ORIENTED_EDGE ( 'NONE', *, *, #14649, .F. ) ;
#12078=CARTESIAN_POINT ( 'NONE',  ( -3.255013540813633366, -5.336859797930840976, 12.37381964045070859 ) ) ;
#12083=CARTESIAN_POINT ( 'NONE',  ( -7.490007020835684592, -2.433650805992431110, 11.49999999999998224 ) ) ;
#12085=CARTESIAN_POINT ( 'NONE',  ( 2.692143549875279707, 5.362363179736537866, 18.26194324003145653 ) ) ;
#12089=CARTESIAN_POINT ( 'NONE',  ( -5.375763363753442547, 2.665284979407548160, 10.99610204984015560 ) ) ;
#12090=CARTESIAN_POINT ( 'NONE',  ( -5.570722351696268504, 2.834100162821960645, 11.23809786915986741 ) ) ;
#12091=CARTESIAN_POINT ( 'NONE',  ( -5.903119516422487223, 1.077859910107424879, 30.38480617551147844 ) ) ;
#12094=EDGE_LOOP ( 'NONE', ( #14768, #12413 ) ) ;
#12095=ORIENTED_EDGE ( 'NONE', *, *, #6399, .F. ) ;
#12099=CARTESIAN_POINT ( 'NONE',  ( 0.1306171417088619613, 6.000000000000000000, 4.000000000000004441 ) ) ;
#12100=FACE_OUTER_BOUND ( 'NONE', #12, .T. ) ;
#12103=CARTESIAN_POINT ( 'NONE',  ( 5.558508435838229289, -2.857531096718853192, 5.000000000000004441 ) ) ;
#12106=CARTESIAN_POINT ( 'NONE',  ( -5.131373506000769247, 7.062729720843990755, 11.49999999999998224 ) ) ;
#12108=AXIS2_PLACEMENT_3D ( 'NONE', #11501, #5551, #12618 ) ;
#12109=CARTESIAN_POINT ( 'NONE',  ( 6.176542424588105540, 0.9554180641286316167, 5.000000000000004441 ) ) ;
#12113=ORIENTED_EDGE ( 'NONE', *, *, #1472, .T. ) ;
#12114=ORIENTED_EDGE ( 'NONE', *, *, #677, .T. ) ;
#12115=CARTESIAN_POINT ( 'NONE',  ( -6.155854678529453672, 1.081900940642229081, 25.00425949503011225 ) ) ;
#12116=EDGE_CURVE ( 'NONE', #10806, #10812, #1940, .T. ) ;
#12117=CARTESIAN_POINT ( 'NONE',  ( -4.152999119458068655, -4.671604476854271049, 23.69973484982322276 ) ) ;
#12118=CARTESIAN_POINT ( 'NONE',  ( 6.176542424588138402, 0.9554180641284283348, 24.36936067245787996 ) ) ;
#12120=CARTESIAN_POINT ( 'NONE',  ( -6.176542424588101987, -0.9554180641286524889, 31.00000000000000000 ) ) ;
#12121=VECTOR ( 'NONE', #9534, 1000.000000000000000 ) ;
#12122=DIRECTION ( 'NONE',  ( -0.5877852522924685852, -0.8090169943749507819, 0.000000000000000000 ) ) ;
#12124=CARTESIAN_POINT ( 'NONE',  ( -2.817313151351249711, 5.579000502529400940, 11.49999999999998224 ) ) ;
#12125=CARTESIAN_POINT ( 'NONE',  ( 0.8737888311111418060, -5.936248257219488345, 18.50344185141215192 ) ) ;
#12127=ADVANCED_FACE ( 'NONE', ( #857, #13103, #10566, #8265, #4685, #1016, #5724, #4522, #9377, #11681, #11825, #932, #1967, #6844, #5798, #15347, #780, #10493, #10644, #1095, #12947, #15506, #2203, #9298, #4604, #5879 ), #3242, .F. ) ;
#12130=B_SPLINE_CURVE_WITH_KNOTS ( 'NONE', 3,
 ( #11350, #5320, #13575, #10165, #15020, #9932, #10012, #13812, #14783, #2684, #12619, #7536, #6360, #11197, #1716, #11427, #296, #3308 ),
 .UNSPECIFIED., .F., .F.,
 ( 4, 2, 2, 2, 2, 2, 2, 2, 4 ),
 ( 0.000000000000000000, 0.0003914357524127504129, 0.0007828715048255008259, 0.001174307257238251185, 0.001565743009651001652, 0.001957178762063751902, 0.002348614514476502369, 0.002740050266889252836, 0.003131486019302003303 ),
 .UNSPECIFIED. ) ;
#12133=CARTESIAN_POINT ( 'NONE',  ( -6.176542424588084224, -0.9554180641287668418, 18.13237410716305220 ) ) ;
#12136=CARTESIAN_POINT ( 'NONE',  ( -5.317509234263939177, 2.779225709351033302, 11.49999999999998224 ) ) ;
#12137=DIRECTION ( 'NONE',  ( 0.9510565162951500895, 0.3090169943749582204, 0.000000000000000000 ) ) ;
#12138=CARTESIAN_POINT ( 'NONE',  ( 5.487097279078493983, 2.429065649168680618, 25.29952054102716019 ) ) ;
#12139=VERTEX_POINT ( 'NONE', #8348 ) ;
#12141=DIRECTION ( 'NONE',  ( -0.3090169943749446202, -0.9510565162951544194, 0.000000000000000000 ) ) ;
#12143=CARTESIAN_POINT ( 'NONE',  ( -4.142620314836410245, 4.341347824677476375, 10.88557478428060499 ) ) ;
#12146=CARTESIAN_POINT ( 'NONE',  ( -4.290821322214536160, 4.545321419741401137, 23.88558052754514804 ) ) ;
#12153=ORIENTED_EDGE ( 'NONE', *, *, #10697, .F. ) ;
#12155=AXIS2_PLACEMENT_3D ( 'NONE', #10554, #2267, #9768 ) ;
#12158=EDGE_LOOP ( 'NONE', ( #8864, #10556 ) ) ;
#12160=CARTESIAN_POINT ( 'NONE',  ( -5.317509234263835260, -2.779225709351231366, 24.49999999999999289 ) ) ;
#12161=EDGE_CURVE ( 'NONE', #7643, #14650, #13187, .T. ) ;
#12162=CARTESIAN_POINT ( 'NONE',  ( 1.354942164753511828E-13, -6.250000000000000888, 16.99999999999998579 ) ) ;
#12166=CARTESIAN_POINT ( 'NONE',  ( 4.267558728637157905, -4.217879122113839863, 18.26382603205596311 ) ) ;
#12171=CARTESIAN_POINT ( 'NONE',  ( -0.6144300524832365662, -6.220417338033064070, 17.20033372175933195 ) ) ;
#12175=EDGE_LOOP ( 'NONE', ( #3117, #746 ) ) ;
#12177=ORIENTED_EDGE ( 'NONE', *, *, #2206, .T. ) ;
#12178=CARTESIAN_POINT ( 'NONE',  ( -4.005361199355159663, 4.468319061418626781, 25.30022217383879024 ) ) ;
#12179=ORIENTED_EDGE ( 'NONE', *, *, #4196, .T. ) ;
#12182=DIRECTION ( 'NONE',  ( -0.3090169943749584980, 0.9510565162951498674, 0.000000000000000000 ) ) ;
#12185=CARTESIAN_POINT ( 'NONE',  ( -5.931734679891455642, 0.9039278060243561841, 31.26382603205594179 ) ) ;
#12186=CARTESIAN_POINT ( 'NONE',  ( -5.770167736194620645, -2.404664418229350620, 25.37367328635991726 ) ) ;
#12190=CARTESIAN_POINT ( 'NONE',  ( 5.859155363331360888, 2.178872204145034797, 5.974000980233302727 ) ) ;
#12191=VERTEX_POINT ( 'NONE', #13573 ) ;
#12192=VERTEX_POINT ( 'NONE', #12302 ) ;
#12197=CARTESIAN_POINT ( 'NONE',  ( 6.123233995736766282E-16, -6.250000000000000888, 6.000000000000005329 ) ) ;
#12198=CARTESIAN_POINT ( 'NONE',  ( -6.176542424588100211, -0.9554180641286524889, 31.13237410716304510 ) ) ;
#12202=B_SPLINE_CURVE_WITH_KNOTS ( 'NONE', 3,
 ( #155, #3964, #1188, #2703, #6061, #7553, #1267, #2466, #3655, #5019, #12401, #9874, #8532, #13361, #9796, #1501, #14727, #11211 ),
 .UNSPECIFIED., .F., .F.,
 ( 4, 2, 2, 2, 2, 2, 2, 2, 4 ),
 ( 0.003131486019301978150, 0.003522824630466687024, 0.003914163241631395465, 0.004305501852796104340, 0.004696840463960812347, 0.005088179075125520354, 0.005479517686290228361, 0.005870856297454936368, 0.006262194908619644375 ),
 .UNSPECIFIED. ) ;
#12209=CARTESIAN_POINT ( 'NONE',  ( 5.915699123067165388, 1.003533581835513999, 10.99610204984015915 ) ) ;
#12212=EDGE_LOOP ( 'NONE', ( #5829, #1602, #259, #9399 ) ) ;
#12215=CARTESIAN_POINT ( 'NONE',  ( 5.665707375537499146, 1.979196487016603667, 25.50007961174476279 ) ) ;
#12216=CARTESIAN_POINT ( 'NONE',  ( -4.435347140101057128, -4.403429997944487084, 11.49999999999998224 ) ) ;
#12218=CARTESIAN_POINT ( 'NONE',  ( -3.634089073485479382, 4.776071126502653641, 10.50007997643736601 ) ) ;
#12219=EDGE_CURVE ( 'NONE', #7578, #5982, #12749, .T. ) ;
#12221=CARTESIAN_POINT ( 'NONE',  ( 0.000000000000000000, 6.250000000000000888, 18.99999999999998934 ) ) ;
#12224=CYLINDRICAL_SURFACE ( 'NONE', #12620, 6.250000000000000888 ) ;
#12225=ADVANCED_FACE ( 'NONE', ( #11717 ), #11560, .F. ) ;
#12228=CARTESIAN_POINT ( 'NONE',  ( 5.903596343266304558, 2.055998103990562154, 17.00004921015705861 ) ) ;
#12229=EDGE_LOOP ( 'NONE', ( #5668, #2650, #863, #7542 ) ) ;
#12232=CARTESIAN_POINT ( 'NONE',  ( 5.409274167810704803, 2.597759609440538853, 23.88480617551148555 ) ) ;
#12234=EDGE_LOOP ( 'NONE', ( #7877, #4290, #14487, #10573 ) ) ;
#12235=CARTESIAN_POINT ( 'NONE',  ( -3.922672396097165670, -4.541739265057607611, 23.62635295315577011 ) ) ;
#12236=CARTESIAN_POINT ( 'NONE',  ( 5.903347812666353001, -1.076697810262575272, 5.613977389430843346 ) ) ;
#12237=EDGE_CURVE ( 'NONE', #13722, #10051, #10294, .T. ) ;
#12238=CARTESIAN_POINT ( 'NONE',  ( 6.020822430078805354, -1.681351817312369823, 31.97408542334170889 ) ) ;
#12239=CARTESIAN_POINT ( 'NONE',  ( -4.322356511625826236, 7.650514973136471220, 11.49999999999998224 ) ) ;
#12244=CARTESIAN_POINT ( 'NONE',  ( -0.5031281619707573816, -5.980084330432670292, 30.12602272744525678 ) ) ;
#12245=CARTESIAN_POINT ( 'NONE',  ( 5.747343991580209810, -1.727858744772199584, 10.50007997643736424 ) ) ;
#12246=CARTESIAN_POINT ( 'NONE',  ( -5.329907877631365309, 2.755840666746240508, 11.23805675996853104 ) ) ;
#12253=ORIENTED_EDGE ( 'NONE', *, *, #15184, .F. ) ;
#12254=AXIS2_PLACEMENT_3D ( 'NONE', #7058, #7221, #3547 ) ;
#12264=CARTESIAN_POINT ( 'NONE',  ( 3.312524433819824754, 5.004191858253972391, 5.974080527831012510 ) ) ;
#12267=CYLINDRICAL_SURFACE ( 'NONE', #9884, 0.9999999999999998890 ) ;
#12273=CARTESIAN_POINT ( 'NONE',  ( 5.935543223013862502, -0.8771126767606430841, 31.00000000000000000 ) ) ;
#12274=CARTESIAN_POINT ( 'NONE',  ( 4.435347140101058905, -4.403429997944484420, 31.00000000000000000 ) ) ;
#12275=CARTESIAN_POINT ( 'NONE',  ( -0.9739805876847985600, -5.920636045238166112, 5.261713868144209272 ) ) ;
#12277=CARTESIAN_POINT ( 'NONE',  ( 1.000049271338626644, -6.169473353325530596, 17.86969612704554322 ) ) ;
#12278=CARTESIAN_POINT ( 'NONE',  ( 0.9737778612006245949, 5.920671847850506708, 11.23736375884651828 ) ) ;
#12280=CARTESIAN_POINT ( 'NONE',  ( -6.176542424588120639, 0.9554180641285460185, 5.000000000000004441 ) ) ;
#12290=CARTESIAN_POINT ( 'NONE',  ( 4.153663429050794775, -4.670992970568362601, 10.70066851092421878 ) ) ;
#12291=CARTESIAN_POINT ( 'NONE',  ( 5.915755444410821795, 1.003187219519724893, 25.00312048902375395 ) ) ;
#12292=CARTESIAN_POINT ( 'NONE',  ( 0.2638277032950948620, 5.995407492418031836, 25.47332055281517782 ) ) ;
#12302=CARTESIAN_POINT ( 'NONE',  ( 5.317509234263970264, -2.779225709350972906, 5.000000000000004441 ) ) ;
#12303=FACE_OUTER_BOUND ( 'NONE', #11142, .T. ) ;
#12304=CARTESIAN_POINT ( 'NONE',  ( 0.9999196734182850266, 5.916093360767511022, 30.86725955955067136 ) ) ;
#12305=ORIENTED_EDGE ( 'NONE', *, *, #2535, .T. ) ;
#12308=B_SPLINE_CURVE_WITH_KNOTS ( 'NONE', 3,
 ( #15385, #4481, #3284, #6957, #11001, #14665, #5995, #2403, #3519, #13140, #8302, #15544, #9572, #13061, #9817, #2159, #14500, #8390 ),
 .UNSPECIFIED., .F., .F.,
 ( 4, 2, 2, 2, 2, 2, 2, 2, 4 ),
 ( 0.000000000000000000, 0.0003914357524127473230, 0.0007828715048254946459, 0.001174307257238241860, 0.001565743009650990376, 0.001957178762063739759, 0.002348614514476488925, 0.002740050266889238525, 0.003131486019301987691 ),
 .UNSPECIFIED. ) ;
#12311=EDGE_LOOP ( 'NONE', ( #15569, #11367, #1913, #6147 ) ) ;
#12312=FACE_OUTER_BOUND ( 'NONE', #12774, .T. ) ;
#12315=CYLINDRICAL_SURFACE ( 'NONE', #15448, 1.000000000000000666 ) ;
#12320=CARTESIAN_POINT ( 'NONE',  ( 5.329945432499706648, -2.755769831644989232, 24.76229037835931734 ) ) ;
#12324=CARTESIAN_POINT ( 'NONE',  ( -0.7995524673974289120, -6.199337389817286770, 18.61453679452458232 ) ) ;
#12325=CARTESIAN_POINT ( 'NONE',  ( 7.490007020835686369, -2.433650805992243260, 5.000000000000004441 ) ) ;
#12326=CARTESIAN_POINT ( 'NONE',  ( 4.141923667210504867, 4.342011609040599573, 23.88438267301394191 ) ) ;
#12327=B_SPLINE_CURVE_WITH_KNOTS ( 'NONE', 3,
 ( #9558, #2141, #10745, #8287, #6863, #12884, #4390, #14158, #1911, #14396, #6784, #3340, #10513, #2223, #3261, #5898, #1034, #11929 ),
 .UNSPECIFIED., .F., .F.,
 ( 4, 2, 2, 2, 2, 2, 2, 2, 4 ),
 ( 0.003131923598877003109, 0.003523316383094320450, 0.003914709167311637358, 0.004306101951528954266, 0.004697494735746271174, 0.005088887519963588082, 0.005480280304180905858, 0.005871673088398223633, 0.006263065872615540541 ),
 .UNSPECIFIED. ) ;
#12328=ORIENTED_EDGE ( 'NONE', *, *, #7354, .F. ) ;
#12330=ORIENTED_EDGE ( 'NONE', *, *, #10606, .F. ) ;
#12332=CARTESIAN_POINT ( 'NONE',  ( -5.375763363753348401, -2.665284979407742671, 25.00389795015983552 ) ) ;
#12339=B_SPLINE_CURVE_WITH_KNOTS ( 'NONE', 3,
 ( #12772, #10480, #1798, #6984, #15253, #11813, #4354, #1955, #9363, #14124, #9213, #14204, #917, #4431, #8012, #15410, #11506, #3157 ),
 .UNSPECIFIED., .F., .F.,
 ( 4, 2, 2, 2, 2, 2, 2, 2, 4 ),
 ( 0.003131486019301973813, 0.003522824630466682688, 0.003914163241631391128, 0.004305501852796100003, 0.004696840463960808877, 0.005088179075125516884, 0.005479517686290227493, 0.005870856297454936368, 0.006262194908619646110 ),
 .UNSPECIFIED. ) ;
#12341=CARTESIAN_POINT ( 'NONE',  ( 5.616116467183635663, -2.743044348085595718, 4.495740504969914397 ) ) ;
#12343=CARTESIAN_POINT ( 'NONE',  ( 3.419318284370281180, -4.932111238568118949, 31.99992002356261267 ) ) ;
#12345=DIRECTION ( 'NONE',  ( 0.000000000000000000, 1.000000000000000000, 0.000000000000000000 ) ) ;
#12348=ORIENTED_EDGE ( 'NONE', *, *, #15326, .T. ) ;
#12349=EDGE_LOOP ( 'NONE', ( #4854, #8116, #10790, #13194 ) ) ;
#12351=CARTESIAN_POINT ( 'NONE',  ( 5.915755444410805808, -1.003187219519832585, 30.49687951097622118 ) ) ;
#12353=CARTESIAN_POINT ( 'NONE',  ( 0.1306070469493385289, 6.250000000000000000, 4.000000000000004441 ) ) ;
#12355=CARTESIAN_POINT ( 'NONE',  ( 0.2638277032949492007, 5.995407492418038053, 12.47332055281516716 ) ) ;
#12359=CARTESIAN_POINT ( 'NONE',  ( -5.558508435838226625, 2.857531096718854968, 5.130606907234993130 ) ) ;
#12360=CARTESIAN_POINT ( 'NONE',  ( 0.9740807849838198917, -5.920620690450655310, 24.23850119700669126 ) ) ;
#12366=ORIENTED_EDGE ( 'NONE', *, *, #358, .T. ) ;
#12367=CARTESIAN_POINT ( 'NONE',  ( -5.726307184802613470, 2.506131700382554950, 17.19973484982324408 ) ) ;
#12368=APPLICATION_CONTEXT ( 'automotive_design' ) ;
#12369=CARTESIAN_POINT ( 'NONE',  ( -5.570722351696208108, 2.834100162822084101, 24.23809786915987985 ) ) ;
#12370=CARTESIAN_POINT ( 'NONE',  ( -0.1323736289504354180, 6.250000000000000888, 6.000000000000004441 ) ) ;
#12371=CARTESIAN_POINT ( 'NONE',  ( 6.020822430078779597, 1.681351817312460861, 30.02591457665829111 ) ) ;
#12373=CARTESIAN_POINT ( 'NONE',  ( -3.883588957979168477, -4.898466244119000557, 31.97377282875268989 ) ) ;
#12375=CARTESIAN_POINT ( 'NONE',  ( -4.070863287254287144, 4.743975846881624214, 23.62694108445698760 ) ) ;
#12376=ORIENTED_EDGE ( 'NONE', *, *, #13518, .F. ) ;
#12377=CARTESIAN_POINT ( 'NONE',  ( -3.882673863916222601, -4.899192824800991275, 30.02591457665829466 ) ) ;
#12383=CARTESIAN_POINT ( 'NONE',  ( 6.081590040723123813, -1.446205118472801754, 25.37367328635992081 ) ) ;
#12390=CARTESIAN_POINT ( 'NONE',  ( -4.152999119458038457, -4.671604476854300358, 17.19973484982324408 ) ) ;
#12392=DIRECTION ( 'NONE',  ( -0.5877852522924685852, -0.8090169943749508930, 0.000000000000000000 ) ) ;
#12393=CARTESIAN_POINT ( 'NONE',  ( 4.344313232727081697, -4.493553492990136178, 17.49563030319847101 ) ) ;
#12394=CARTESIAN_POINT ( 'NONE',  ( -5.375763363753478075, 2.665284979407481547, 4.496102049840166259 ) ) ;
#12395=CARTESIAN_POINT ( 'NONE',  ( -0.6156133477426046774, -6.220296490279947577, 12.29872387345510454 ) ) ;
#12396=CARTESIAN_POINT ( 'NONE',  ( 2.668367453516506504, 5.373994336898192614, 17.99999999999998934 ) ) ;
#12398=FACE_OUTER_BOUND ( 'NONE', #3245, .T. ) ;
#12399=CARTESIAN_POINT ( 'NONE',  ( 5.375913338529123564, -2.664979843780373336, 10.99571079637980553 ) ) ;
#12400=AXIS2_PLACEMENT_3D ( 'NONE', #10441, #1763, #15294 ) ;
#12401=CARTESIAN_POINT ( 'NONE',  ( -3.459447313391871059, 5.206669755180970860, 30.02599901976670438 ) ) ;
#12403=CARTESIAN_POINT ( 'NONE',  ( -5.665308849928797130, -1.980336949702578009, 10.50007997643736424 ) ) ;
#12407=EDGE_CURVE ( 'NONE', #5925, #2012, #4202, .T. ) ;
#12409=CARTESIAN_POINT ( 'NONE',  ( -5.935543223013816316, -0.8771126767609508379, 24.49999999999999289 ) ) ;
#12412=CARTESIAN_POINT ( 'NONE',  ( 4.435347140100866170, 4.403429997944679819, 24.49999999999999289 ) ) ;
#12413=ORIENTED_EDGE ( 'NONE', *, *, #7306, .F. ) ;
#12416=CARTESIAN_POINT ( 'NONE',  ( -3.781065399485988188, 4.978303713186458701, 4.000082581897114409 ) ) ;
#12418=DIRECTION ( 'NONE',  ( 0.5877852522924802425, -0.8090169943749422332, 0.000000000000000000 ) ) ;
#12420=CARTESIAN_POINT ( 'NONE',  ( -4.286401442266690509, 4.198423832313033621, 17.86938304467860306 ) ) ;
#12421=CARTESIAN_POINT ( 'NONE',  ( 3.922288969639793343, 4.542045818322514528, 5.873784308702619583 ) ) ;
#12423=CARTESIAN_POINT ( 'NONE',  ( 5.571002711501443549, -2.833546409886217976, 11.23620383159194525 ) ) ;
#12425=EDGE_CURVE ( 'NONE', #8130, #159, #2243, .T. ) ;
#12426=VERTEX_POINT ( 'NONE', #13142 ) ;
#12430=CARTESIAN_POINT ( 'NONE',  ( 0.9739805876849262356, 5.920636045238144796, 18.26171386814421638 ) ) ;
#12434=CARTESIAN_POINT ( 'NONE',  ( 0.9740807849836315979, -5.920620690450686396, 30.73850119700668415 ) ) ;
#12436=AXIS2_PLACEMENT_3D ( 'NONE', #348, #189, #3844 ) ;
#12440=B_SPLINE_CURVE_WITH_KNOTS ( 'NONE', 3,
 ( #9652, #2314, #13298, #2560, #10832, #90, #15694, #14493, #10917, #6073, #8698, #3590, #14408, #3513, #9734, #15614, #3746, #4716 ),
 .UNSPECIFIED., .F., .F.,
 ( 4, 2, 2, 2, 2, 2, 2, 2, 4 ),
 ( 0.003131486019301973379, 0.003522824630466680519, 0.003914163241631388526, 0.004305501852796095666, 0.004696840463960802806, 0.005088179075125510813, 0.005479517686290218820, 0.005870856297454926827, 0.006262194908619634834 ),
 .UNSPECIFIED. ) ;
#12447=EDGE_CURVE ( 'NONE', #10051, #8233, #15621, .T. ) ;
#12448=ORIENTED_EDGE ( 'NONE', *, *, #8473, .T. ) ;
#12449=CARTESIAN_POINT ( 'NONE',  ( -5.915641100987826029, 1.003868594704782069, 12.00428920362018914 ) ) ;
#12450=FACE_OUTER_BOUND ( 'NONE', #11774, .T. ) ;
#12452=CARTESIAN_POINT ( 'NONE',  ( 6.143143148203041193, 1.154591847827807882, 30.38603820591927374 ) ) ;
#12455=CARTESIAN_POINT ( 'NONE',  ( -2.817313151351126255, -5.579000502529464001, 31.00000000000000000 ) ) ;
#12457=CARTESIAN_POINT ( 'NONE',  ( 5.867109477881239599, -1.259218163100936927, 4.201117577520603774 ) ) ;
#12458=CARTESIAN_POINT ( 'NONE',  ( -4.291255145204003973, -4.544933371694741098, 30.38603820591928439 ) ) ;
#12460=FACE_BOUND ( 'NONE', #8175, .T. ) ;
#12466=CARTESIAN_POINT ( 'NONE',  ( -5.375763363753377710, -2.665284979407680943, 18.50389795015982841 ) ) ;
#12470=CARTESIAN_POINT ( 'NONE',  ( 5.558508435838283468, 2.857531096718750607, 24.49999999999999289 ) ) ;
#12474=CARTESIAN_POINT ( 'NONE',  ( 5.866817325727553545, -1.260653813891763120, 25.30022217383879024 ) ) ;
#12477=CARTESIAN_POINT ( 'NONE',  ( 5.409423237179043831, -2.597448116730963985, 10.88438267301394191 ) ) ;
#12478=CARTESIAN_POINT ( 'NONE',  ( 2.668367453516690357, -5.373994336898101132, 31.00000000000000000 ) ) ;
#12480=AXIS2_PLACEMENT_3D ( 'NONE', #7301, #9526, #9772 ) ;
#12482=VERTEX_POINT ( 'NONE', #3598 ) ;
#12485=CARTESIAN_POINT ( 'NONE',  ( -5.866923913994597228, -1.260079467906751516, 23.70047945897283270 ) ) ;
#12486=ORIENTED_EDGE ( 'NONE', *, *, #2586, .F. ) ;
#12489=ORIENTED_EDGE ( 'NONE', *, *, #14068, .T. ) ;
#12492=B_SPLINE_CURVE_WITH_KNOTS ( 'NONE', 3,
 ( #12514, #2971, #421, #346, #9983, #11400, #7822, #5210, #1537, #12590, #1688, #15067, #6565, #11325, #1769, #11244, #4000, #9033 ),
 .UNSPECIFIED., .F., .F.,
 ( 4, 2, 2, 2, 2, 2, 2, 2, 4 ),
 ( 0.003131490185285952174, 0.003522829482338570451, 0.003914168779391188728, 0.004305508076443806571, 0.004696847373496425282, 0.005088186670549043125, 0.005479525967601660968, 0.005870865264654279679, 0.006262204561706897522 ),
 .UNSPECIFIED. ) ;
#12493=CARTESIAN_POINT ( 'NONE',  ( 1.353717517954364224E-13, 6.000000000000000888, 18.99999999999998934 ) ) ;
#12497=EDGE_CURVE ( 'NONE', #1820, #15059, #2405, .T. ) ;
#12498=CARTESIAN_POINT ( 'NONE',  ( -3.922672396097048875, -4.541739265057705310, 10.62635295315574702 ) ) ;
#12499=CARTESIAN_POINT ( 'NONE',  ( -6.081464507797580410, -1.446657058464413170, 25.37380055247394495 ) ) ;
#12501=CARTESIAN_POINT ( 'NONE',  ( -5.984595133899190955, 1.806709459528622386, 30.00004921015706572 ) ) ;
#12502=CARTESIAN_POINT ( 'NONE',  ( -0.8002720181890644602, 6.199262377003409874, 30.38606262465555474 ) ) ;
#12503=ORIENTED_EDGE ( 'NONE', *, *, #4450, .F. ) ;
#12506=EDGE_LOOP ( 'NONE', ( #4356, #13385 ) ) ;
#12507=CARTESIAN_POINT ( 'NONE',  ( 5.783198643800777639, -1.602922020054677432, 30.02622176056706493 ) ) ;
#12509=ORIENTED_EDGE ( 'NONE', *, *, #11938, .T. ) ;
#12510=CARTESIAN_POINT ( 'NONE',  ( -5.903061651806559063, -2.057626436184912144, 17.00008258189709309 ) ) ;
#12511=CARTESIAN_POINT ( 'NONE',  ( -3.634089073485469168, -4.776071126502662523, 18.99992002356260912 ) ) ;
#12513=CARTESIAN_POINT ( 'NONE',  ( -0.6139731865238436948, 6.220476368274066914, 17.19975545601930733 ) ) ;
#12514=CARTESIAN_POINT ( 'NONE',  ( 1.354942165116848791E-13, 6.250000000000000888, 16.99999999999998579 ) ) ;
#12517=CARTESIAN_POINT ( 'NONE',  ( -3.567258970016013553, 5.133675764669650476, 10.49991780678442232 ) ) ;
#12518=CARTESIAN_POINT ( 'NONE',  ( 4.286401442266483564, 4.198423832313243231, 11.49999999999998224 ) ) ;
#12522=EDGE_CURVE ( 'NONE', #28, #14650, #11216, .T. ) ;
#12526=ORIENTED_EDGE ( 'NONE', *, *, #15436, .F. ) ;
#12527=CARTESIAN_POINT ( 'NONE',  ( -4.286401442266592809, 4.198423832313131321, 5.000000000000004441 ) ) ;
#12528=CARTESIAN_POINT ( 'NONE',  ( -5.648559266344472363, 2.676764518776052704, 23.88603820591928084 ) ) ;
#12529=CARTESIAN_POINT ( 'NONE',  ( -4.267838854167295359, 4.217593933790213079, 24.23760108194401397 ) ) ;
#12530=CARTESIAN_POINT ( 'NONE',  ( 5.859155363331391086, 2.178872204144949531, 12.47400098023328852 ) ) ;
#12532=CARTESIAN_POINT ( 'NONE',  ( 3.312524433819711511, -5.004191858254047887, 23.52591947216898660 ) ) ;
#12536=ADVANCED_FACE ( 'NONE', ( #5580 ), #9467, .F. ) ;
#12538=DIRECTION ( 'NONE',  ( 0.5877852522924802425, -0.8090169943749422332, 0.000000000000000000 ) ) ;
#12543=CARTESIAN_POINT ( 'NONE',  ( 6.176542424588150837, -0.9554180641283406272, 24.63063932754212004 ) ) ;
#12544=CARTESIAN_POINT ( 'NONE',  ( -6.000000000000000888, 0.000000000000000000, 36.00000000000000711 ) ) ;
#12547=DIRECTION ( 'NONE',  ( -0.5877852522924685852, -0.8090169943749507819, 0.000000000000000000 ) ) ;
#12549=ORIENTED_EDGE ( 'NONE', *, *, #5329, .T. ) ;
#12551=CARTESIAN_POINT ( 'NONE',  ( 5.858736126997183824, -2.179962889276933602, 12.47359571723299965 ) ) ;
#12556=CARTESIAN_POINT ( 'NONE',  ( 4.286401442266591033, -4.198423832313133097, 5.132360785839115813 ) ) ;
#12557=CARTESIAN_POINT ( 'NONE',  ( 6.021135683317753617, -1.680226122398018163, 23.52622717124730656 ) ) ;
#12558=EDGE_CURVE ( 'NONE', #4806, #10183, #14294, .T. ) ;
#12561=EDGE_LOOP ( 'NONE', ( #12549, #1815, #7798, #4216 ) ) ;
#12564=CARTESIAN_POINT ( 'NONE',  ( -5.782947755040608762, -1.603807858344187487, 23.52601979877760030 ) ) ;
#12566=ORIENTED_EDGE ( 'NONE', *, *, #11920, .F. ) ;
#12568=CARTESIAN_POINT ( 'NONE',  ( -4.322356511625935482, 7.650514973136391284, 24.49999999999999289 ) ) ;
#12569=ORIENTED_EDGE ( 'NONE', *, *, #943, .T. ) ;
#12571=CARTESIAN_POINT ( 'NONE',  ( -3.159082487394791361, 5.393634094348326080, 4.200455375311574535 ) ) ;
#12576=CARTESIAN_POINT ( 'NONE',  ( 6.123233995736766282E-16, -6.250000000000000888, 5.000000000000004441 ) ) ;
#12578=CARTESIAN_POINT ( 'NONE',  ( -5.317509234263873452, 2.779225709351156315, 24.49999999999999289 ) ) ;
#12583=ORIENTED_EDGE ( 'NONE', *, *, #9643, .F. ) ;
#12584=CARTESIAN_POINT ( 'NONE',  ( -5.558508435838158235, -2.857531096718993080, 11.36939309276498911 ) ) ;
#12588=CARTESIAN_POINT ( 'NONE',  ( -2.668367453516752974, -5.373994336898072710, 17.99999999999998934 ) ) ;
#12589=CARTESIAN_POINT ( 'NONE',  ( -0.1323736289504275354, 6.250000000000000000, 18.99999999999997158 ) ) ;
#12590=CARTESIAN_POINT ( 'NONE',  ( 1.000082492230843334, 6.169467968613687070, 18.13152538105398293 ) ) ;
#12593=CARTESIAN_POINT ( 'NONE',  ( 3.735808404764946467, 4.696639218303165997, 10.52601979877758787 ) ) ;
#12601=VERTEX_POINT ( 'NONE', #15510 ) ;
#12603=CARTESIAN_POINT ( 'NONE',  ( -2.668367453516708565, 5.373994336898094026, 5.000000000000004441 ) ) ;
#12604=CARTESIAN_POINT ( 'NONE',  ( -6.176542424588088664, 0.9554180641287480791, 24.49999999999999289 ) ) ;
#12605=CARTESIAN_POINT ( 'NONE',  ( -0.6139731865239884678, 6.220476368274053591, 4.199755456019329536 ) ) ;
#12606=CARTESIAN_POINT ( 'NONE',  ( 5.558508435838199979, 2.857531096718914476, 31.00000000000000000 ) ) ;
#12610=CARTESIAN_POINT ( 'NONE',  ( -3.781065399485938894, -4.978303713186498669, 31.99991741810289625 ) ) ;
#12612=CARTESIAN_POINT ( 'NONE',  ( -4.286401442266546624, -4.198423832313178394, 31.00000000000000000 ) ) ;
#12614=CARTESIAN_POINT ( 'NONE',  ( -3.255128505894239854, -5.336774832660761803, 30.12619944752604084 ) ) ;
#12618=DIRECTION ( 'NONE',  ( -1.000000000000000000, 0.000000000000000000, 0.000000000000000000 ) ) ;
#12619=CARTESIAN_POINT ( 'NONE',  ( 3.459597053047784865, 5.206576120509786243, 12.47408542334169113 ) ) ;
#12620=AXIS2_PLACEMENT_3D ( 'NONE', #6199, #11036, #9789 ) ;
#12623=CARTESIAN_POINT ( 'NONE',  ( -3.922672396097174552, 4.541739265057599617, 18.87364704684421923 ) ) ;
#12625=ORIENTED_EDGE ( 'NONE', *, *, #5440, .F. ) ;
#12626=CARTESIAN_POINT ( 'NONE',  ( -4.005361199355057522, -4.468319061418718263, 17.19977782616121686 ) ) ;
#12632=CARTESIAN_POINT ( 'NONE',  ( -0.9999502950801862911, 5.916088184763887092, 31.13108149190011176 ) ) ;
#12634=DIRECTION ( 'NONE',  ( -0.9510565162951545304, 0.3090169943749447867, 0.000000000000000000 ) ) ;
#12636=EDGE_CURVE ( 'NONE', #6786, #6402, #13740, .T. ) ;
#12637=CARTESIAN_POINT ( 'NONE',  ( -5.375605342016462451, -2.665598297262376182, 10.99687951097621408 ) ) ;
#12638=ORIENTED_EDGE ( 'NONE', *, *, #13872, .T. ) ;
#12642=FACE_OUTER_BOUND ( 'NONE', #2552, .T. ) ;
#12643=EDGE_LOOP ( 'NONE', ( #4309, #13849 ) ) ;
#12647=EDGE_LOOP ( 'NONE', ( #13143, #13310, #3682, #6709 ) ) ;
#12648=CARTESIAN_POINT ( 'NONE',  ( -5.665308849928812229, -1.980336949702540261, 30.00007997643738022 ) ) ;
#12650=CARTESIAN_POINT ( 'NONE',  ( 0.5042987395407738660, 5.979983180450076041, 5.873293041799771963 ) ) ;
#12651=VECTOR ( 'NONE', #1404, 1000.000000000000000 ) ;
#12652=CARTESIAN_POINT ( 'NONE',  ( 5.783198643800823824, -1.602922020054500463, 23.52622176056705783 ) ) ;
#12654=CARTESIAN_POINT ( 'NONE',  ( -5.615973259022306152, -2.743340227996199587, 5.503892131249681796 ) ) ;
#12658=CARTESIAN_POINT ( 'NONE',  ( -7.490007020835705909, -2.433650805992367161, 5.000000000000004441 ) ) ;
#12660=CARTESIAN_POINT ( 'NONE',  ( 2.094888806938587637E-14, 6.250000000000000888, 30.00000000000000000 ) ) ;
#12662=VERTEX_POINT ( 'NONE', #12544 ) ;
#12664=ORIENTED_EDGE ( 'NONE', *, *, #8143, .T. ) ;
#12665=CARTESIAN_POINT ( 'NONE',  ( 3.458623254138732950, -5.207221900902805345, 12.47377282875266324 ) ) ;
#12666=CARTESIAN_POINT ( 'NONE',  ( 5.858736126997123428, 2.179962889277093918, 4.026404282766995912 ) ) ;
#12667=ORIENTED_EDGE ( 'NONE', *, *, #14471, .T. ) ;
#12668=CARTESIAN_POINT ( 'NONE',  ( 5.843075991566613503, -1.368655265450920533, 18.87364704684421923 ) ) ;
#12670=CARTESIAN_POINT ( 'NONE',  ( -3.567624405365311446, 5.133384272590732600, 31.99995078984293428 ) ) ;
#12671=CARTESIAN_POINT ( 'NONE',  ( 5.726049995854478603, -2.506679546901855460, 30.20045537531156654 ) ) ;
#12673=DIRECTION ( 'NONE',  ( 0.5877852522924802425, -0.8090169943749422332, 0.000000000000000000 ) ) ;
#12680=B_SPLINE_CURVE_WITH_KNOTS ( 'NONE', 3,
 ( #15145, #14991, #502, #4082, #7743, #1687, #5369, #15066, #4162, #9032, #5445, #2970, #10291, #4239, #10367, #9108, #7900, #12741 ),
 .UNSPECIFIED., .F., .F.,
 ( 4, 2, 2, 2, 2, 2, 2, 2, 4 ),
 ( 0.003131918686235971288, 0.003523310662250261124, 0.003914702638264550526, 0.004306094614278840361, 0.004697486590293130197, 0.005088878566307420033, 0.005480270542321709869, 0.005871662518335999704, 0.006263054494350289540 ),
 .UNSPECIFIED. ) ;
#12681=EDGE_LOOP ( 'NONE', ( #800, #5841 ) ) ;
#12682=CARTESIAN_POINT ( 'NONE',  ( 3.922288969639853295, -4.542045818322462125, 4.126215691297385746 ) ) ;
#12683=ORIENTED_EDGE ( 'NONE', *, *, #10429, .T. ) ;
#12684=DIRECTION ( 'NONE',  ( 0.5877852522924802425, -0.8090169943749422332, 0.000000000000000000 ) ) ;
#12686=CARTESIAN_POINT ( 'NONE',  ( 0.2619041840695610635, -6.245686665308499919, 10.52605849433793495 ) ) ;
#12687=CARTESIAN_POINT ( 'NONE',  ( -0.9735856429312839122, 5.920699391845025694, 5.262852839067274857 ) ) ;
#12689=CARTESIAN_POINT ( 'NONE',  ( 4.416779112813651764, 4.422345839825798208, 5.262252817217140333 ) ) ;
#12690=CARTESIAN_POINT ( 'NONE',  ( 2.817313151351064970, -5.579000502529494199, 17.86936067245787285 ) ) ;
#12692=CARTESIAN_POINT ( 'NONE',  ( 3.311576095066571579, 5.004818610361311926, 4.026221760567070262 ) ) ;
#12693=CARTESIAN_POINT ( 'NONE',  ( -4.070051655338055241, -4.744673454622520659, 30.12632671364007564 ) ) ;
#12698=CARTESIAN_POINT ( 'NONE',  ( 6.143143148203090043, -1.154591847827534101, 25.11396179408070850 ) ) ;
#12702=DIRECTION ( 'NONE',  ( 0.000000000000000000, 0.000000000000000000, 1.000000000000000000 ) ) ;
#12706=CARTESIAN_POINT ( 'NONE',  ( -4.286401442266688733, 4.198423832313033621, 17.99999999999998934 ) ) ;
#12711=CARTESIAN_POINT ( 'NONE',  ( -0.9740807849835945165, 5.920620690450692614, 30.73850119700669126 ) ) ;
#12713=CARTESIAN_POINT ( 'NONE',  ( -4.286401442266607908, 4.198423832313116222, 30.86938304467861016 ) ) ;
#12715=FACE_OUTER_BOUND ( 'NONE', #14446, .T. ) ;
#12718=ORIENTED_EDGE ( 'NONE', *, *, #11282, .T. ) ;
#12721=CARTESIAN_POINT ( 'NONE',  ( 2.094888799673178700E-14, -6.250000000000000888, 30.00000000000000000 ) ) ;
#12722=CARTESIAN_POINT ( 'NONE',  ( -2.668367453516630849, -5.373994336898132218, 5.000000000000004441 ) ) ;
#12723=CARTESIAN_POINT ( 'NONE',  ( -2.841519077896158318, 5.566940434250007286, 4.736203831591942581 ) ) ;
#12724=CARTESIAN_POINT ( 'NONE',  ( 5.843318061569099164, -1.367618216965411637, 23.62696220972947359 ) ) ;
#12727=CARTESIAN_POINT ( 'NONE',  ( -5.558508435838188433, -2.857531096718933128, 5.130639327542137806 ) ) ;
#12728=CARTESIAN_POINT ( 'NONE',  ( -4.267992336621177607, -4.217442018460021202, 11.23805675996852216 ) ) ;
#12732=EDGE_CURVE ( 'NONE', #8051, #9247, #5533, .T. ) ;
#12733=ORIENTED_EDGE ( 'NONE', *, *, #15177, .T. ) ;
#12734=ORIENTED_EDGE ( 'NONE', *, *, #9801, .F. ) ;
#12736=CARTESIAN_POINT ( 'NONE',  ( 3.158296126777861978, -5.394094919772070007, 12.29887838423337953 ) ) ;
#12741=CARTESIAN_POINT ( 'NONE',  ( -5.935543223013861613, 0.8771126767606655106, 5.000000000000004441 ) ) ;
#12745=CARTESIAN_POINT ( 'NONE',  ( 5.531757352715618303, 2.326874507723293295, 18.87380682714709579 ) ) ;
#12747=CARTESIAN_POINT ( 'NONE',  ( -5.486741141153776091, -2.429871531109769389, 4.201117577520603774 ) ) ;
#12749=LINE ( 'NONE', #975, #7254 ) ;
#12751=VERTEX_POINT ( 'NONE', #1153 ) ;
#12753=ORIENTED_EDGE ( 'NONE', *, *, #9912, .T. ) ;
#12754=CARTESIAN_POINT ( 'NONE',  ( 4.290130679986631890, -4.545972905167674050, 5.615601928929212505 ) ) ;
#12755=CARTESIAN_POINT ( 'NONE',  ( 5.940390500375388072, 6.474944468551740329, 24.49999999999999289 ) ) ;
#12758=CARTESIAN_POINT ( 'NONE',  ( -5.487348639458843103, 2.428538342494515501, 17.19977782616120976 ) ) ;
#12759=FACE_BOUND ( 'NONE', #7639, .T. ) ;
#12763=CARTESIAN_POINT ( 'NONE',  ( 5.330189595673604508, 2.755293208590308573, 5.263826032055957782 ) ) ;
#12767=FACE_BOUND ( 'NONE', #13352, .T. ) ;
#12769=CARTESIAN_POINT ( 'NONE',  ( -5.935543223013841185, 0.8771126767608004027, 17.99999999999998934 ) ) ;
#12772=CARTESIAN_POINT ( 'NONE',  ( 2.817313151351004130, -5.579000502529524397, 24.49999999999999289 ) ) ;
#12773=DIRECTION ( 'NONE',  ( 1.000000000000000000, 0.000000000000000000, 0.000000000000000000 ) ) ;
#12774=EDGE_LOOP ( 'NONE', ( #14484, #9086, #6537, #11356 ) ) ;
#12776=B_SPLINE_CURVE_WITH_KNOTS ( 'NONE', 3,
 ( #3226, #762, #840, #9060, #10474, #2998, #4427, #2028, #7854, #13005, #15443, #14521, #2426, #3460, #9597, #10707, #6020, #15564 ),
 .UNSPECIFIED., .F., .F.,
 ( 4, 2, 2, 2, 2, 2, 2, 2, 4 ),
 ( 0.003131486019301990727, 0.003522824630466697433, 0.003914163241631404139, 0.004305501852796111278, 0.004696840463960818418, 0.005088179075125524690, 0.005479517686290231830, 0.005870856297454938102, 0.006262194908619645242 ),
 .UNSPECIFIED. ) ;
#12782=CYLINDRICAL_SURFACE ( 'NONE', #10637, 0.9999999999999998890 ) ;
#12785=CARTESIAN_POINT ( 'NONE',  ( 5.558508435838229289, -2.857531096718853192, 5.000000000000004441 ) ) ;
#12786=CARTESIAN_POINT ( 'NONE',  ( -5.726307184802674755, 2.506131700382416394, 4.199734849823247629 ) ) ;
#12787=CARTESIAN_POINT ( 'NONE',  ( -4.005361199354954493, -4.468319061418810634, 30.19977782616120621 ) ) ;
#12790=AXIS2_PLACEMENT_3D ( 'NONE', #5800, #8027, #5726 ) ;
#12791=CARTESIAN_POINT ( 'NONE',  ( -0.8737888311109246464, 5.936248257219519431, 12.00344185141216791 ) ) ;
#12793=EDGE_LOOP ( 'NONE', ( #4752, #985 ) ) ;
#12797=CARTESIAN_POINT ( 'NONE',  ( -3.634089073485356369, -4.776071126502746900, 5.999920023562623328 ) ) ;
#12799=CARTESIAN_POINT ( 'NONE',  ( 4.344265632482022355, 4.493596842505021449, 17.49574050496990552 ) ) ;
#12801=CARTESIAN_POINT ( 'NONE',  ( -6.176542424588100211, 0.9554180641286806885, 17.99999999999998934 ) ) ;
#12805=CARTESIAN_POINT ( 'NONE',  ( -2.817313151351109379, -5.579000502529471994, 5.000000000000004441 ) ) ;
#12806=CARTESIAN_POINT ( 'NONE',  ( -5.782947755040629190, -1.603807858344125092, 17.02601979877759319 ) ) ;
#12807=CARTESIAN_POINT ( 'NONE',  ( 4.286401442266496886, -4.198423832313229020, 17.99999999999998934 ) ) ;
#12811=VERTEX_POINT ( 'NONE', #9043 ) ;
#12812=CARTESIAN_POINT ( 'NONE',  ( 4.153440676704390988, -4.671190581744499859, 18.79954462468842280 ) ) ;
#12817=VECTOR ( 'NONE', #6457, 1000.000000000000114 ) ;
#12818=CARTESIAN_POINT ( 'NONE',  ( -3.882673863916292323, 4.899192824800937096, 31.97408542334170178 ) ) ;
#12819=CARTESIAN_POINT ( 'NONE',  ( 4.344313232726957352, 4.493553492990258746, 25.00436969680153965 ) ) ;
#12822=CARTESIAN_POINT ( 'NONE',  ( 5.330189595673665792, 2.755293208590188669, 18.26382603205595956 ) ) ;
#12825=CARTESIAN_POINT ( 'NONE',  ( -5.317509234263932072, -2.779225709351048401, 4.869383044678627925 ) ) ;
#12827=CARTESIAN_POINT ( 'NONE',  ( 3.159612573729133178, 5.393342049074686173, 18.80026515017675237 ) ) ;
#12828=EDGE_CURVE ( 'NONE', #11831, #3400, #8384, .T. ) ;
#12829=ORIENTED_EDGE ( 'NONE', *, *, #15078, .T. ) ;
#12831=CARTESIAN_POINT ( 'NONE',  ( 4.195842658231538458, -4.289229542213101709, 4.495602393557861731 ) ) ;
#12833=CARTESIAN_POINT ( 'NONE',  ( 4.153440676704494905, -4.671190581744405712, 5.799544624688432570 ) ) ;
#12835=CARTESIAN_POINT ( 'NONE',  ( -0.9999502950802086065, 5.916088184763882651, 5.131081491900111757 ) ) ;
#12836=EDGE_CURVE ( 'NONE', #13014, #8520, #15624, .T. ) ;
#12842=CARTESIAN_POINT ( 'NONE',  ( 3.010624175977970385, 5.190832888732223260, 4.201117577520603774 ) ) ;
#12845=LINE ( 'NONE', #1946, #142 ) ;
#12849=CARTESIAN_POINT ( 'NONE',  ( -5.903057025253901635, 1.078199533779546915, 18.61561732698604743 ) ) ;
#12853=CARTESIAN_POINT ( 'NONE',  ( -0.6156307853267388719, -5.969051238897275624, 25.29870573410680379 ) ) ;
#12856=CARTESIAN_POINT ( 'NONE',  ( -5.531623157106110966, 2.327208526676568745, 23.62635295315577011 ) ) ;
#12858=CARTESIAN_POINT ( 'NONE',  ( 6.021135683317731413, 1.680226122398092548, 25.47377282875267923 ) ) ;
#12860=CYLINDRICAL_SURFACE ( 'NONE', #1691, 1.000000000000000444 ) ;
#12864=CARTESIAN_POINT ( 'NONE',  ( -6.021167129161084652, 1.680051667990202446, 4.026404282766995024 ) ) ;
#12866=VERTEX_POINT ( 'NONE', #9664 ) ;
#12869=CARTESIAN_POINT ( 'NONE',  ( -0.8002302970945894822, 5.947135855825873563, 10.88601773212297985 ) ) ;
#12871=CARTESIAN_POINT ( 'NONE',  ( -2.668367453516892418, 5.373994336898001656, 24.49999999999999289 ) ) ;
#12873=CARTESIAN_POINT ( 'NONE',  ( -4.286401442266532413, -4.198423832313194382, 5.130616955321391615 ) ) ;
#12877=CARTESIAN_POINT ( 'NONE',  ( -0.8002720181888681728, 6.199262377003435631, 23.88606262465553343 ) ) ;
#12879=CARTESIAN_POINT ( 'NONE',  ( 2.668367453516645948, -5.373994336898125113, 11.36935038651143515 ) ) ;
#12884=CARTESIAN_POINT ( 'NONE',  ( -0.7988914244716894819, -5.947301735519300969, 17.38456289168617630 ) ) ;
#12885=ADVANCED_FACE ( 'NONE', ( #9578 ), #14419, .F. ) ;
#12886=AXIS2_PLACEMENT_3D ( 'NONE', #2376, #8677, #7243 ) ;
#12888=ORIENTED_EDGE ( 'NONE', *, *, #14007, .T. ) ;
#12889=EDGE_LOOP ( 'NONE', ( #10439, #13853 ) ) ;
#12890=CARTESIAN_POINT ( 'NONE',  ( 3.922396193918953777, -4.541970110199528676, 25.37380682714711000 ) ) ;
#12892=ORIENTED_EDGE ( 'NONE', *, *, #4384, .T. ) ;
#12897=EDGE_CURVE ( 'NONE', #9246, #5961, #1212, .T. ) ;
#12899=CARTESIAN_POINT ( 'NONE',  ( 2.030576276931546336E-13, 6.000000000000000888, 25.49999999999999645 ) ) ;
#12909=CARTESIAN_POINT ( 'NONE',  ( 3.254737477227878983, 5.337033878705280010, 18.87367328635991726 ) ) ;
#12913=ORIENTED_EDGE ( 'NONE', *, *, #12016, .T. ) ;
#12914=CARTESIAN_POINT ( 'NONE',  ( -4.416678568553792594, 4.422441866694168944, 17.73763026556123634 ) ) ;
#12916=CARTESIAN_POINT ( 'NONE',  ( -0.5039079366032412910, 5.980031194523151683, 4.126370681098134874 ) ) ;
#12919=CARTESIAN_POINT ( 'NONE',  ( -5.915653884842700272, 1.003805156977486401, 17.49560239355786351 ) ) ;
#12920=FACE_BOUND ( 'NONE', #430, .T. ) ;
#12921=CARTESIAN_POINT ( 'NONE',  ( 6.155912734541135301, -1.081577393120877861, 31.50389213124968890 ) ) ;
#12923=CARTESIAN_POINT ( 'NONE',  ( -2.668367453516648169, -5.373994336898123336, 31.00000000000000000 ) ) ;
#12928=FACE_BOUND ( 'NONE', #6132, .T. ) ;
#12930=CARTESIAN_POINT ( 'NONE',  ( -5.866923913994628315, 1.260079467906601858, 18.79952054102714243 ) ) ;
#12934=FACE_OUTER_BOUND ( 'NONE', #12349, .T. ) ;
#12937=ORIENTED_EDGE ( 'NONE', *, *, #13896, .T. ) ;
#12944=CYLINDRICAL_SURFACE ( 'NONE', #1474, 1.000000000000000666 ) ;
#12947=FACE_BOUND ( 'NONE', #5844, .T. ) ;
#12949=CARTESIAN_POINT ( 'NONE',  ( -2.782713018890577761, -5.315928322779191362, 30.49560239355785995 ) ) ;
#12952=CARTESIAN_POINT ( 'NONE',  ( -0.8736516769106251745, 5.936271176698245000, 10.99606771578675612 ) ) ;
#12954=ORIENTED_EDGE ( 'NONE', *, *, #3313, .T. ) ;
#12956=B_SPLINE_CURVE_WITH_KNOTS ( 'NONE', 3,
 ( #7091, #5896, #10743, #1420, #11136, #8611, #7480, #6222, #236, #4945, #3734, #1346, #10026, #2, #12089, #12246, #13446, #2624 ),
 .UNSPECIFIED., .F., .F.,
 ( 4, 2, 2, 2, 2, 2, 2, 2, 4 ),
 ( 0.000000000000000000, 0.0003914898357794950015, 0.0007829796715589900031, 0.001174469507338485059, 0.001565959343117980006, 0.001957449178897474520, 0.002348939014676968817, 0.002740428850456463113, 0.003131918686235957410 ),
 .UNSPECIFIED. ) ;
#12959=CARTESIAN_POINT ( 'NONE',  ( 5.935543223013889147, -0.8771126767604598973, 24.36938304467860306 ) ) ;
#12961=CARTESIAN_POINT ( 'NONE',  ( 3.011899281037459630, -5.190111395030252872, 10.69977782616120621 ) ) ;
#12965=DIRECTION ( 'NONE',  ( -0.5877852522924685852, -0.8090169943749508930, 0.000000000000000000 ) ) ;
#12966=EDGE_LOOP ( 'NONE', ( #1764, #10611, #417, #3122 ) ) ;
#12968=EDGE_LOOP ( 'NONE', ( #12664, #12489 ) ) ;
#12971=ORIENTED_EDGE ( 'NONE', *, *, #2290, .T. ) ;
#12974=CARTESIAN_POINT ( 'NONE',  ( -5.783239563508407954, -1.602707436861167789, 31.97358595436693918 ) ) ;
#12975=CARTESIAN_POINT ( 'NONE',  ( 4.290381260516126005, 4.545736887716346430, 25.11517780375843145 ) ) ;
#12978=DIRECTION ( 'NONE',  ( 0.5877852522924802425, -0.8090169943749422332, 0.000000000000000000 ) ) ;
#12984=VERTEX_POINT ( 'NONE', #3440 ) ;
#12986=ORIENTED_EDGE ( 'NONE', *, *, #2600, .F. ) ;
#12987=CARTESIAN_POINT ( 'NONE',  ( -4.435347140101170815, 4.403429997944372509, 17.99999999999998934 ) ) ;
#12989=CARTESIAN_POINT ( 'NONE',  ( -4.322356511625826236, 7.650514973136471220, 11.49999999999998224 ) ) ;
#12990=CARTESIAN_POINT ( 'NONE',  ( 6.176542424588110869, 0.9554180641286100784, 30.86936067245787996 ) ) ;
#12992=EDGE_CURVE ( 'NONE', #11779, #14829, #3076, .T. ) ;
#12993=CARTESIAN_POINT ( 'NONE',  ( 4.290130679986520867, 4.545972905167775302, 10.88439807107078572 ) ) ;
#12995=VECTOR ( 'NONE', #10620, 1000.000000000000000 ) ;
#12996=CARTESIAN_POINT ( 'NONE',  ( -3.255128505894364199, 5.336774832660688084, 12.37380055247394672 ) ) ;
#13001=DIRECTION ( 'NONE',  ( 0.9510565162951500895, 0.3090169943749582204, 0.000000000000000000 ) ) ;
#13005=CARTESIAN_POINT ( 'NONE',  ( 5.903472034603544749, -2.056448723545062585, 16.99991780678442410 ) ) ;
#13006=ADVANCED_FACE ( 'NONE', ( #12642 ), #9006, .F. ) ;
#13007=CARTESIAN_POINT ( 'NONE',  ( 0.1306070469495508313, 6.249999999999997335, 23.50000000000000000 ) ) ;
#13009=CARTESIAN_POINT ( 'NONE',  ( 5.935543223013849179, 0.8771126767607272390, 31.13061695532137918 ) ) ;
#13012=CARTESIAN_POINT ( 'NONE',  ( -4.344502777243695490, 4.493369211529107510, 25.00389213124970667 ) ) ;
#13013=CARTESIAN_POINT ( 'NONE',  ( -0.7995298244852583336, -5.947211616899275910, 25.11456014619857413 ) ) ;
#13014=VERTEX_POINT ( 'NONE', #1663 ) ;
#13015=CARTESIAN_POINT ( 'NONE',  ( -6.105861027178942635, 1.337741388557024624, 18.79954462468841925 ) ) ;
#13020=CARTESIAN_POINT ( 'NONE',  ( 5.859155363331436384, 2.178872204144837621, 25.47400098023329562 ) ) ;
#13024=CARTESIAN_POINT ( 'NONE',  ( 6.176542424588117086, 0.9554180641285650033, 11.36936067245785154 ) ) ;
#13025=DIRECTION ( 'NONE',  ( -0.5877852522924685852, -0.8090169943749508930, 0.000000000000000000 ) ) ;
#13026=CARTESIAN_POINT ( 'NONE',  ( -2.692215568229745948, -5.362327947133643136, 30.73770962164067200 ) ) ;
#13027=ORIENTED_EDGE ( 'NONE', *, *, #6399, .T. ) ;
#13029=EDGE_CURVE ( 'NONE', #4150, #10768, #10926, .T. ) ;
#13030=CARTESIAN_POINT ( 'NONE',  ( -0.2622916576875877759, 5.995491482261832594, 12.47384942646812078 ) ) ;
#13033=CARTESIAN_POINT ( 'NONE',  ( 4.435347140100995844, 4.403429997944549257, 31.00000000000000000 ) ) ;
#13034=EDGE_CURVE ( 'NONE', #13722, #721, #9085, .T. ) ;
#13038=CARTESIAN_POINT ( 'NONE',  ( 2.692335458626850642, -5.362264153667234190, 18.26239891805596827 ) ) ;
#13040=CARTESIAN_POINT ( 'NONE',  ( -6.105861027178951517, -1.337741388556972444, 4.200455375311574535 ) ) ;
#13042=CARTESIAN_POINT ( 'NONE',  ( 0.9999505860953618042, -6.169489349035804260, 31.13105903165812194 ) ) ;
#13044=VECTOR ( 'NONE', #6998, 1000.000000000000114 ) ;
#13045=CARTESIAN_POINT ( 'NONE',  ( 5.783198643800769645, 1.602922020054704078, 12.47377823943291375 ) ) ;
#13046=EDGE_LOOP ( 'NONE', ( #14296, #11541 ) ) ;
#13048=ORIENTED_EDGE ( 'NONE', *, *, #13374, .T. ) ;
#13051=EDGE_LOOP ( 'NONE', ( #7738, #10188 ) ) ;
#13053=CARTESIAN_POINT ( 'NONE',  ( -0.8736516769104770708, 5.936271176698266316, 23.99606771578674369 ) ) ;
#13054=LINE ( 'NONE', #9180, #1360 ) ;
#13057=VECTOR ( 'NONE', #14454, 1000.000000000000114 ) ;
#13058=CARTESIAN_POINT ( 'NONE',  ( 6.106056299406747101, -1.336851112280680098, 4.201121615766614248 ) ) ;
#13061=CARTESIAN_POINT ( 'NONE',  ( 2.996417732210646889, -5.485687819086863648, 4.386038205919295940 ) ) ;
#13064=ORIENTED_EDGE ( 'NONE', *, *, #1934, .F. ) ;
#13065=DIRECTION ( 'NONE',  ( 0.000000000000000000, 0.000000000000000000, -1.000000000000000000 ) ) ;
#13068=CARTESIAN_POINT ( 'NONE',  ( 2.094888806938587637E-14, 6.250000000000000888, 30.00000000000000000 ) ) ;
#13069=AXIS2_PLACEMENT_3D ( 'NONE', #4127, #12634, #5569 ) ;
#13070=CARTESIAN_POINT ( 'NONE',  ( -3.634089073485525123, -4.776071126502616337, 25.49992002356260912 ) ) ;
#13074=CARTESIAN_POINT ( 'NONE',  ( -0.5030929395818275474, -6.230885867001161316, 23.62600319116548775 ) ) ;
#13075=CARTESIAN_POINT ( 'NONE',  ( -3.781065399486035261, -4.978303713186424950, 18.99991741810288559 ) ) ;
#13076=CARTESIAN_POINT ( 'NONE',  ( 1.353717517954364224E-13, -6.000000000000000888, 18.99999999999998934 ) ) ;
#13078=( NAMED_UNIT ( * ) PLANE_ANGLE_UNIT ( ) SI_UNIT ( $, .RADIAN. ) );
#13079=CARTESIAN_POINT ( 'NONE',  ( 5.317509234263932072, 2.779225709351047957, 5.132360785839114925 ) ) ;
#13084=CARTESIAN_POINT ( 'NONE',  ( -6.021167129161020704, -1.680051667990425379, 18.97359571723300320 ) ) ;
#13085=EDGE_CURVE ( 'NONE', #5746, #6892, #13758, .T. ) ;
#13087=ORIENTED_EDGE ( 'NONE', *, *, #5524, .T. ) ;
#13090=CARTESIAN_POINT ( 'NONE',  ( 0.9735856429313511917, -5.920699391845015924, 11.76285283906725354 ) ) ;
#13091=CARTESIAN_POINT ( 'NONE',  ( -0.7988914244716200930, -5.947301735519313404, 23.88456289168616919 ) ) ;
#13092=ORIENTED_EDGE ( 'NONE', *, *, #2206, .F. ) ;
#13093=DIRECTION ( 'NONE',  ( 0.000000000000000000, 1.000000000000000000, 0.000000000000000000 ) ) ;
#13094=CYLINDRICAL_SURFACE ( 'NONE', #772, 1.000000000000000888 ) ;
#13095=ORIENTED_EDGE ( 'NONE', *, *, #11539, .F. ) ;
#13096=CARTESIAN_POINT ( 'NONE',  ( -5.935543223013830527, 0.8771126767608677932, 24.36760611998364823 ) ) ;
#13102=EDGE_CURVE ( 'NONE', #2089, #902, #7256, .T. ) ;
#13103=FACE_BOUND ( 'NONE', #1442, .T. ) ;
#13105=CARTESIAN_POINT ( 'NONE',  ( -3.420659742068319353, -4.931142898501779115, 30.00004946353777058 ) ) ;
#13108=CARTESIAN_POINT ( 'NONE',  ( -0.5044069930202613739, 5.979990686695000335, 12.37335743227902718 ) ) ;
#13113=CARTESIAN_POINT ( 'NONE',  ( 5.746619684944291429, 1.730157667110781672, 16.99995067926686687 ) ) ;
#13115=CARTESIAN_POINT ( 'NONE',  ( 4.286401442266437378, 4.198423832313292969, 18.13239388001634467 ) ) ;
#13117=CARTESIAN_POINT ( 'NONE',  ( -6.176542424588105540, -0.9554180641286327269, 5.000000000000004441 ) ) ;
#13119=CARTESIAN_POINT ( 'NONE',  ( 4.322356511625595310, 7.650514973136599117, 11.49999999999998224 ) ) ;
#13121=CYLINDRICAL_SURFACE ( 'NONE', #3633, 0.9999999999999998890 ) ;
#13124=ORIENTED_EDGE ( 'NONE', *, *, #9282, .T. ) ;
#13126=ORIENTED_EDGE ( 'NONE', *, *, #7594, .F. ) ;
#13130=ORIENTED_EDGE ( 'NONE', *, *, #13196, .T. ) ;
#13133=CARTESIAN_POINT ( 'NONE',  ( -5.842945980534652861, -1.369128644668926809, 31.87378430870261425 ) ) ;
#13135=CARTESIAN_POINT ( 'NONE',  ( 3.883716939928917977, 4.898343590941304448, 25.47359571723300675 ) ) ;
#13138=CARTESIAN_POINT ( 'NONE',  ( 6.081836621194441683, -1.445163676684824594, 4.126941084456995590 ) ) ;
#13140=CARTESIAN_POINT ( 'NONE',  ( 3.568242062701607598, -5.132954954975453177, 3.999950931234679263 ) ) ;
#13142=CARTESIAN_POINT ( 'NONE',  ( 4.286401442266518202, 4.198423832313208592, 31.00000000000000000 ) ) ;
#13143=ORIENTED_EDGE ( 'NONE', *, *, #14842, .F. ) ;
#13145=CARTESIAN_POINT ( 'NONE',  ( 2.692143549875480435, -5.362363179736437502, 4.738056759968539922 ) ) ;
#13147=ORIENTED_EDGE ( 'NONE', *, *, #8639, .F. ) ;
#13149=CARTESIAN_POINT ( 'NONE',  ( 0.6144300524833891108, 6.220417338033052523, 30.20033372175935327 ) ) ;
#13151=CARTESIAN_POINT ( 'NONE',  ( 3.107278289587155573, -5.134157760522071179, 17.12635295315575235 ) ) ;
#13152=CARTESIAN_POINT ( 'NONE',  ( 0.7993401192311868630, -6.199366368793663540, 5.614832469365748757 ) ) ;
#13153=ORIENTED_EDGE ( 'NONE', *, *, #2168, .F. ) ;
#13154=CARTESIAN_POINT ( 'NONE',  ( -5.317509234263906315, 2.779225709351095475, 17.99999999999998934 ) ) ;
#13156=CARTESIAN_POINT ( 'NONE',  ( 2.668367453516444776, 5.373994336898222812, 24.49999999999999289 ) ) ;
#13159=CARTESIAN_POINT ( 'NONE',  ( 5.409274167810628420, 2.597759609440700057, 30.38480617551148910 ) ) ;
#13160=CYLINDRICAL_SURFACE ( 'NONE', #5667, 0.9999999999999998890 ) ;
#13165=CARTESIAN_POINT ( 'NONE',  ( 3.107278289587176445, 5.134157760522058744, 31.87364704684422634 ) ) ;
#13167=ORIENTED_EDGE ( 'NONE', *, *, #5722, .T. ) ;
#13168=CARTESIAN_POINT ( 'NONE',  ( -5.842988226680567720, 1.369004370660693137, 12.37380682714709756 ) ) ;
#13169=CARTESIAN_POINT ( 'NONE',  ( -0.5042987395406965945, -5.979983180450083147, 12.37329304179975509 ) ) ;
#13170=CIRCLE ( 'NONE', #464, 6.000000000000000888 ) ;
#13172=VERTEX_POINT ( 'NONE', #11686 ) ;
#13176=CARTESIAN_POINT ( 'NONE',  ( -5.782947755040658500, -1.603807858344011406, 30.02601979877761096 ) ) ;
#13177=EDGE_CURVE ( 'NONE', #10924, #398, #3247, .T. ) ;
#13181=CARTESIAN_POINT ( 'NONE',  ( -5.769755079862307845, 2.405651898699003421, 12.37305891554298931 ) ) ;
#13183=CARTESIAN_POINT ( 'NONE',  ( -2.841041022017386286, 5.567186575787263614, 5.262252817217141221 ) ) ;
#13187=LINE ( 'NONE', #14539, #14607 ) ;
#13190=EDGE_LOOP ( 'NONE', ( #10616, #14421 ) ) ;
#13194=ORIENTED_EDGE ( 'NONE', *, *, #10709, .F. ) ;
#13195=CARTESIAN_POINT ( 'NONE',  ( -3.011139120916454637, -5.190534000030377904, 4.200681937418262457 ) ) ;
#13196=EDGE_CURVE ( 'NONE', #567, #12426, #3429, .T. ) ;
#13198=CARTESIAN_POINT ( 'NONE',  ( 5.843075991566581529, -1.368655265451063086, 5.873647046844242325 ) ) ;
#13200=VECTOR ( 'NONE', #514, 1000.000000000000114 ) ;
#13202=CARTESIAN_POINT ( 'NONE',  ( 0.7988860301923105256, 6.199427171881326082, 10.88455580536195377 ) ) ;
#13204=B_SPLINE_CURVE_WITH_KNOTS ( 'NONE', 3,
 ( #7446, #2751, #8807, #8891, #8968, #12290, #10073, #4014, #5065, #14771, #5384, #6345, #13636, #6578, #10153, #9998, #7679, #11412 ),
 .UNSPECIFIED., .F., .F.,
 ( 4, 2, 2, 2, 2, 2, 2, 2, 4 ),
 ( 0.000000000000000000, 0.0003914357524127465640, 0.0007828715048254931280, 0.001174307257238239692, 0.001565743009650986256, 0.001957178762063731519, 0.002348614514476477216, 0.002740050266889222479, 0.003131486019301968175 ),
 .UNSPECIFIED. ) ;
#13205=CARTESIAN_POINT ( 'NONE',  ( 2.782156709077369339, -5.316215864844073380, 18.50312048902377526 ) ) ;
#13207=CARTESIAN_POINT ( 'NONE',  ( 3.421280866381160024, -4.930711975950901937, 10.49995067926686687 ) ) ;
#13208=CARTESIAN_POINT ( 'NONE',  ( 5.329945432499622271, -2.755769831645151324, 31.26229037835932090 ) ) ;
#13210=CARTESIAN_POINT ( 'NONE',  ( 5.329945432499570757, 2.755769831645247692, 4.737709621640687985 ) ) ;
#13211=CARTESIAN_POINT ( 'NONE',  ( 5.487097279078438028, 2.429065649168800523, 12.29952054102714243 ) ) ;
#13214=VERTEX_POINT ( 'NONE', #8031 ) ;
#13219=CARTESIAN_POINT ( 'NONE',  ( -5.531623157106149158, -2.327208526676475930, 31.87364704684421923 ) ) ;
#13220=DIRECTION ( 'NONE',  ( 0.000000000000000000, 0.000000000000000000, 1.000000000000000000 ) ) ;
#13222=EDGE_CURVE ( 'NONE', #8130, #13429, #6500, .T. ) ;
#13224=CARTESIAN_POINT ( 'NONE',  ( -5.531209434046356677, 2.328189801702577277, 31.87303779027051576 ) ) ;
#13227=CARTESIAN_POINT ( 'NONE',  ( 4.069684453406360092, -4.744965295353502199, 30.12619944752604439 ) ) ;
#13231=B_SPLINE_CURVE_WITH_KNOTS ( 'NONE', 3,
 ( #14513, #6175, #11089, #3689, #8489, #6011, #1068, #10853, #15719, #13317, #7286, #34, #4899, #7127, #8567, #7360, #11012, #14344 ),
 .UNSPECIFIED., .F., .F.,
 ( 4, 2, 2, 2, 2, 2, 2, 2, 4 ),
 ( 0.003131918686235948303, 0.003523310662250241174, 0.003914702638264534046, 0.004306094614278826484, 0.004697486590293120656, 0.005088878566307413961, 0.005480270542321708134, 0.005871662518336002307, 0.006263054494350295612 ),
 .UNSPECIFIED. ) ;
#13234=EDGE_LOOP ( 'NONE', ( #10746, #10109, #11445, #11776 ) ) ;
#13235=ORIENTED_EDGE ( 'NONE', *, *, #10297, .F. ) ;
#13236=CARTESIAN_POINT ( 'NONE',  ( -5.984759433606971157, 1.806271833852423070, 25.50008219321556524 ) ) ;
#13237=CARTESIAN_POINT ( 'NONE',  ( -4.416837305303585204, -4.422286678978921692, 24.23809786915986919 ) ) ;
#13238=CARTESIAN_POINT ( 'NONE',  ( 0.2622538972264162327, -6.245673238944476680, 5.973859943692001906 ) ) ;
#13239=CARTESIAN_POINT ( 'NONE',  ( -5.726307184802632122, -2.506131700382510985, 31.80026515017676658 ) ) ;
#13240=CARTESIAN_POINT ( 'NONE',  ( -0.1306070469493368635, -6.249999999999999112, 4.000000000000003553 ) ) ;
#13242=CARTESIAN_POINT ( 'NONE',  ( -4.416837305303549677, 4.422286678978957219, 11.76190213084010239 ) ) ;
#13243=CARTESIAN_POINT ( 'NONE',  ( -5.984759433606947177, -1.806271833852501674, 23.49991780678443476 ) ) ;
#13244=CARTESIAN_POINT ( 'NONE',  ( -2.782769401326143477, -5.315896561274865206, 31.50428920362020335 ) ) ;
#13251=CARTESIAN_POINT ( 'NONE',  ( 4.435347140100914132, 4.403429997944631857, 17.99999999999998934 ) ) ;
#13252=B_SPLINE_CURVE_WITH_KNOTS ( 'NONE', 3,
 ( #7736, #12584, #6169, #8637, #14672, #13469, #7428, #4314, #6556, #14164, #15373, #5594, #15137, #571, #1916, #15214, #804, #496 ),
 .UNSPECIFIED., .F., .F.,
 ( 4, 2, 2, 2, 2, 2, 2, 2, 4 ),
 ( 0.003131486019302004171, 0.003522824630466709142, 0.003914163241631414547, 0.004305501852796119085, 0.004696840463960824490, 0.005088179075125529027, 0.005479517686290234432, 0.005870856297454939837, 0.006262194908619644375 ),
 .UNSPECIFIED. ) ;
#13259=LINE ( 'NONE', #13415, #3094 ) ;
#13262=CARTESIAN_POINT ( 'NONE',  ( -0.9740012993919970885, -6.173846968979643357, 31.26164920628438892 ) ) ;
#13270=ORIENTED_EDGE ( 'NONE', *, *, #14566, .T. ) ;
#13273=CARTESIAN_POINT ( 'NONE',  ( 6.780834062235653815E-14, 6.000000000000000888, 10.49999999999998224 ) ) ;
#13275=CARTESIAN_POINT ( 'NONE',  ( -2.668367453516814258, -5.373994336898041624, 24.36760611998364467 ) ) ;
#13279=CARTESIAN_POINT ( 'NONE',  ( 0.5042675786779380331, 6.230788509548837339, 12.37331068310448678 ) ) ;
#13281=CARTESIAN_POINT ( 'NONE',  ( 3.633127580202223150, -4.776802569231096030, 19.00007961174475213 ) ) ;
#13286=CARTESIAN_POINT ( 'NONE',  ( 5.486982057989152395, 2.429327048029968683, 4.200681937418260681 ) ) ;
#13287=CARTESIAN_POINT ( 'NONE',  ( 5.317509234263963158, 2.779225709350988449, 11.63236078583908650 ) ) ;
#13293=VERTEX_POINT ( 'NONE', #3403 ) ;
#13294=CARTESIAN_POINT ( 'NONE',  ( -2.692215568229873401, 5.362327947133580075, 11.76229037835932978 ) ) ;
#13295=ORIENTED_EDGE ( 'NONE', *, *, #10002, .T. ) ;
#13298=CARTESIAN_POINT ( 'NONE',  ( 6.172614129015227213, 0.9817721000789304542, 31.26236973443873879 ) ) ;
#13302=CARTESIAN_POINT ( 'NONE',  ( -5.330004929009606762, 2.755647751839361170, 31.26239891805596827 ) ) ;
#13304=CARTESIAN_POINT ( 'NONE',  ( 4.416779112813693509, -4.422345839825757352, 30.73774718278283302 ) ) ;
#13310=ORIENTED_EDGE ( 'NONE', *, *, #13510, .F. ) ;
#13311=CARTESIAN_POINT ( 'NONE',  ( -5.558508435838135142, 2.857531096719037489, 24.49999999999999289 ) ) ;
#13316=CARTESIAN_POINT ( 'NONE',  ( 6.780834062235653815E-14, 6.000000000000000888, 10.49999999999998224 ) ) ;
#13317=CARTESIAN_POINT ( 'NONE',  ( -3.420311045507815617, -4.931422832349310781, 12.50007961174474502 ) ) ;
#13319=CARTESIAN_POINT ( 'NONE',  ( 0.1323933160976972501, -6.000000000000000000, 18.99999999999998934 ) ) ;
#13324=CARTESIAN_POINT ( 'NONE',  ( 5.317509234263963158, 2.779225709350988449, 11.49999999999998224 ) ) ;
#13328=VERTEX_POINT ( 'NONE', #7950 ) ;
#13330=CARTESIAN_POINT ( 'NONE',  ( 0.6139908388541727158, -5.969238533166604022, 10.69977627912011187 ) ) ;
#13331=CARTESIAN_POINT ( 'NONE',  ( 5.317509234264027107, 2.779225709350867213, 24.63236078583910071 ) ) ;
#13333=CARTESIAN_POINT ( 'NONE',  ( 2.817313151351127587, -5.579000502529462224, 11.49999999999998224 ) ) ;
#13335=CARTESIAN_POINT ( 'NONE',  ( 3.566234721237914407, 5.134387337253918382, 23.50008258189710375 ) ) ;
#13337=AXIS2_PLACEMENT_3D ( 'NONE', #6246, #7660, #9899 ) ;
#13339=FACE_OUTER_BOUND ( 'NONE', #11164, .T. ) ;
#13340=CARTESIAN_POINT ( 'NONE',  ( -0.5030929395820097350, -6.230885867001147993, 30.12600319116549485 ) ) ;
#13345=CARTESIAN_POINT ( 'NONE',  ( 5.649053410273092268, 2.675685104943213766, 17.38482219624156855 ) ) ;
#13349=DIRECTION ( 'NONE',  ( 0.5877852522924802425, -0.8090169943749422332, 0.000000000000000000 ) ) ;
#13350=VECTOR ( 'NONE', #10555, 1000.000000000000114 ) ;
#13352=EDGE_LOOP ( 'NONE', ( #5200, #6030 ) ) ;
#13354=LINE ( 'NONE', #12162, #2640 ) ;
#13357=CARTESIAN_POINT ( 'NONE',  ( 4.142173849413805620, -4.341773579105349334, 30.38480617551148910 ) ) ;
#13360=CARTESIAN_POINT ( 'NONE',  ( -5.935543223013850955, 0.8771126767607324570, 11.49999999999998224 ) ) ;
#13361=CARTESIAN_POINT ( 'NONE',  ( -2.997753866155832725, 5.484939622623836719, 30.38439807107077684 ) ) ;
#13366=ORIENTED_EDGE ( 'NONE', *, *, #1640, .T. ) ;
#13367=CARTESIAN_POINT ( 'NONE',  ( -5.487348639458788035, -2.428538342494640290, 25.30022217383879024 ) ) ;
#13374=EDGE_CURVE ( 'NONE', #15059, #471, #15593, .T. ) ;
#13376=CARTESIAN_POINT ( 'NONE',  ( -5.859221468178898107, -2.178708437343367166, 25.47408542334170534 ) ) ;
#13382=ORIENTED_EDGE ( 'NONE', *, *, #6976, .F. ) ;
#13383=ORIENTED_EDGE ( 'NONE', *, *, #445, .F. ) ;
#13385=ORIENTED_EDGE ( 'NONE', *, *, #12732, .F. ) ;
#13386=CARTESIAN_POINT ( 'NONE',  ( -5.769755079862290081, -2.405651898699045610, 30.12694108445699825 ) ) ;
#13387=ADVANCED_FACE ( 'NONE', ( #14468 ), #14711, .F. ) ;
#13390=CARTESIAN_POINT ( 'NONE',  ( -5.648794263291781803, 2.676232015153535926, 31.61441947245485196 ) ) ;
#13393=CARTESIAN_POINT ( 'NONE',  ( 4.344313232727033736, -4.493553492990184139, 23.99563030319847456 ) ) ;
#13394=CARTESIAN_POINT ( 'NONE',  ( 2.030576276931546336E-13, -6.250000000000000888, 25.49999999999999645 ) ) ;
#13397=CARTESIAN_POINT ( 'NONE',  ( -5.615811513734916716, -2.743665920700641525, 23.99691356133952524 ) ) ;
#13404=CARTESIAN_POINT ( 'NONE',  ( 5.931828553037968632, 0.9033193133619482618, 11.23805675996852571 ) ) ;
#13409=CARTESIAN_POINT ( 'NONE',  ( -5.665308849928823776, 1.980336949702511173, 12.49992002356259668 ) ) ;
#13410=CARTESIAN_POINT ( 'NONE',  ( 0.1323933160976290824, -6.000000000000000000, 12.49999999999998579 ) ) ;
#13411=CARTESIAN_POINT ( 'NONE',  ( 5.531757352715640508, 2.326874507723235563, 25.37380682714710645 ) ) ;
#13412=CARTESIAN_POINT ( 'NONE',  ( 4.435347140101058905, -4.403429997944485308, 31.13234125634170368 ) ) ;
#13415=CARTESIAN_POINT ( 'NONE',  ( 1.353717517954364224E-13, -6.250000000000000888, 18.99999999999998934 ) ) ;
#13416=AXIS2_PLACEMENT_3D ( 'NONE', #230, #72, #1261 ) ;
#13418=CARTESIAN_POINT ( 'NONE',  ( -4.435347140101218777, 4.403429997944323659, 24.49999999999999289 ) ) ;
#13420=EDGE_CURVE ( 'NONE', #3400, #11314, #4853, .T. ) ;
#13421=CARTESIAN_POINT ( 'NONE',  ( -6.105861027178951517, 1.337741388556971778, 12.29954462468842458 ) ) ;
#13424=FACE_BOUND ( 'NONE', #9856, .T. ) ;
#13427=CARTESIAN_POINT ( 'NONE',  ( 5.570760634536900291, -2.834026536768054605, 24.76225281721715987 ) ) ;
#13428=ADVANCED_FACE ( 'NONE', ( #2209 ), #10732, .F. ) ;
#13429=VERTEX_POINT ( 'NONE', #13273 ) ;
#13434=CARTESIAN_POINT ( 'NONE',  ( 4.286401442266448925, -4.198423832313278758, 24.63236078583909716 ) ) ;
#13445=CARTESIAN_POINT ( 'NONE',  ( 5.915755444410815578, -1.003187219519776852, 10.99687951097621408 ) ) ;
#13446=CARTESIAN_POINT ( 'NONE',  ( -5.317509234263939177, 2.779225709351034634, 11.36935038651144758 ) ) ;
#13448=CARTESIAN_POINT ( 'NONE',  ( 2.668367453516444776, 5.373994336898222812, 24.49999999999999289 ) ) ;
#13450=ORIENTED_EDGE ( 'NONE', *, *, #11539, .T. ) ;
#13456=CARTESIAN_POINT ( 'NONE',  ( -5.648559266344491903, -2.676764518776009627, 12.11396179408069784 ) ) ;
#13462=CARTESIAN_POINT ( 'NONE',  ( 4.005998022989971652, 4.467726698309252065, 5.799318062581741984 ) ) ;
#13464=CARTESIAN_POINT ( 'NONE',  ( -5.903843691985246167, 2.055287728870609509, 29.99995093123466816 ) ) ;
#13469=CARTESIAN_POINT ( 'NONE',  ( -5.725684683139582454, -2.507514573674833880, 10.70112161576659915 ) ) ;
#13471=CARTESIAN_POINT ( 'NONE',  ( 2.817313151351108047, 5.579000502529472882, 5.000000000000004441 ) ) ;
#13472=CARTESIAN_POINT ( 'NONE',  ( 0.1323408341374891217, 6.250000000000000888, 6.000000000000006217 ) ) ;
#13473=CARTESIAN_POINT ( 'NONE',  ( -5.903061651806624788, 2.057626436184726515, 31.99991741810289625 ) ) ;
#13474=CARTESIAN_POINT ( 'NONE',  ( 0.8730424326981676142, 5.936362132114451740, 10.99500690218562937 ) ) ;
#13476=CARTESIAN_POINT ( 'NONE',  ( 5.329945432499647140, -2.755769831645103363, 11.76229037835932800 ) ) ;
#13477=CARTESIAN_POINT ( 'NONE',  ( -6.142908455506942644, -1.155755562476059817, 5.615177803758428787 ) ) ;
#13482=EDGE_CURVE ( 'NONE', #6460, #3929, #14635, .T. ) ;
#13485=EDGE_CURVE ( 'NONE', #1423, #13328, #2850, .T. ) ;
#13486=CARTESIAN_POINT ( 'NONE',  ( -2.668367453516709009, 5.373994336898094026, 5.132393880016356214 ) ) ;
#13489=CARTESIAN_POINT ( 'NONE',  ( 3.780072143464270784, -4.979057943639705996, 32.00008219321556169 ) ) ;
#13491=CARTESIAN_POINT ( 'NONE',  ( 3.458623254138554870, 5.207221900902925249, 23.52622717124731011 ) ) ;
#13493=CARTESIAN_POINT ( 'NONE',  ( 5.487097279078438916, -2.429065649168797858, 4.200479458972859348 ) ) ;
#13494=CARTESIAN_POINT ( 'NONE',  ( -5.558508435838198203, 2.857531096718914476, 11.49999999999998224 ) ) ;
#13499=CARTESIAN_POINT ( 'NONE',  ( 6.768587589771821120E-14, -6.000000000000000888, 12.49999999999998401 ) ) ;
#13504=CARTESIAN_POINT ( 'NONE',  ( -5.666074146197956907, -1.978051345703274011, 19.00004932073311181 ) ) ;
#13505=CARTESIAN_POINT ( 'NONE',  ( 4.153440676704409640, 4.671190581744483872, 30.20045537531156654 ) ) ;
#13508=CARTESIAN_POINT ( 'NONE',  ( 5.570760634536812361, -2.834026536768229576, 31.26225281721713145 ) ) ;
#13509=CARTESIAN_POINT ( 'NONE',  ( 0.2637975869347859437, 6.245592211692893692, 12.47332839949191197 ) ) ;
#13510=EDGE_CURVE ( 'NONE', #1465, #6001, #4774, .T. ) ;
#13513=VECTOR ( 'NONE', #7450, 1000.000000000000114 ) ;
#13514=CARTESIAN_POINT ( 'NONE',  ( 5.558508435838221295, 2.857531096718871844, 11.49999999999998224 ) ) ;
#13517=CARTESIAN_POINT ( 'NONE',  ( 1.353717517954364224E-13, -6.250000000000000888, 18.99999999999998934 ) ) ;
#13518=EDGE_CURVE ( 'NONE', #5609, #2306, #3802, .T. ) ;
#13519=CARTESIAN_POINT ( 'NONE',  ( 3.735808404764840329, 4.696639218303251262, 23.52601979877760030 ) ) ;
#13520=ORIENTED_EDGE ( 'NONE', *, *, #7856, .T. ) ;
#13522=ORIENTED_EDGE ( 'NONE', *, *, #10127, .T. ) ;
#13523=ORIENTED_EDGE ( 'NONE', *, *, #4466, .T. ) ;
#13524=EDGE_CURVE ( 'NONE', #15573, #2516, #6102, .T. ) ;
#13526=B_SPLINE_CURVE_WITH_KNOTS ( 'NONE', 3,
 ( #10956, #4921, #1091, #13340, #216, #14778, #2525, #3864, #7454, #10881, #13262, #9615, #2443, #2280, #8425, #4842, #3711, #1246 ),
 .UNSPECIFIED., .F., .F.,
 ( 4, 2, 2, 2, 2, 2, 2, 2, 4 ),
 ( 0.003131490185286079676, 0.003522829482338674534, 0.003914168779391269393, 0.004305508076443864685, 0.004696847373496459976, 0.005088186670549064809, 0.005479525967601669642, 0.005870865264654275342, 0.006262204561706881042 ),
 .UNSPECIFIED. ) ;
#13530=CARTESIAN_POINT ( 'NONE',  ( -6.021167129161037579, -1.680051667990365871, 12.47359571723300142 ) ) ;
#13532=FACE_OUTER_BOUND ( 'NONE', #14006, .T. ) ;
#13538=AXIS2_PLACEMENT_3D ( 'NONE', #7189, #254, #14741 ) ;
#13539=CARTESIAN_POINT ( 'NONE',  ( -6.105925084677703119, 1.337450587213082631, 30.20066851092422411 ) ) ;
#13543=ORIENTED_EDGE ( 'NONE', *, *, #158, .T. ) ;
#13544=CARTESIAN_POINT ( 'NONE',  ( 0.1306171417089971032, 5.999999999999999112, 16.99999999999998224 ) ) ;
#13546=CARTESIAN_POINT ( 'NONE',  ( 0.6156133477426871670, 6.220296490279942248, 5.798723873455116973 ) ) ;
#13547=CARTESIAN_POINT ( 'NONE',  ( 0.9999505860954734926, -6.169489349035784720, 18.13105903165811839 ) ) ;
#13548=CARTESIAN_POINT ( 'NONE',  ( 6.768587589771821120E-14, 6.000000000000000888, 12.49999999999998401 ) ) ;
#13551=CARTESIAN_POINT ( 'NONE',  ( -6.142844459177253746, 1.156093792145113319, 5.615601928929211617 ) ) ;
#13559=ORIENTED_EDGE ( 'NONE', *, *, #4590, .T. ) ;
#13561=CARTESIAN_POINT ( 'NONE',  ( -7.180990026460740694, -3.384707322287537679, 31.00000000000000000 ) ) ;
#13562=CARTESIAN_POINT ( 'NONE',  ( -4.286401442266736694, 4.198423832312983883, 24.36938304467860661 ) ) ;
#13563=CARTESIAN_POINT ( 'NONE',  ( 0.9999196734184672142, 5.916093360767482601, 24.36725955955066425 ) ) ;
#13565=DIRECTION ( 'NONE',  ( -0.3090169943749447867, -0.9510565162951544194, 0.000000000000000000 ) ) ;
#13567=CARTESIAN_POINT ( 'NONE',  ( 5.747343991580192046, -1.727858744772256427, 4.000079976437387330 ) ) ;
#13569=LINE ( 'NONE', #5235, #5207 ) ;
#13572=EDGE_CURVE ( 'NONE', #15526, #8395, #8179, .T. ) ;
#13573=CARTESIAN_POINT ( 'NONE',  ( 6.176542424588109093, 0.9554180641286111886, 31.00000000000000000 ) ) ;
#13575=CARTESIAN_POINT ( 'NONE',  ( 4.416779112813599362, 4.422345839825853275, 11.76225281721714744 ) ) ;
#13580=EDGE_LOOP ( 'NONE', ( #2224, #5306, #6321, #4394 ) ) ;
#13581=CARTESIAN_POINT ( 'NONE',  ( -3.632151824461103740, -4.777505256984581727, 16.99995067926686332 ) ) ;
#13583=CARTESIAN_POINT ( 'NONE',  ( 6.020822430078820453, -1.681351817312314090, 12.47408542334169113 ) ) ;
#13585=ADVANCED_FACE ( 'NONE', ( #13891 ), #5710, .F. ) ;
#13587=CARTESIAN_POINT ( 'NONE',  ( 3.010624175977864692, 5.190832888732285433, 17.20111757752057002 ) ) ;
#13589=B_SPLINE_CURVE_WITH_KNOTS ( 'NONE', 3,
 ( #8506, #2439, #11982, #12063, #12143, #4916, #6114, #10952, #12218, #50, #1317, #3552, #4755, #14775, #128, #14616, #1088, #9845 ),
 .UNSPECIFIED., .F., .F.,
 ( 4, 2, 2, 2, 2, 2, 2, 2, 4 ),
 ( 0.003131918686235978661, 0.003523310662250268930, 0.003914702638264559199, 0.004306094614278849902, 0.004697486590293139738, 0.005088878566307429574, 0.005480270542321720277, 0.005871662518336010980, 0.006263054494350300816 ),
 .UNSPECIFIED. ) ;
#13593=CARTESIAN_POINT ( 'NONE',  ( -5.866984344570825627, -1.259800266528668500, 12.29931806258173488 ) ) ;
#13598=ORIENTED_EDGE ( 'NONE', *, *, #5981, .T. ) ;
#13599=CARTESIAN_POINT ( 'NONE',  ( -5.330004929009483305, -2.755647751839598758, 24.23760108194402108 ) ) ;
#13601=CARTESIAN_POINT ( 'NONE',  ( -4.143041610105492545, 4.340967609746855693, 25.11397738943081848 ) ) ;
#13604=CARTESIAN_POINT ( 'NONE',  ( -6.172639027853106697, -0.9816353142772318296, 11.76225281721714389 ) ) ;
#13606=CARTESIAN_POINT ( 'NONE',  ( -0.7993401192310704007, 6.199366368793674198, 25.11483246936562352 ) ) ;
#13609=CARTESIAN_POINT ( 'NONE',  ( -6.172639027853085381, -0.9816353142773684981, 24.76225281721715987 ) ) ;
#13611=EDGE_CURVE ( 'NONE', #10768, #2588, #12339, .T. ) ;
#13612=CYLINDRICAL_SURFACE ( 'NONE', #14725, 1.000000000000000000 ) ;
#13616=ORIENTED_EDGE ( 'NONE', *, *, #12447, .F. ) ;
#13617=ORIENTED_EDGE ( 'NONE', *, *, #9643, .T. ) ;
#13618=CARTESIAN_POINT ( 'NONE',  ( 5.931793676715097163, -0.9035324301688445470, 30.73760108194402818 ) ) ;
#13621=CARTESIAN_POINT ( 'NONE',  ( -0.7995298244854599501, -5.947211616899247488, 5.614560146198585677 ) ) ;
#13622=CARTESIAN_POINT ( 'NONE',  ( 2.082642335314403343E-14, -6.000000000000000888, 32.00000000000000000 ) ) ;
#13623=CARTESIAN_POINT ( 'NONE',  ( 2.817313151351004574, -5.579000502529524397, 24.36936067245787996 ) ) ;
#13624=CARTESIAN_POINT ( 'NONE',  ( 5.903472034603510110, -2.056448723545162505, 29.99991780678443476 ) ) ;
#13627=CARTESIAN_POINT ( 'NONE',  ( -4.416678568553742856, 4.422441866694219570, 11.23763026556121858 ) ) ;
#13635=CARTESIAN_POINT ( 'NONE',  ( -5.648559266344497232, 2.676764518775994528, 17.38603820591928439 ) ) ;
#13636=CARTESIAN_POINT ( 'NONE',  ( 3.159612573729244200, -5.393342049074621336, 10.69973484982323697 ) ) ;
#13637=CARTESIAN_POINT ( 'NONE',  ( 0.9999505860954052139, -6.169489349035797154, 11.63105903165811839 ) ) ;
#13638=CARTESIAN_POINT ( 'NONE',  ( 5.649053410273044307, 2.675685104943319459, 30.38482219624157565 ) ) ;
#13640=FACE_BOUND ( 'NONE', #7662, .T. ) ;
#13642=CARTESIAN_POINT ( 'NONE',  ( -4.435347140101219665, 4.403429997944324548, 24.36939309276499799 ) ) ;
#13644=CARTESIAN_POINT ( 'NONE',  ( 5.531757352715557019, 2.326874507723430519, 5.873806827147107334 ) ) ;
#13646=FACE_BOUND ( 'NONE', #10728, .T. ) ;
#13647=VECTOR ( 'NONE', #12122, 1000.000000000000114 ) ;
#13650=CARTESIAN_POINT ( 'NONE',  ( 6.105747081304222945, -1.338335777572041474, 25.30026515017674882 ) ) ;
#13653=CARTESIAN_POINT ( 'NONE',  ( -5.531623157106109190, -2.327208526676572298, 18.87364704684421923 ) ) ;
#13656=VERTEX_POINT ( 'NONE', #5787 ) ;
#13660=CARTESIAN_POINT ( 'NONE',  ( 5.931828553037973961, -0.9033193133619329407, 5.261943240031468960 ) ) ;
#13663=DIRECTION ( 'NONE',  ( -0.9510565162951545304, 0.3090169943749447867, 0.000000000000000000 ) ) ;
#13669=CARTESIAN_POINT ( 'NONE',  ( 5.985119669071172765, -1.805077827356371900, 23.50008258189710020 ) ) ;
#13670=LINE ( 'NONE', #3887, #11594 ) ;
#13671=CARTESIAN_POINT ( 'NONE',  ( 4.286401442266389417, 4.198423832313341819, 24.36763921416088863 ) ) ;
#13672=CARTESIAN_POINT ( 'NONE',  ( -5.620879908643967582, 2.102487719021896684, 12.47377823943291375 ) ) ;
#13675=ORIENTED_EDGE ( 'NONE', *, *, #6103, .F. ) ;
#13681=EDGE_LOOP ( 'NONE', ( #3738, #9822 ) ) ;
#13682=VECTOR ( 'NONE', #7717, 1000.000000000000114 ) ;
#13685=ADVANCED_FACE ( 'NONE', ( #12934 ), #3080, .F. ) ;
#13687=DIRECTION ( 'NONE',  ( 0.5877852522924802425, -0.8090169943749422332, 0.000000000000000000 ) ) ;
#13690=CARTESIAN_POINT ( 'NONE',  ( -4.006441409774819995, 4.467329318258138393, 17.20111757752057713 ) ) ;
#13692=CARTESIAN_POINT ( 'NONE',  ( 4.195795028115099079, -4.289273350251257888, 31.50428920362021046 ) ) ;
#13694=CARTESIAN_POINT ( 'NONE',  ( -6.142908455506956855, 1.155755562475991427, 30.38482219624157565 ) ) ;
#13697=ORIENTED_EDGE ( 'NONE', *, *, #92, .T. ) ;
#13698=VECTOR ( 'NONE', #5251, 1000.000000000000114 ) ;
#13700=EDGE_LOOP ( 'NONE', ( #9684, #10207 ) ) ;
#13702=CARTESIAN_POINT ( 'NONE',  ( 4.416397290909912954, 4.422724436066427067, 4.736203831591939917 ) ) ;
#13703=EDGE_LOOP ( 'NONE', ( #10304, #9459 ) ) ;
#13704=CARTESIAN_POINT ( 'NONE',  ( -0.6144377077729846759, -5.969178481556066451, 4.200339668577364627 ) ) ;
#13707=CARTESIAN_POINT ( 'NONE',  ( -2.817313151351206635, 5.579000502529421368, 31.13237410716304865 ) ) ;
#13709=CARTESIAN_POINT ( 'NONE',  ( 5.770288754215132876, -2.404361317819945221, 30.12618035954928075 ) ) ;
#13711=FILL_AREA_STYLE ('',( #3182 ) ) ;
#13712=DIRECTION ( 'NONE',  ( 0.000000000000000000, 0.000000000000000000, -1.000000000000000000 ) ) ;
#13713=AXIS2_PLACEMENT_3D ( 'NONE', #14108, #591, #5769 ) ;
#13714=CARTESIAN_POINT ( 'NONE',  ( 3.311576095066511183, 5.004818610361351006, 10.52622176056705072 ) ) ;
#13722=VERTEX_POINT ( 'NONE', #13251 ) ;
#13725=CARTESIAN_POINT ( 'NONE',  ( -0.5043776560897343941, 6.230795654995838539, 5.873374762960125395 ) ) ;
#13726=CARTESIAN_POINT ( 'NONE',  ( 0.6156307853271528741, 5.969051238897232103, 25.29870573410679668 ) ) ;
#13731=CARTESIAN_POINT ( 'NONE',  ( -2.997753866155750568, -5.484939622623882016, 31.61560192892922672 ) ) ;
#13734=CARTESIAN_POINT ( 'NONE',  ( -2.841041022017330331, -5.567186575787293812, 30.73774718278283302 ) ) ;
#13740=LINE ( 'NONE', #5082, #12651 ) ;
#13742=CARTESIAN_POINT ( 'NONE',  ( -2.668367453516831134, 5.373994336898032742, 18.13239388001634467 ) ) ;
#13745=CARTESIAN_POINT ( 'NONE',  ( 4.286401442266532413, 4.198423832313196158, 5.000000000000004441 ) ) ;
#13746=LINE ( 'NONE', #2614, #6049 ) ;
#13748=LINE ( 'NONE', #1574, #13698 ) ;
#13750=DIRECTION ( 'NONE',  ( 0.000000000000000000, 1.000000000000000000, 0.000000000000000000 ) ) ;
#13752=CARTESIAN_POINT ( 'NONE',  ( -3.011385983131386723, 5.190390249166400238, 30.20047945897283270 ) ) ;
#13757=VERTEX_POINT ( 'NONE', #1155 ) ;
#13758=LINE ( 'NONE', #14807, #9873 ) ;
#13759=ORIENTED_EDGE ( 'NONE', *, *, #11965, .T. ) ;
#13760=DIRECTION ( 'NONE',  ( 0.8090169943749421222, 0.5877852522924802425, 0.000000000000000000 ) ) ;
#13764=CARTESIAN_POINT ( 'NONE',  ( -2.997753866155803415, 5.484939622623852706, 4.384398071070799929 ) ) ;
#13766=FACE_OUTER_BOUND ( 'NONE', #12561, .T. ) ;
#13769=DIRECTION ( 'NONE',  ( -0.3090169943749579429, 0.9510565162951502005, 0.000000000000000000 ) ) ;
#13770=EDGE_CURVE ( 'NONE', #11747, #8394, #3046, .T. ) ;
#13773=CARTESIAN_POINT ( 'NONE',  ( 0.000000000000000000, 6.250000000000000888, 32.00000000000000000 ) ) ;
#13774=EDGE_CURVE ( 'NONE', #9246, #12662, #4286, .T. ) ;
#13780=CARTESIAN_POINT ( 'NONE',  ( 5.616089948629690021, 2.743103014345625645, 4.495630303198470124 ) ) ;
#13781=ORIENTED_EDGE ( 'NONE', *, *, #748, .T. ) ;
#13783=CARTESIAN_POINT ( 'NONE',  ( 0.1306497350717528982, -6.000000000000000000, 30.00000000000000355 ) ) ;
#13784=CARTESIAN_POINT ( 'NONE',  ( -4.344502777243570257, 4.493369211529226526, 31.50389213124969601 ) ) ;
#13787=VECTOR ( 'NONE', #10939, 1000.000000000000114 ) ;
#13789=CARTESIAN_POINT ( 'NONE',  ( -4.435347140101170815, 4.403429997944372509, 17.99999999999998934 ) ) ;
#13798=CARTESIAN_POINT ( 'NONE',  ( -5.558508435838135142, 2.857531096719037489, 24.49999999999999289 ) ) ;
#13799=CARTESIAN_POINT ( 'NONE',  ( -2.668367453516892418, 5.373994336898002544, 24.36763921416089218 ) ) ;
#13801=FACE_OUTER_BOUND ( 'NONE', #6814, .T. ) ;
#13802=CARTESIAN_POINT ( 'NONE',  ( -3.159082487394730521, -5.393634094348361607, 31.79954462468843346 ) ) ;
#13803=EDGE_CURVE ( 'NONE', #4625, #15036, #9603, .T. ) ;
#13805=CARTESIAN_POINT ( 'NONE',  ( 2.848727059636034120, 5.281416301279857173, 4.385574784280629856 ) ) ;
#13812=CARTESIAN_POINT ( 'NONE',  ( 3.883716939929014345, 4.898343590941228065, 12.47359571723299965 ) ) ;
#13815=CARTESIAN_POINT ( 'NONE',  ( -4.286401442266689621, 4.198423832313033621, 18.13064961348853998 ) ) ;
#13820=B_SPLINE_CURVE_WITH_KNOTS ( 'NONE', 3,
 ( #9554, #950, #14392, #8123, #9314, #5585, #15283, #2218, #1030, #13207, #5737, #10660, #12961, #8283, #2061, #11768, #12879, #10581 ),
 .UNSPECIFIED., .F., .F.,
 ( 4, 2, 2, 2, 2, 2, 2, 2, 4 ),
 ( 0.000000000000000000, 0.0003914898357794966278, 0.0007829796715589932557, 0.001174469507338489829, 0.001565959343117987596, 0.001957449178897484494, 0.002348939014676980960, 0.002740428850456477425, 0.003131918686235973890 ),
 .UNSPECIFIED. ) ;
#13825=CARTESIAN_POINT ( 'NONE',  ( -5.487348639458879518, -2.428538342494442226, 5.800222173838808892 ) ) ;
#13827=CARTESIAN_POINT ( 'NONE',  ( 5.558508435838229289, -2.857531096718852748, 5.132374107163055754 ) ) ;
#13832=B_SPLINE_CURVE_WITH_KNOTS ( 'NONE', 3,
 ( #14318, #9487, #2077, #3425, #11782, #11708, #8296, #6950, #3351, #3512, #15457, #884, #965, #10523, #5752, #6874, #10596, #7102 ),
 .UNSPECIFIED., .F., .F.,
 ( 4, 2, 2, 2, 2, 2, 2, 2, 4 ),
 ( 0.000000000000000000, 0.0003914904498596245754, 0.0007829808997192491508, 0.001174471349578873726, 0.001565961799438498302, 0.001957452249298123094, 0.002348942699157747453, 0.002740433149017371811, 0.003131923598876996603 ),
 .UNSPECIFIED. ) ;
#13835=VECTOR ( 'NONE', #1364, 1000.000000000000114 ) ;
#13836=ORIENTED_EDGE ( 'NONE', *, *, #4036, .T. ) ;
#13837=DIRECTION ( 'NONE',  ( 0.5877852522924802425, -0.8090169943749422332, 0.000000000000000000 ) ) ;
#13840=CARTESIAN_POINT ( 'NONE',  ( -2.782769401326126157, -5.315896561274875864, 5.504289203620205129 ) ) ;
#13847=CARTESIAN_POINT ( 'NONE',  ( 2.782468714962335277, 5.316055268221454355, 12.00389795015984795 ) ) ;
#13848=ORIENTED_EDGE ( 'NONE', *, *, #12828, .F. ) ;
#13849=ORIENTED_EDGE ( 'NONE', *, *, #15126, .T. ) ;
#13850=VERTEX_POINT ( 'NONE', #2350 ) ;
#13851=CARTESIAN_POINT ( 'NONE',  ( 3.158296126777787372, -5.394094919772115304, 18.79887838423338309 ) ) ;
#13853=ORIENTED_EDGE ( 'NONE', *, *, #13774, .T. ) ;
#13854=AXIS2_PLACEMENT_3D ( 'NONE', #522, #12538, #3940 ) ;
#13855=CARTESIAN_POINT ( 'NONE',  ( 5.935543223013881153, -0.8771126767605277319, 18.13064961348853998 ) ) ;
#13859=CARTESIAN_POINT ( 'NONE',  ( 6.021135683317704768, -1.680226122398187583, 30.02622717124732077 ) ) ;
#13861=CARTESIAN_POINT ( 'NONE',  ( 5.935543223013869607, -0.8771126767605967878, 11.49999999999998224 ) ) ;
#13867=EDGE_LOOP ( 'NONE', ( #4316, #1800, #15451, #2272 ) ) ;
#13868=EDGE_CURVE ( 'NONE', #13014, #8921, #7612, .T. ) ;
#13869=CARTESIAN_POINT ( 'NONE',  ( 4.286401442266591921, -4.198423832313133985, 4.867606119983652668 ) ) ;
#13870=VERTEX_POINT ( 'NONE', #7522 ) ;
#13871=CARTESIAN_POINT ( 'NONE',  ( 4.416397290909979567, -4.422724436066356901, 5.263796168408045872 ) ) ;
#13872=EDGE_CURVE ( 'NONE', #6892, #8289, #3996, .T. ) ;
#13873=DIRECTION ( 'NONE',  ( -0.5877852522924685852, -0.8090169943749507819, 0.000000000000000000 ) ) ;
#13874=CARTESIAN_POINT ( 'NONE',  ( 1.000049271338558032, -6.169473353325540366, 11.36969612704552546 ) ) ;
#13875=CARTESIAN_POINT ( 'NONE',  ( 0.7988914244720274338, 5.947301735519258337, 23.88456289168618341 ) ) ;
#13877=CARTESIAN_POINT ( 'NONE',  ( 2.782468714962265555, -5.316055268221492547, 23.99610204984018580 ) ) ;
#13880=CARTESIAN_POINT ( 'NONE',  ( -3.107583187530371660, -5.133966411712722611, 31.87380682714712066 ) ) ;
#13882=CARTESIAN_POINT ( 'NONE',  ( 6.780834057763294634E-14, -6.250000000000000888, 10.49999999999998224 ) ) ;
#13886=CYLINDRICAL_SURFACE ( 'NONE', #2713, 6.000000000000000888 ) ;
#13888=CARTESIAN_POINT ( 'NONE',  ( -4.070051655338084551, -4.744673454622494901, 10.62632671364005077 ) ) ;
#13891=FACE_OUTER_BOUND ( 'NONE', #2784, .T. ) ;
#13894=CARTESIAN_POINT ( 'NONE',  ( -3.420659742068413944, -4.931142898501715166, 17.00004946353775992 ) ) ;
#13895=CARTESIAN_POINT ( 'NONE',  ( 3.632753594129150887, 4.777047695051116705, 25.49995053646222232 ) ) ;
#13896=EDGE_CURVE ( 'NONE', #9247, #1121, #3930, .T. ) ;
#13901=CARTESIAN_POINT ( 'NONE',  ( -5.558508435838157347, -2.857531096718993080, 11.49999999999998224 ) ) ;
#13903=DIRECTION ( 'NONE',  ( 0.9510565162951499785, 0.3090169943749582204, 0.000000000000000000 ) ) ;
#13904=CARTESIAN_POINT ( 'NONE',  ( 6.172614129015267181, -0.9817721000786672203, 24.23763026556124700 ) ) ;
#13905=CARTESIAN_POINT ( 'NONE',  ( -5.558508435838229289, 2.857531096718854524, 5.000000000000004441 ) ) ;
#13906=LINE ( 'NONE', #14876, #5950 ) ;
#13911=CARTESIAN_POINT ( 'NONE',  ( -5.782947755040631854, 1.603807858344106441, 25.47398020122238549 ) ) ;
#13913=ORIENTED_EDGE ( 'NONE', *, *, #9736, .F. ) ;
#13914=CARTESIAN_POINT ( 'NONE',  ( -4.322356511625880415, 7.650514973136431252, 17.99999999999998934 ) ) ;
#13918=EDGE_CURVE ( 'NONE', #8844, #5961, #13170, .T. ) ;
#13919=CARTESIAN_POINT ( 'NONE',  ( 5.747343991580251554, -1.727858744772061916, 23.50007997643738022 ) ) ;
#13921=CARTESIAN_POINT ( 'NONE',  ( -5.570722351696259622, -2.834100162821977520, 5.261902130840119263 ) ) ;
#13922=CARTESIAN_POINT ( 'NONE',  ( -3.632151824461037570, -4.777505256984632354, 10.49995067926685977 ) ) ;
#13923=FACE_OUTER_BOUND ( 'NONE', #15076, .T. ) ;
#13926=CARTESIAN_POINT ( 'NONE',  ( 3.107278289587142694, 5.134157760522080061, 12.37364704684420857 ) ) ;
#13928=ORIENTED_EDGE ( 'NONE', *, *, #5208, .T. ) ;
#13931=CARTESIAN_POINT ( 'NONE',  ( 2.668367453516524712, -5.373994336898185509, 24.63061695532138629 ) ) ;
#13933=ORIENTED_EDGE ( 'NONE', *, *, #13177, .F. ) ;
#13934=CARTESIAN_POINT ( 'NONE',  ( 5.375886393124439167, -2.665038680141179395, 18.50439760644211518 ) ) ;
#13937=CARTESIAN_POINT ( 'NONE',  ( -0.2619041840693476231, 6.245686665308508800, 17.02605849433793495 ) ) ;
#13940=CYLINDRICAL_SURFACE ( 'NONE', #4461, 1.000000000000000666 ) ;
#13941=CARTESIAN_POINT ( 'NONE',  ( 5.665707375537479606, 1.979196487016660955, 19.00007961174475568 ) ) ;
#13943=AXIS2_PLACEMENT_3D ( 'NONE', #2753, #11183, #1391 ) ;
#13944=AXIS2_PLACEMENT_3D ( 'NONE', #14297, #10500, #8035 ) ;
#13945=CARTESIAN_POINT ( 'NONE',  ( -5.665308849928819335, -1.980336949702520721, 4.000079976437387330 ) ) ;
#13947=CARTESIAN_POINT ( 'NONE',  ( 2.996417732210459484, 5.485687819086964900, 18.61396179408071561 ) ) ;
#13951=CARTESIAN_POINT ( 'NONE',  ( 2.817313151351187983, -5.579000502529432026, 5.000000000000004441 ) ) ;
#13953=AXIS2_PLACEMENT_3D ( 'NONE', #8833, #13663, #9220 ) ;
#13954=CARTESIAN_POINT ( 'NONE',  ( -7.180990026460726483, -3.384707322287581199, 11.49999999999998224 ) ) ;
#13955=CARTESIAN_POINT ( 'NONE',  ( 5.858736126997189153, 2.179962889276912286, 23.52640428276698614 ) ) ;
#13956=AXIS2_PLACEMENT_3D ( 'NONE', #8602, #2374, #1105 ) ;
#13957=B_SPLINE_CURVE_WITH_KNOTS ( 'NONE', 3,
 ( #6188, #13410, #4912, #9769, #12058, #1083, #5944, #13090, #3465, #9604, #6025, #15648, #14443, #13330, #8417, #8501, #15571, #5864 ),
 .UNSPECIFIED., .F., .F.,
 ( 4, 2, 2, 2, 2, 2, 2, 2, 4 ),
 ( 0.000000000000000000, 0.0003914904498596249007, 0.0007829808997192496929, 0.001174471349578874377, 0.001565961799438498952, 0.001957452249298123528, 0.002348942699157748754, 0.002740433149017373546, 0.003131923598876997904 ),
 .UNSPECIFIED. ) ;
#13960=CARTESIAN_POINT ( 'NONE',  ( 6.176542424588124192, -0.9554180641285233699, 31.13063932754212360 ) ) ;
#13962=CARTESIAN_POINT ( 'NONE',  ( -4.196288036172386882, -4.288789315524898171, 31.50312048902376105 ) ) ;
#13965=EDGE_CURVE ( 'NONE', #8394, #11747, #12018, .T. ) ;
#13968=FACE_BOUND ( 'NONE', #10535, .T. ) ;
#13969=CARTESIAN_POINT ( 'NONE',  ( 6.155973317223295105, -1.081218830693672972, 30.49691356133954301 ) ) ;
#13971=B_SPLINE_CURVE_WITH_KNOTS ( 'NONE', 3,
 ( #15395, #9344, #14185, #5461, #8155, #2414, #4652, #983, #1063, #15712, #14589, #13151, #10692, #5927, #10930, #3444, #8484, #9504 ),
 .UNSPECIFIED., .F., .F.,
 ( 4, 2, 2, 2, 2, 2, 2, 2, 4 ),
 ( 0.000000000000000000, 0.0003914898357794971157, 0.0007829796715589942314, 0.001174469507338491347, 0.001565959343117987379, 0.001957449178897484061, 0.002348939014676979659, 0.002740428850456476124, 0.003131918686235972155 ),
 .UNSPECIFIED. ) ;
#13974=CARTESIAN_POINT ( 'NONE',  ( -2.817313151351372724, 5.579000502529338767, 24.49999999999999289 ) ) ;
#13976=CARTESIAN_POINT ( 'NONE',  ( -0.1306171417086578468, -6.000000000000006217, 23.50000000000000000 ) ) ;
#13977=VERTEX_POINT ( 'NONE', #203 ) ;
#13978=FACE_OUTER_BOUND ( 'NONE', #7559, .T. ) ;
#13979=CARTESIAN_POINT ( 'NONE',  ( 5.487097279078491319, -2.429065649168680174, 17.20047945897285047 ) ) ;
#13983=LINE ( 'NONE', #11439, #7065 ) ;
#13984=DIRECTION ( 'NONE',  ( -0.5877852522924685852, -0.8090169943749508930, 0.000000000000000000 ) ) ;
#13986=CARTESIAN_POINT ( 'NONE',  ( 5.616116467183726257, -2.743044348085402540, 23.99574050496988065 ) ) ;
#13988=DIRECTION ( 'NONE',  ( -0.5877852522924685852, -0.8090169943749508930, 0.000000000000000000 ) ) ;
#13989=ORIENTED_EDGE ( 'NONE', *, *, #10999, .F. ) ;
#13991=AXIS2_PLACEMENT_3D ( 'NONE', #4434, #9368, #8256 ) ;
#13994=DIRECTION ( 'NONE',  ( 0.000000000000000000, 1.000000000000000000, 0.000000000000000000 ) ) ;
#13996=CARTESIAN_POINT ( 'NONE',  ( 5.531796221294892568, 2.326749136277177499, 17.12621569129737509 ) ) ;
#13998=CARTESIAN_POINT ( 'NONE',  ( -0.1306394121197269609, 6.250000000000005329, 23.49999999999999289 ) ) ;
#14003=CYLINDRICAL_SURFACE ( 'NONE', #15369, 1.000000000000000666 ) ;
#14004=CARTESIAN_POINT ( 'NONE',  ( 4.416779112813637553, 4.422345839825811531, 31.26225281721713856 ) ) ;
#14006=EDGE_LOOP ( 'NONE', ( #8791, #10928, #14586, #6925 ) ) ;
#14007=EDGE_CURVE ( 'NONE', #159, #15355, #6344, .T. ) ;
#14009=ORIENTED_EDGE ( 'NONE', *, *, #1670, .F. ) ;
#14011=CARTESIAN_POINT ( 'NONE',  ( 2.668367453516524268, -5.373994336898184621, 24.49999999999999289 ) ) ;
#14013=B_SPLINE_CURVE_WITH_KNOTS ( 'NONE', 3,
 ( #8081, #7546, #5389, #15087, #7845, #9129, #9431, #4580, #13075, #2175, #11964, #1224, #8160, #5775, #5932, #1146, #7287, #5854 ),
 .UNSPECIFIED., .F., .F.,
 ( 4, 2, 2, 2, 2, 2, 2, 2, 4 ),
 ( 0.003131486019301977283, 0.003522824630466687024, 0.003914163241631397200, 0.004305501852796106074, 0.004696840463960814949, 0.005088179075125523823, 0.005479517686290232698, 0.005870856297454941572, 0.006262194908619650446 ),
 .UNSPECIFIED. ) ;
#14014=ORIENTED_EDGE ( 'NONE', *, *, #5939, .T. ) ;
#14015=CARTESIAN_POINT ( 'NONE',  ( 5.620786884546348006, -2.102685372472733683, 18.97358595436693207 ) ) ;
#14018=CARTESIAN_POINT ( 'NONE',  ( -4.070051655338123631, 4.744673454622464703, 31.87367328635992791 ) ) ;
#14022=CARTESIAN_POINT ( 'NONE',  ( -4.152999119458083754, 4.671604476854259502, 18.80026515017675237 ) ) ;
#14025=VECTOR ( 'NONE', #5659, 1000.000000000000000 ) ;
#14029=ORIENTED_EDGE ( 'NONE', *, *, #12828, .T. ) ;
#14030=EDGE_LOOP ( 'NONE', ( #1526, #1761, #12734, #3021 ) ) ;
#14031=CARTESIAN_POINT ( 'NONE',  ( 4.435347140101073116, -4.403429997944471985, 5.132341256341692137 ) ) ;
#14036=CARTESIAN_POINT ( 'NONE',  ( 4.153440676704393653, 4.671190581744498083, 10.70045537531157365 ) ) ;
#14037=FACE_BOUND ( 'NONE', #8499, .T. ) ;
#14038=CARTESIAN_POINT ( 'NONE',  ( 3.254737477227961584, -5.337033878705229384, 17.12632671364005077 ) ) ;
#14044=FACE_BOUND ( 'NONE', #6653, .T. ) ;
#14045=CARTESIAN_POINT ( 'NONE',  ( 0.5030929395822668626, 6.230885867001124900, 23.62600319116549841 ) ) ;
#14048=CARTESIAN_POINT ( 'NONE',  ( -4.435347140101220553, 4.403429997944323659, 24.63063932754212360 ) ) ;
#14049=CARTESIAN_POINT ( 'NONE',  ( -1.000079958707936756, -5.916066267613731888, 24.63152738882033432 ) ) ;
#14050=ORIENTED_EDGE ( 'NONE', *, *, #3366, .T. ) ;
#14052=ADVANCED_FACE ( 'NONE', ( #15312 ), #4335, .F. ) ;
#14053=CARTESIAN_POINT ( 'NONE',  ( -5.915653884842686061, 1.003805156977559676, 23.99560239355785640 ) ) ;
#14056=DIRECTION ( 'NONE',  ( 0.5877852522924802425, -0.8090169943749422332, 0.000000000000000000 ) ) ;
#14059=CARTESIAN_POINT ( 'NONE',  ( 6.172651332693092741, 0.9815532474593937629, 11.23809786915985853 ) ) ;
#14060=EDGE_CURVE ( 'NONE', #11314, #11875, #1786, .T. ) ;
#14063=ORIENTED_EDGE ( 'NONE', *, *, #6146, .F. ) ;
#14065=CARTESIAN_POINT ( 'NONE',  ( -0.9735856429312097493, 5.920699391845040793, 11.76285283906727841 ) ) ;
#14068=EDGE_CURVE ( 'NONE', #13757, #3740, #5578, .T. ) ;
#14069=CARTESIAN_POINT ( 'NONE',  ( -3.107583187530343682, -5.133966411712735933, 5.873806827147109111 ) ) ;
#14070=CARTESIAN_POINT ( 'NONE',  ( 7.490007020835692586, -2.433650805992223720, 31.00000000000000000 ) ) ;
#14072=( LENGTH_UNIT ( ) NAMED_UNIT ( * ) SI_UNIT ( .MILLI., .METRE. ) );
#14073=CARTESIAN_POINT ( 'NONE',  ( -3.255013540813561423, -5.336859797930882721, 5.873819640450717472 ) ) ;
#14075=CARTESIAN_POINT ( 'NONE',  ( -5.558508435838189321, -2.857531096718932684, 4.869393092765017528 ) ) ;
#14077=CARTESIAN_POINT ( 'NONE',  ( -5.558508435838096950, -2.857531096719117425, 24.63063932754212715 ) ) ;
#14078=CARTESIAN_POINT ( 'NONE',  ( -5.935543223013826974, -0.8771126767608833363, 17.86763921416087442 ) ) ;
#14084=CARTESIAN_POINT ( 'NONE',  ( 3.633127580202175189, -4.776802569231135109, 25.50007961174476634 ) ) ;
#14090=CARTESIAN_POINT ( 'NONE',  ( 6.021135683317711873, 1.680226122398159161, 18.97377282875267213 ) ) ;
#14091=CARTESIAN_POINT ( 'NONE',  ( 1.353717517954364224E-13, 6.000000000000000888, 18.99999999999998934 ) ) ;
#14093=EDGE_CURVE ( 'NONE', #13172, #4668, #5535, .T. ) ;
#14095=B_SPLINE_CURVE_WITH_KNOTS ( 'NONE', 3,
 ( #10021, #1414, #11130, #1183, #5093, #4939, #3881, #9791, #14640, #1341, #9944, #7548, #6055, #12395, #1494, #6372, #11206, #4860 ),
 .UNSPECIFIED., .F., .F.,
 ( 4, 2, 2, 2, 2, 2, 2, 2, 4 ),
 ( 0.003131490185286089217, 0.003522829482338690147, 0.003914168779391291077, 0.004305508076443891573, 0.004696847373496492069, 0.005088186670549092565, 0.005479525967601693928, 0.005870865264654294424, 0.006262204561706894920 ),
 .UNSPECIFIED. ) ;
#14100=EDGE_CURVE ( 'NONE', #4730, #11432, #11833, .T. ) ;
#14104=AXIS2_PLACEMENT_3D ( 'NONE', #8646, #1540, #14679 ) ;
#14106=CARTESIAN_POINT ( 'NONE',  ( 2.817313151351188871, -5.579000502529433803, 5.130606907234995795 ) ) ;
#14108=CARTESIAN_POINT ( 'NONE',  ( 7.490007020835728113, -2.433650805992114918, 17.99999999999998934 ) ) ;
#14109=CARTESIAN_POINT ( 'NONE',  ( 6.020822430078827558, 1.681351817312285668, 23.52591457665828756 ) ) ;
#14111=CARTESIAN_POINT ( 'NONE',  ( 3.780072143464171752, 4.979057943639783268, 10.49991780678442410 ) ) ;
#14112=DIRECTION ( 'NONE',  ( -1.000000000000000000, 0.000000000000000000, 0.000000000000000000 ) ) ;
#14116=CARTESIAN_POINT ( 'NONE',  ( -4.435347140101154828, -4.403429997944389385, 24.63060690723497714 ) ) ;
#14120=DIRECTION ( 'NONE',  ( -0.9510565162951544194, 0.3090169943749447312, 0.000000000000000000 ) ) ;
#14121=CARTESIAN_POINT ( 'NONE',  ( -5.486741141153758328, 2.429871531109806249, 18.79888242247939800 ) ) ;
#14124=CARTESIAN_POINT ( 'NONE',  ( 3.780072143464118906, -4.979057943639823236, 25.50008219321556879 ) ) ;
#14128=DIRECTION ( 'NONE',  ( 0.5877852522924802425, -0.8090169943749422332, 0.000000000000000000 ) ) ;
#14140=CARTESIAN_POINT ( 'NONE',  ( -3.632151824461010925, -4.777505256984653670, 29.99995067926689174 ) ) ;
#14143=EDGE_CURVE ( 'NONE', #12751, #15454, #14706, .T. ) ;
#14145=ORIENTED_EDGE ( 'NONE', *, *, #6110, .F. ) ;
#14152=CARTESIAN_POINT ( 'NONE',  ( -4.290821322214329214, -4.545321419741597424, 5.614419472454843962 ) ) ;
#14157=CARTESIAN_POINT ( 'NONE',  ( 4.069684453406294367, 4.744965295353559043, 31.87380055247396271 ) ) ;
#14158=CARTESIAN_POINT ( 'NONE',  ( -0.9737778612004134304, -5.920671847850539571, 17.73736375884649519 ) ) ;
#14160=EDGE_CURVE ( 'NONE', #1022, #8273, #2351, .T. ) ;
#14162=ORIENTED_EDGE ( 'NONE', *, *, #10606, .T. ) ;
#14163=EDGE_LOOP ( 'NONE', ( #14162, #6554, #6185, #7778 ) ) ;
#14164=CARTESIAN_POINT ( 'NONE',  ( -5.984759433606990697, -1.806271833852358011, 10.49991780678442232 ) ) ;
#14165=CARTESIAN_POINT ( 'NONE',  ( -3.420659742068434817, 4.931142898501699179, 12.49995053646221166 ) ) ;
#14166=ORIENTED_EDGE ( 'NONE', *, *, #11861, .F. ) ;
#14170=CARTESIAN_POINT ( 'NONE',  ( -5.408775798201155283, -2.598833957129672800, 31.61397738943081492 ) ) ;
#14171=CARTESIAN_POINT ( 'NONE',  ( -2.931156713028388427, -5.520271803279265477, 4.495630303198470124 ) ) ;
#14184=CARTESIAN_POINT ( 'NONE',  ( -0.8738043859790136647, 6.188821459035888317, 12.00341560223746207 ) ) ;
#14185=CARTESIAN_POINT ( 'NONE',  ( 4.267936573529204303, -4.217499624512243805, 17.73770962164069331 ) ) ;
#14188=CARTESIAN_POINT ( 'NONE',  ( -5.931817299736841242, 0.9033986943602623221, 17.73770962164069331 ) ) ;
#14190=AXIS2_PLACEMENT_3D ( 'NONE', #704, #6694, #5576 ) ;
#14191=CARTESIAN_POINT ( 'NONE',  ( 0.000000000000000000, 0.000000000000000000, 53.67766952966368876 ) ) ;
#14192=CARTESIAN_POINT ( 'NONE',  ( -3.158825713737595020, 5.393784879207108141, 12.29933148907576346 ) ) ;
#14194=CARTESIAN_POINT ( 'NONE',  ( 1.354942164390165777E-13, -6.250000000000000888, 16.99999999999998579 ) ) ;
#14201=AXIS2_PLACEMENT_3D ( 'NONE', #6680, #11513, #1651 ) ;
#14204=CARTESIAN_POINT ( 'NONE',  ( 4.069800786343695798, -4.744882212776915686, 25.37381964045071925 ) ) ;
#14205=CARTESIAN_POINT ( 'NONE',  ( 5.317509234264064411, -2.779225709350791274, 24.49999999999999289 ) ) ;
#14207=CARTESIAN_POINT ( 'NONE',  ( -6.020865209844581400, 1.681180471732190984, 18.97400098023329562 ) ) ;
#14211=CARTESIAN_POINT ( 'NONE',  ( 5.903472034603542085, 2.056448723545071022, 25.50008219321556524 ) ) ;
#14212=CARTESIAN_POINT ( 'NONE',  ( -7.490007020835684592, -2.433650805992431110, 11.49999999999998224 ) ) ;
#14213=CARTESIAN_POINT ( 'NONE',  ( 5.935543223013869607, -0.8771126767605967878, 11.49999999999998224 ) ) ;
#14216=CYLINDRICAL_SURFACE ( 'NONE', #14654, 1.000000000000000888 ) ;
#14217=CARTESIAN_POINT ( 'NONE',  ( -4.286401442266546624, -4.198423832313179282, 30.86935038651143870 ) ) ;
#14220=CARTESIAN_POINT ( 'NONE',  ( 2.692335458626878175, 5.362264153667219979, 30.73760108194402818 ) ) ;
#14223=CARTESIAN_POINT ( 'NONE',  ( -2.668367453516631738, -5.373994336898133106, 4.867606119983652668 ) ) ;
#14225=CARTESIAN_POINT ( 'NONE',  ( 4.153440676704335921, 4.671190581744546044, 17.20045537531156654 ) ) ;
#14227=CARTESIAN_POINT ( 'NONE',  ( -0.9735954530123476225, 6.173909381474019575, 24.76281793585233615 ) ) ;
#14232=CARTESIAN_POINT ( 'NONE',  ( -5.317509234263865459, -2.779225709351170526, 17.99999999999998934 ) ) ;
#14233=CARTESIAN_POINT ( 'NONE',  ( 5.867109477881234270, 1.259218163100955135, 12.29888242247938202 ) ) ;
#14234=ORIENTED_EDGE ( 'NONE', *, *, #10365, .F. ) ;
#14242=CARTESIAN_POINT ( 'NONE',  ( -0.9740807849834127730, 5.920620690450721924, 24.23850119700668770 ) ) ;
#14246=EDGE_CURVE ( 'NONE', #7176, #7562, #15263, .T. ) ;
#14247=CARTESIAN_POINT ( 'NONE',  ( 5.317509234263995133, 2.779225709350928497, 18.13236078583908650 ) ) ;
#14250=CARTESIAN_POINT ( 'NONE',  ( 4.286401442266483564, 4.198423832313243231, 11.49999999999998224 ) ) ;
#14253=ORIENTED_EDGE ( 'NONE', *, *, #7457, .T. ) ;
#14254=CARTESIAN_POINT ( 'NONE',  ( -5.486741141153734347, 2.429871531109867533, 25.29888242247941221 ) ) ;
#14255=VERTEX_POINT ( 'NONE', #12274 ) ;
#14256=ORIENTED_EDGE ( 'NONE', *, *, #9015, .T. ) ;
#14257=CARTESIAN_POINT ( 'NONE',  ( -5.570820891630772209, -2.833901239560386642, 30.73763026556126476 ) ) ;
#14259=CARTESIAN_POINT ( 'NONE',  ( 1.000049271338486978, -6.169473353325553688, 4.869696127045518352 ) ) ;
#14261=CARTESIAN_POINT ( 'NONE',  ( -5.531623157106139388, 2.327208526676502132, 17.12635295315576300 ) ) ;
#14262=CARTESIAN_POINT ( 'NONE',  ( 2.668367453516445220, 5.373994336898223700, 24.63064961348855064 ) ) ;
#14263=CARTESIAN_POINT ( 'NONE',  ( 2.030576276931546336E-13, 6.000000000000000888, 25.49999999999999645 ) ) ;
#14264=CARTESIAN_POINT ( 'NONE',  ( -2.997451966578492222, 5.485105005465963579, 12.11517780375842790 ) ) ;
#14266=CARTESIAN_POINT ( 'NONE',  ( -3.255013540813738615, -5.336859797930776139, 25.37381964045071214 ) ) ;
#14270=CARTESIAN_POINT ( 'NONE',  ( -6.142908455506914223, -1.155755562476204590, 18.61517780375842790 ) ) ;
#14272=AXIS2_PLACEMENT_3D ( 'NONE', #11026, #12137, #124 ) ;
#14274=CARTESIAN_POINT ( 'NONE',  ( -3.736532060717997261, 4.696070028785964467, 4.026221760567070262 ) ) ;
#14275=CARTESIAN_POINT ( 'NONE',  ( 6.123233995736766282E-16, -6.250000000000000888, 5.000000000000004441 ) ) ;
#14277=FACE_OUTER_BOUND ( 'NONE', #6326, .T. ) ;
#14279=CARTESIAN_POINT ( 'NONE',  ( 5.131373506000491247, 7.062729720844170167, 17.99999999999998934 ) ) ;
#14280=VERTEX_POINT ( 'NONE', #9175 ) ;
#14285=CYLINDRICAL_SURFACE ( 'NONE', #9808, 1.000000000000000666 ) ;
#14288=B_SPLINE_CURVE_WITH_KNOTS ( 'NONE', 3,
 ( #3665, #2474, #86, #245, #5183, #8539, #9880, #8848, #1429, #8770, #7335, #9958, #12178, #13601, #6305, #2711, #6149, #10987 ),
 .UNSPECIFIED., .F., .F.,
 ( 4, 2, 2, 2, 2, 2, 2, 2, 4 ),
 ( 0.000000000000000000, 0.0003914898357794972241, 0.0007829796715589944483, 0.001174469507338491564, 0.001565959343117988897, 0.001957449178897486229, 0.002348939014676983128, 0.002740428850456480461, 0.003131918686235977793 ),
 .UNSPECIFIED. ) ;
#14290=CARTESIAN_POINT ( 'NONE',  ( 5.770331821586398569, 2.404225004693612000, 10.62619944752603196 ) ) ;
#14293=ORIENTED_EDGE ( 'NONE', *, *, #1458, .T. ) ;
#14294=LINE ( 'NONE', #2287, #5301 ) ;
#14295=CARTESIAN_POINT ( 'NONE',  ( 3.311576095066566694, 5.004818610361317255, 30.02622176056706493 ) ) ;
#14296=ORIENTED_EDGE ( 'NONE', *, *, #12522, .F. ) ;
#14297=CARTESIAN_POINT ( 'NONE',  ( -5.131373506000731055, 7.062729720844018289, 31.00000000000000000 ) ) ;
#14299=CARTESIAN_POINT ( 'NONE',  ( 3.458623254138613046, 5.207221900902883505, 17.02622717124729945 ) ) ;
#14301=CARTESIAN_POINT ( 'NONE',  ( 3.922396193919000407, -4.541970110199484267, 18.87380682714709579 ) ) ;
#14305=CARTESIAN_POINT ( 'NONE',  ( 7.799024015210652472, -1.482594289697024781, 11.49999999999998224 ) ) ;
#14308=CARTESIAN_POINT ( 'NONE',  ( 5.940390500375496430, 6.474944468551661281, 11.49999999999998224 ) ) ;
#14310=B_SPLINE_CURVE_WITH_KNOTS ( 'NONE', 3,
 ( #3516, #5035, #13302, #2563, #4962, #6315, #13224, #6237, #1204, #8549, #10920, #2399, #2485, #11151, #8625, #12185, #1283, #6157 ),
 .UNSPECIFIED., .F., .F.,
 ( 4, 2, 2, 2, 2, 2, 2, 2, 4 ),
 ( 0.003131918686235973456, 0.003523310662250264159, 0.003914702638264554863, 0.004306094614278845566, 0.004697486590293136269, 0.005088878566307427839, 0.005480270542321719410, 0.005871662518336010980, 0.006263054494350302551 ),
 .UNSPECIFIED. ) ;
#14314=CARTESIAN_POINT ( 'NONE',  ( 6.176542424588105540, 0.9554180641286316167, 5.000000000000004441 ) ) ;
#14318=CARTESIAN_POINT ( 'NONE',  ( 6.123233995736766282E-16, -6.000000000000000888, 6.000000000000005329 ) ) ;
#14319=CARTESIAN_POINT ( 'NONE',  ( 4.069684453406150482, 4.744965295353682500, 25.37380055247395561 ) ) ;
#14323=B_SPLINE_CURVE_WITH_KNOTS ( 'NONE', 3,
 ( #15434, #14223, #10424, #3250, #9545, #13195, #4534, #942, #3330, #705, #3488, #4695, #6772, #9465, #4452, #2055, #15356, #11689 ),
 .UNSPECIFIED., .F., .F.,
 ( 4, 2, 2, 2, 2, 2, 2, 2, 4 ),
 ( 0.000000000000000000, 0.0003914898357794969531, 0.0007829796715589939062, 0.001174469507338490913, 0.001565959343117987812, 0.001957449178897484494, 0.002348939014676980526, 0.002740428850456476557, 0.003131918686235972155 ),
 .UNSPECIFIED. ) ;
#14324=CARTESIAN_POINT ( 'NONE',  ( 5.903472034603497676, -2.056448723545186485, 3.999917806784441865 ) ) ;
#14325=EDGE_CURVE ( 'NONE', #3644, #3603, #6713, .T. ) ;
#14329=CARTESIAN_POINT ( 'NONE',  ( 6.172614129015222773, 0.9817721000789578767, 5.262369734438754776 ) ) ;
#14330=ORIENTED_EDGE ( 'NONE', *, *, #748, .F. ) ;
#14333=ORIENTED_EDGE ( 'NONE', *, *, #2290, .F. ) ;
#14335=VERTEX_POINT ( 'NONE', #9251 ) ;
#14337=CARTESIAN_POINT ( 'NONE',  ( 1.354942164753511828E-13, -6.250000000000000888, 16.99999999999998579 ) ) ;
#14339=CARTESIAN_POINT ( 'NONE',  ( -2.817313151351291012, -5.579000502529382288, 24.36762589283694780 ) ) ;
#14340=CARTESIAN_POINT ( 'NONE',  ( -4.142620314836442219, -4.341347824677446177, 25.11442521571937547 ) ) ;
#14342=CARTESIAN_POINT ( 'NONE',  ( -6.142844459177249306, 1.156093792145143961, 31.61560192892921251 ) ) ;
#14343=CARTESIAN_POINT ( 'NONE',  ( 3.736691294293271959, 4.695920479336495923, 25.47358595436692852 ) ) ;
#14344=CARTESIAN_POINT ( 'NONE',  ( -2.668367453516691690, -5.373994336898102020, 11.49999999999998224 ) ) ;
#14345=CARTESIAN_POINT ( 'NONE',  ( -4.435347140101121965, 4.403429997944423135, 11.63063932754213070 ) ) ;
#14346=CARTESIAN_POINT ( 'NONE',  ( -6.172552660730949547, -0.9821660343540521421, 24.23620383159192926 ) ) ;
#14351=CARTESIAN_POINT ( 'NONE',  ( -6.172639027853096927, -0.9816353142772993312, 18.26225281721714566 ) ) ;
#14355=CARTESIAN_POINT ( 'NONE',  ( -5.746996058422770837, 1.729015645941936796, 12.50007961174474858 ) ) ;
#14356=CARTESIAN_POINT ( 'NONE',  ( -0.7995298244853823455, -5.947211616899259923, 12.11456014619857946 ) ) ;
#14360=CARTESIAN_POINT ( 'NONE',  ( -6.176542424588100211, 0.9554180641286806885, 17.99999999999998934 ) ) ;
#14362=EDGE_CURVE ( 'NONE', #5008, #12192, #2966, .T. ) ;
#14364=CARTESIAN_POINT ( 'NONE',  ( -5.935543223013843850, -0.8771126767607685393, 31.00000000000000000 ) ) ;
#14373=DIRECTION ( 'NONE',  ( -1.000000000000000000, 0.000000000000000000, 0.000000000000000000 ) ) ;
#14375=CARTESIAN_POINT ( 'NONE',  ( 6.176542424588126856, 0.9554180641284961695, 17.86936067245787285 ) ) ;
#14380=CARTESIAN_POINT ( 'NONE',  ( 5.866817325727539334, 1.260653813891824182, 23.69977782616121331 ) ) ;
#14384=CARTESIAN_POINT ( 'NONE',  ( 5.486982057989181705, -2.429327048029897629, 5.799318062581740207 ) ) ;
#14385=CARTESIAN_POINT ( 'NONE',  ( -4.267992336621205141, 4.217442018459991893, 31.26194324003147429 ) ) ;
#14386=AXIS2_PLACEMENT_3D ( 'NONE', #4048, #9875, #8919 ) ;
#14390=CARTESIAN_POINT ( 'NONE',  ( 3.632753594129205510, 4.777047695051075848, 18.99995053646221521 ) ) ;
#14392=CARTESIAN_POINT ( 'NONE',  ( 4.267936573529251376, -4.217499624512195844, 11.23770962164068798 ) ) ;
#14394=CARTESIAN_POINT ( 'NONE',  ( 0.2622538972264353285, -6.245673238944475791, 31.97385994369199835 ) ) ;
#14395=CARTESIAN_POINT ( 'NONE',  ( -6.172639027853123572, 0.9816353142771289120, 11.23774718278287743 ) ) ;
#14396=CARTESIAN_POINT ( 'NONE',  ( -1.000079958708000483, -5.916066267613719454, 18.13152738882033432 ) ) ;
#14397=ORIENTED_EDGE ( 'NONE', *, *, #1458, .F. ) ;
#14400=CARTESIAN_POINT ( 'NONE',  ( -3.311384659207207370, 5.004923837169374501, 12.47358595436692852 ) ) ;
#14402=ADVANCED_FACE ( 'NONE', ( #5671 ), #11625, .F. ) ;
#14405=B_SPLINE_CURVE_WITH_KNOTS ( 'NONE', 3,
 ( #4028, #8904, #8743, #2847, #449, #5396, #5158, #8984, #221, #5080, #14859, #13888, #4192, #7855, #7695, #1641, #6517, #11117 ),
 .UNSPECIFIED., .F., .F.,
 ( 4, 2, 2, 2, 2, 2, 2, 2, 4 ),
 ( 0.000000000000000000, 0.0003914357524127460761, 0.0007828715048254921522, 0.001174307257238238174, 0.001565743009650984304, 0.001957178762063730218, 0.002348614514476476348, 0.002740050266889222479, 0.003131486019301968609 ),
 .UNSPECIFIED. ) ;
#14406=DIRECTION ( 'NONE',  ( 0.000000000000000000, 1.000000000000000000, 0.000000000000000000 ) ) ;
#14408=CARTESIAN_POINT ( 'NONE',  ( 5.726049995854435970, 2.506679546901950051, 31.79954462468841214 ) ) ;
#14412=CARTESIAN_POINT ( 'NONE',  ( 5.571002711501416016, -2.833546409886269934, 4.736203831591940805 ) ) ;
#14419=CYLINDRICAL_SURFACE ( 'NONE', #11379, 1.000000000000000888 ) ;
#14421=ORIENTED_EDGE ( 'NONE', *, *, #13611, .T. ) ;
#14423=CARTESIAN_POINT ( 'NONE',  ( -6.142844459177229766, -1.156093792145233001, 30.38439807107076973 ) ) ;
#14427=CARTESIAN_POINT ( 'NONE',  ( -3.011385983131470212, -5.190390249166353165, 25.29952054102714953 ) ) ;
#14428=CARTESIAN_POINT ( 'NONE',  ( 4.267558728637206755, -4.217879122113790125, 11.76382603205595423 ) ) ;
#14430=CARTESIAN_POINT ( 'NONE',  ( 2.848235266350816808, 5.281699484015757839, 25.11397738943081848 ) ) ;
#14432=CARTESIAN_POINT ( 'NONE',  ( -3.882673863916337176, 4.899192824800900681, 12.47408542334169113 ) ) ;
#14433=CARTESIAN_POINT ( 'NONE',  ( -5.648794263291666340, -2.676232015153777510, 23.88558052754514094 ) ) ;
#14439=CARTESIAN_POINT ( 'NONE',  ( 2.668367453516610865, 5.373994336898140212, 31.00000000000000000 ) ) ;
#14440=CARTESIAN_POINT ( 'NONE',  ( 5.935543223013849179, 0.8771126767607271280, 31.00000000000000000 ) ) ;
#14443=CARTESIAN_POINT ( 'NONE',  ( 0.8002302970947245964, -5.947135855825854023, 10.88601773212297985 ) ) ;
#14446=EDGE_LOOP ( 'NONE', ( #9229, #4710, #15625, #3342 ) ) ;
#14449=CYLINDRICAL_SURFACE ( 'NONE', #9707, 1.000000000000000666 ) ;
#14450=LINE ( 'NONE', #4994, #4368 ) ;
#14453=EDGE_CURVE ( 'NONE', #2012, #5925, #11091, .T. ) ;
#14454=DIRECTION ( 'NONE',  ( 0.9510565162951499785, 0.3090169943749582204, 0.000000000000000000 ) ) ;
#14456=CARTESIAN_POINT ( 'NONE',  ( -4.291255145204061705, 4.544933371694689583, 5.613961794080712053 ) ) ;
#14465=ORIENTED_EDGE ( 'NONE', *, *, #5042, .F. ) ;
#14468=FACE_OUTER_BOUND ( 'NONE', #1504, .T. ) ;
#14470=B_SPLINE_CURVE_WITH_KNOTS ( 'NONE', 3,
 ( #10288, #5597, #1765, #13934, #10521, #6871, #11547, #14015, #3045, #10211, #1920, #12668, #5673, #574, #9105, #4236, #13855, #7898 ),
 .UNSPECIFIED., .F., .F.,
 ( 4, 2, 2, 2, 2, 2, 2, 2, 4 ),
 ( 0.000000000000000000, 0.0003914898357794965736, 0.0007829796715589931472, 0.001174469507338489829, 0.001565959343117986294, 0.001957449178897482760, 0.002348939014676979659, 0.002740428850456476124, 0.003131918686235972589 ),
 .UNSPECIFIED. ) ;
#14471=EDGE_CURVE ( 'NONE', #2830, #12811, #15634, .T. ) ;
#14472=COLOUR_RGB ( '', 0.09019608, 0.27058824, 0.51372549) ;
#14473=CARTESIAN_POINT ( 'NONE',  ( 0.5039005892423336075, -6.230833003620525723, 23.62636388911297303 ) ) ;
#14475=CARTESIAN_POINT ( 'NONE',  ( 0.9999171162590435591, 6.169494774098537526, 11.36722320330675906 ) ) ;
#14477=CARTESIAN_POINT ( 'NONE',  ( 3.419318284370187477, -4.932111238568182898, 18.99992002356260201 ) ) ;
#14479=CARTESIAN_POINT ( 'NONE',  ( -0.7988914244718040569, -5.947301735519289423, 30.38456289168619051 ) ) ;
#14481=CARTESIAN_POINT ( 'NONE',  ( 0.7993401192312087344, -6.199366368793657323, 31.61483246936573721 ) ) ;
#14482=CARTESIAN_POINT ( 'NONE',  ( -6.176542424588111757, 0.9554180641286128539, 11.36762589283694425 ) ) ;
#14483=CARTESIAN_POINT ( 'NONE',  ( -5.783239563508432823, 1.602707436861086299, 30.02641404563305016 ) ) ;
#14484=ORIENTED_EDGE ( 'NONE', *, *, #8988, .F. ) ;
#14487=ORIENTED_EDGE ( 'NONE', *, *, #12425, .T. ) ;
#14488=CARTESIAN_POINT ( 'NONE',  ( -3.107688324358770071, 5.133887830459799240, 12.37378430870260715 ) ) ;
#14489=VERTEX_POINT ( 'NONE', #12020 ) ;
#14490=ADVANCED_FACE ( 'NONE', ( #8214 ), #2391, .F. ) ;
#14493=CARTESIAN_POINT ( 'NONE',  ( 6.021135683317684339, 1.680226122398269295, 31.97377282875269700 ) ) ;
#14496=CARTESIAN_POINT ( 'NONE',  ( -2.668367453516692134, -5.373994336898103796, 11.36760611998364467 ) ) ;
#14499=ADVANCED_FACE ( 'NONE', ( #5985 ), #1195, .F. ) ;
#14500=CARTESIAN_POINT ( 'NONE',  ( 2.817313151351187983, -5.579000502529432914, 4.869360672457872852 ) ) ;
#14504=ORIENTED_EDGE ( 'NONE', *, *, #993, .F. ) ;
#14506=ORIENTED_EDGE ( 'NONE', *, *, #11965, .F. ) ;
#14508=CARTESIAN_POINT ( 'NONE',  ( 0.1323408341374887331, 6.250000000000000888, 32.00000000000000000 ) ) ;
#14512=DIRECTION ( 'NONE',  ( 0.5877852522924802425, -0.8090169943749422332, 0.000000000000000000 ) ) ;
#14513=CARTESIAN_POINT ( 'NONE',  ( -4.286401442266578599, -4.198423832313146420, 11.49999999999998224 ) ) ;
#14515=CARTESIAN_POINT ( 'NONE',  ( 5.935543223013849179, 0.8771126767607271280, 31.00000000000000000 ) ) ;
#14516=DIRECTION ( 'NONE',  ( -0.3090169943749584980, 0.9510565162951498674, 0.000000000000000000 ) ) ;
#14521=CARTESIAN_POINT ( 'NONE',  ( 5.770288754215171956, -2.404361317819854182, 17.12618035954928075 ) ) ;
#14522=CARTESIAN_POINT ( 'NONE',  ( 5.747343991580175171, 1.727858744772314159, 31.99992002356261267 ) ) ;
#14524=CARTESIAN_POINT ( 'NONE',  ( -3.634089073485431420, 4.776071126502690944, 4.000079976437387330 ) ) ;
#14525=CARTESIAN_POINT ( 'NONE',  ( -0.8738118504724939895, -5.936246475285042123, 12.00357242174242423 ) ) ;
#14526=CARTESIAN_POINT ( 'NONE',  ( 5.931793676715113151, 0.9035324301687462922, 24.76239891805597537 ) ) ;
#14533=CARTESIAN_POINT ( 'NONE',  ( 5.317509234263970264, -2.779225709350972906, 4.867639214160894845 ) ) ;
#14535=CARTESIAN_POINT ( 'NONE',  ( -6.081509788407740480, 1.446521464462707129, 12.37381964045070504 ) ) ;
#14538=CYLINDRICAL_SURFACE ( 'NONE', #6287, 1.000000000000000888 ) ;
#14539=CARTESIAN_POINT ( 'NONE',  ( -5.940390500375673177, 6.474944468551537824, 31.00000000000000000 ) ) ;
#14542=CARTESIAN_POINT ( 'NONE',  ( 5.616089948629745976, 2.743103014345511070, 17.49563030319846746 ) ) ;
#14546=CARTESIAN_POINT ( 'NONE',  ( -4.416678568553683348, -4.422441866694277302, 11.76236973443872280 ) ) ;
#14548=ADVANCED_FACE ( 'NONE', ( #8133 ), #962, .F. ) ;
#14550=CARTESIAN_POINT ( 'NONE',  ( 5.746619684944276329, -1.730157667110832298, 6.000049320733125136 ) ) ;
#14553=CARTESIAN_POINT ( 'NONE',  ( 7.347881158177969135E-16, 6.250000000000000888, 4.000000000000004441 ) ) ;
#14555=LINE ( 'NONE', #9792, #3357 ) ;
#14558=CARTESIAN_POINT ( 'NONE',  ( 5.931793676715104269, -0.9035324301687984727, 11.23760108194400864 ) ) ;
#14561=CARTESIAN_POINT ( 'NONE',  ( -5.531623157106185573, 2.327208526676387557, 30.12635295315577366 ) ) ;
#14564=VECTOR ( 'NONE', #1422, 1000.000000000000000 ) ;
#14565=ORIENTED_EDGE ( 'NONE', *, *, #2448, .F. ) ;
#14566=EDGE_CURVE ( 'NONE', #5961, #8844, #2755, .T. ) ;
#14568=CARTESIAN_POINT ( 'NONE',  ( -5.317509234263835260, -2.779225709351231366, 24.49999999999999289 ) ) ;
#14571=CARTESIAN_POINT ( 'NONE',  ( 0.7988914244718127167, 5.947301735519285870, 4.384562891686175412 ) ) ;
#14577=CARTESIAN_POINT ( 'NONE',  ( 3.106366801612054029, -5.134708448381249291, 31.87303779027051576 ) ) ;
#14582=B_SPLINE_CURVE_WITH_KNOTS ( 'NONE', 3,
 ( #11744, #13976, #5865, #2188, #9141, #13091, #11667, #9365, #1877, #14049, #5634, #7059, #13013, #12853, #11894, #7930, #6752, #11586 ),
 .UNSPECIFIED., .F., .F.,
 ( 4, 2, 2, 2, 2, 2, 2, 2, 4 ),
 ( 0.003131923598877004410, 0.003523316383094321751, 0.003914709167311639093, 0.004306101951528956001, 0.004697494735746272909, 0.005088887519963589817, 0.005480280304180906725, 0.005871673088398223633, 0.006263065872615540541 ),
 .UNSPECIFIED. ) ;
#14584=ORIENTED_EDGE ( 'NONE', *, *, #10283, .T. ) ;
#14586=ORIENTED_EDGE ( 'NONE', *, *, #11076, .T. ) ;
#14587=EDGE_LOOP ( 'NONE', ( #4395, #2627 ) ) ;
#14588=CARTESIAN_POINT ( 'NONE',  ( -5.725684683139601105, -2.507514573674792135, 30.20112161576661691 ) ) ;
#14589=CARTESIAN_POINT ( 'NONE',  ( 3.312524433819772351, -5.004191858254007030, 17.02591947216898660 ) ) ;
#14592=B_SPLINE_CURVE_WITH_KNOTS ( 'NONE', 3,
 ( #9016, #484, #15127, #4304, #13477, #11458, #4223, #6255, #404, #7886, #1673, #1380, #5353, #10199, #12654, #13921, #12727, #871 ),
 .UNSPECIFIED., .F., .F.,
 ( 4, 2, 2, 2, 2, 2, 2, 2, 4 ),
 ( 0.000000000000000000, 0.0003914357524127483529, 0.0007828715048254967059, 0.001174307257238245113, 0.001565743009650993412, 0.001957178762063741927, 0.002348614514476490226, 0.002740050266889238525, 0.003131486019301986824 ),
 .UNSPECIFIED. ) ;
#14593=CARTESIAN_POINT ( 'NONE',  ( -5.725684683139636633, 2.507514573674706426, 31.79887838423339019 ) ) ;
#14594=AXIS2_PLACEMENT_3D ( 'NONE', #15091, #2760, #7768 ) ;
#14599=CARTESIAN_POINT ( 'NONE',  ( -4.154121946520968223, 4.670585111242886001, 10.70112161576659915 ) ) ;
#14601=CARTESIAN_POINT ( 'NONE',  ( -6.155854678529437685, -1.081900940642313236, 23.99574050496988065 ) ) ;
#14607=VECTOR ( 'NONE', #11194, 1000.000000000000000 ) ;
#14610=CARTESIAN_POINT ( 'NONE',  ( -2.668367453516708565, 5.373994336898094026, 5.000000000000004441 ) ) ;
#14612=CARTESIAN_POINT ( 'NONE',  ( 5.375913338529152874, 2.664979843780314273, 25.00428920362019980 ) ) ;
#14613=CARTESIAN_POINT ( 'NONE',  ( 3.458623254138780911, -5.207221900902773370, 31.97377282875268989 ) ) ;
#14614=CYLINDRICAL_SURFACE ( 'NONE', #12480, 1.000000000000000666 ) ;
#14615=EDGE_CURVE ( 'NONE', #902, #2089, #4643, .T. ) ;
#14616=CARTESIAN_POINT ( 'NONE',  ( -2.692693252389644520, 5.362085866495079678, 11.23617396794405465 ) ) ;
#14617=B_SPLINE_CURVE_WITH_KNOTS ( 'NONE', 3,
 ( #4765, #10962, #9703, #14542, #13345, #9538, #15664, #1328, #12228, #3639, #8514, #7461, #5960, #10727, #8668, #6202, #14375, #7312 ),
 .UNSPECIFIED., .F., .F.,
 ( 4, 2, 2, 2, 2, 2, 2, 2, 4 ),
 ( 0.000000000000000000, 0.0003914357524127464556, 0.0007828715048254929112, 0.001174307257238239258, 0.001565743009650985822, 0.001957178762063732386, 0.002348614514476478517, 0.002740050266889225081, 0.003131486019301971645 ),
 .UNSPECIFIED. ) ;
#14624=FACE_BOUND ( 'NONE', #5025, .T. ) ;
#14627=CARTESIAN_POINT ( 'NONE',  ( 5.649053410273161546, -2.675685104943071213, 25.11517780375841724 ) ) ;
#14628=EDGE_LOOP ( 'NONE', ( #3503, #6753 ) ) ;
#14635=B_SPLINE_CURVE_WITH_KNOTS ( 'NONE', 3,
 ( #10892, #8598, #5885, #2537, #12232, #1333, #4030, #6206, #1021, #11043, #15590, #9542, #14380, #8356, #2289, #5965, #10809, #4770 ),
 .UNSPECIFIED., .F., .F.,
 ( 4, 2, 2, 2, 2, 2, 2, 2, 4 ),
 ( 0.000000000000000000, 0.0003914898357794970073, 0.0007829796715589940146, 0.001174469507338491130, 0.001565959343117988029, 0.001957449178897484928, 0.002348939014676982261, 0.002740428850456479160, 0.003131918686235976058 ),
 .UNSPECIFIED. ) ;
#14638=CARTESIAN_POINT ( 'NONE',  ( 2.030576276931546336E-13, -6.250000000000000888, 25.49999999999999645 ) ) ;
#14640=CARTESIAN_POINT ( 'NONE',  ( -0.9999171162589062245, -6.169494774098559731, 11.36722320330676084 ) ) ;
#14646=CARTESIAN_POINT ( 'NONE',  ( -0.2637975869346481095, -6.245592211692898132, 18.97332839949189776 ) ) ;
#14648=CARTESIAN_POINT ( 'NONE',  ( 3.010624175977807848, 5.190832888732320072, 23.70111757752058423 ) ) ;
#14649=EDGE_CURVE ( 'NONE', #5163, #9339, #14288, .T. ) ;
#14650=VERTEX_POINT ( 'NONE', #4954 ) ;
#14654=AXIS2_PLACEMENT_3D ( 'NONE', #8188, #13025, #5413 ) ;
#14662=ADVANCED_FACE ( 'NONE', ( #11528 ), #5499, .F. ) ;
#14663=CARTESIAN_POINT ( 'NONE',  ( 2.782156709077468815, -5.316215864844020977, 31.50312048902376816 ) ) ;
#14665=CARTESIAN_POINT ( 'NONE',  ( 4.153663429050834743, -4.670992970568328850, 4.200668510924230326 ) ) ;
#14669=ORIENTED_EDGE ( 'NONE', *, *, #178, .T. ) ;
#14670=ORIENTED_EDGE ( 'NONE', *, *, #9992, .F. ) ;
#14671=ORIENTED_EDGE ( 'NONE', *, *, #12116, .F. ) ;
#14672=CARTESIAN_POINT ( 'NONE',  ( -5.648794263291724960, -2.676232015153657606, 10.88558052754513383 ) ) ;
#14674=CARTESIAN_POINT ( 'NONE',  ( -0.8730424326980914529, -5.936362132114464174, 4.495006902185641806 ) ) ;
#14675=CARTESIAN_POINT ( 'NONE',  ( -5.859221468178962056, -2.178708437343193971, 31.97408542334170889 ) ) ;
#14679=DIRECTION ( 'NONE',  ( 0.000000000000000000, 0.000000000000000000, 1.000000000000000000 ) ) ;
#14681=CYLINDRICAL_SURFACE ( 'NONE', #2094, 1.000000000000000666 ) ;
#14688=CARTESIAN_POINT ( 'NONE',  ( -3.922672396097064418, 4.541739265057694652, 5.873647046844240549 ) ) ;
#14693=VECTOR ( 'NONE', #13349, 1000.000000000000000 ) ;
#14694=DIRECTION ( 'NONE',  ( 0.000000000000000000, 1.000000000000000000, 0.000000000000000000 ) ) ;
#14695=ADVANCED_FACE ( 'NONE', ( #6619 ), #3386, .F. ) ;
#14697=DIRECTION ( 'NONE',  ( -0.9510565162951545304, 0.3090169943749447867, 0.000000000000000000 ) ) ;
#14701=CARTESIAN_POINT ( 'NONE',  ( -4.286401442266578599, -4.198423832313146420, 11.49999999999998224 ) ) ;
#14704=ADVANCED_FACE ( 'NONE', ( #15120 ), #626, .F. ) ;
#14705=CARTESIAN_POINT ( 'NONE',  ( 0.2638277032949121748, 5.995407492418038053, 31.97332055281518137 ) ) ;
#14706=B_SPLINE_CURVE_WITH_KNOTS ( 'NONE', 3,
 ( #7120, #9750, #14257, #5926, #11871, #14588, #13386, #5845, #1062, #10847, #8561, #11956, #8235, #14423, #3529, #15710, #8399, #10772 ),
 .UNSPECIFIED., .F., .F.,
 ( 4, 2, 2, 2, 2, 2, 2, 2, 4 ),
 ( 0.003131486019301978150, 0.003522824630466686157, 0.003914163241631393730, 0.004305501852796101737, 0.004696840463960809745, 0.005088179075125517752, 0.005479517686290225759, 0.005870856297454933766, 0.006262194908619641773 ),
 .UNSPECIFIED. ) ;
#14709=AXIS2_PLACEMENT_3D ( 'NONE', #1310, #8500, #2517 ) ;
#14711=CYLINDRICAL_SURFACE ( 'NONE', #7830, 1.000000000000000666 ) ;
#14713=CARTESIAN_POINT ( 'NONE',  ( 4.344265632482096073, 4.493596842504949507, 30.49574050496988420 ) ) ;
#14715=CARTESIAN_POINT ( 'NONE',  ( -4.286401442266677186, -4.198423832313046944, 24.36935038651144225 ) ) ;
#14716=CARTESIAN_POINT ( 'NONE',  ( 0.1323736289506388109, -6.249999999999996447, 25.49999999999999645 ) ) ;
#14717=CARTESIAN_POINT ( 'NONE',  ( 2.817313151350923750, 5.579000502529566141, 24.63063932754212004 ) ) ;
#14725=AXIS2_PLACEMENT_3D ( 'NONE', #2566, #12345, #5278 ) ;
#14727=CARTESIAN_POINT ( 'NONE',  ( -2.817313151351207523, 5.579000502529421368, 30.86765874365831763 ) ) ;
#14728=DIRECTION ( 'NONE',  ( 0.5877852522924802425, -0.8090169943749422332, 0.000000000000000000 ) ) ;
#14729=CARTESIAN_POINT ( 'NONE',  ( 3.311576095066412151, 5.004818610361416731, 23.52622176056705783 ) ) ;
#14731=EDGE_LOOP ( 'NONE', ( #1723, #3545 ) ) ;
#14733=VERTEX_POINT ( 'NONE', #12721 ) ;
#14735=EDGE_LOOP ( 'NONE', ( #1403, #8254, #2871, #7334 ) ) ;
#14737=CARTESIAN_POINT ( 'NONE',  ( 5.571002711501436444, 2.833546409886228190, 18.26379616840806008 ) ) ;
#14738=CARTESIAN_POINT ( 'NONE',  ( 0.000000000000000000, 0.000000000000000000, 0.000000000000000000 ) ) ;
#14739=CARTESIAN_POINT ( 'NONE',  ( -0.1323736289504250097, 6.250000000000000000, 25.49999999999997158 ) ) ;
#14741=DIRECTION ( 'NONE',  ( 0.000000000000000000, 0.000000000000000000, 1.000000000000000000 ) ) ;
#14744=LINE ( 'NONE', #2564, #13835 ) ;
#14746=CARTESIAN_POINT ( 'NONE',  ( -5.859221468178992254, 2.178708437343110482, 30.02591457665829466 ) ) ;
#14748=B_SPLINE_CURVE_WITH_KNOTS ( 'NONE', 3,
 ( #11509, #7779, #455, #2691, #2930, #5248, #5403, #7625, #4119, #4037, #8911, #5327, #12390, #2773, #4199, #10251, #11357, #6367 ),
 .UNSPECIFIED., .F., .F.,
 ( 4, 2, 2, 2, 2, 2, 2, 2, 4 ),
 ( 0.000000000000000000, 0.0003914357524127471603, 0.0007828715048254943206, 0.001174307257238241427, 0.001565743009650988641, 0.001957178762063735856, 0.002348614514476482854, 0.002740050266889230285, 0.003131486019301977283 ),
 .UNSPECIFIED. ) ;
#14749=ORIENTED_EDGE ( 'NONE', *, *, #6913, .F. ) ;
#14752=CARTESIAN_POINT ( 'NONE',  ( 1.000079958708271821, 5.916066267613677709, 18.13152738882034143 ) ) ;
#14755=CARTESIAN_POINT ( 'NONE',  ( -5.648794263291692097, -2.676232015153728216, 17.38558052754515160 ) ) ;
#14756=ADVANCED_FACE ( 'NONE', ( #14277 ), #2190, .F. ) ;
#14757=CARTESIAN_POINT ( 'NONE',  ( 0.6151877315911188360, -6.220340188096003864, 18.79906673469668732 ) ) ;
#14758=CARTESIAN_POINT ( 'NONE',  ( 0.6156307853270029939, 5.969051238897248979, 12.29870573410680556 ) ) ;
#14761=CARTESIAN_POINT ( 'NONE',  ( 5.620786884546321360, -2.102685372472797631, 12.47358595436692319 ) ) ;
#14762=CARTESIAN_POINT ( 'NONE',  ( -2.841041022017514184, 5.567186575787197889, 18.26225281721714566 ) ) ;
#14768=ORIENTED_EDGE ( 'NONE', *, *, #358, .F. ) ;
#14769=CARTESIAN_POINT ( 'NONE',  ( -4.196038884587180995, 4.289036423669260856, 5.503897950159858610 ) ) ;
#14771=CARTESIAN_POINT ( 'NONE',  ( 3.568242062701560524, -5.132954954975482487, 10.49995093123465217 ) ) ;
#14772=CARTESIAN_POINT ( 'NONE',  ( 0.1306394121200051550, -6.250000000000003553, 10.49999999999998579 ) ) ;
#14775=CARTESIAN_POINT ( 'NONE',  ( -2.849573632035303561, 5.280958870664584914, 10.88438267301394369 ) ) ;
#14777=CARTESIAN_POINT ( 'NONE',  ( 5.843318061569054755, -1.367618216965598821, 4.126962209729495790 ) ) ;
#14778=CARTESIAN_POINT ( 'NONE',  ( -0.7988860301921972829, -6.199427171881341181, 30.38455580536194134 ) ) ;
#14783=CARTESIAN_POINT ( 'NONE',  ( 3.779681992289742887, 4.979315417303941338, 12.49995078984291830 ) ) ;
#14791=CARTESIAN_POINT ( 'NONE',  ( 6.143143148203064285, -1.154591847827665774, 12.11396179408069607 ) ) ;
#14792=ADVANCED_FACE ( 'NONE', ( #5422 ), #475, .F. ) ;
#14793=CARTESIAN_POINT ( 'NONE',  ( 4.416779112813619790, -4.422345839825831071, 17.73774718278285079 ) ) ;
#14796=CARTESIAN_POINT ( 'NONE',  ( 2.668367453516506060, 5.373994336898192614, 17.86938304467859950 ) ) ;
#14801=CARTESIAN_POINT ( 'NONE',  ( -0.5042675786777902625, -6.230788509548851550, 18.87331068310446369 ) ) ;
#14802=CARTESIAN_POINT ( 'NONE',  ( -5.935543223013839409, -0.8771126767608161678, 11.63239388001634289 ) ) ;
#14803=CARTESIAN_POINT ( 'NONE',  ( -4.286401442266737583, 4.198423832312984771, 24.49999999999999289 ) ) ;
#14807=CARTESIAN_POINT ( 'NONE',  ( 7.180990026460783326, -3.384707322287269893, 17.99999999999998934 ) ) ;
#14813=CARTESIAN_POINT ( 'NONE',  ( 5.649200442566199243, 2.675373855294061798, 18.61560192892921251 ) ) ;
#14815=DIRECTION ( 'NONE',  ( 0.8090169943749506709, -0.5877852522924689183, 0.000000000000000000 ) ) ;
#14819=CARTESIAN_POINT ( 'NONE',  ( 4.286401442266533302, 4.198423832313197046, 5.132393880016353549 ) ) ;
#14822=CARTESIAN_POINT ( 'NONE',  ( 6.176542424588132185, -0.9554180641284774067, 11.36939309276498911 ) ) ;
#14825=ORIENTED_EDGE ( 'NONE', *, *, #11157, .T. ) ;
#14827=FACE_OUTER_BOUND ( 'NONE', #7732, .T. ) ;
#14829=VERTEX_POINT ( 'NONE', #9087 ) ;
#14830=CARTESIAN_POINT ( 'NONE',  ( -0.9999196734182633772, -5.916093360767516351, 4.867259559550685566 ) ) ;
#14831=CARTESIAN_POINT ( 'NONE',  ( -2.692693252389637859, -5.362085866495083231, 18.26382603205596311 ) ) ;
#14835=CARTESIAN_POINT ( 'NONE',  ( -2.817313151351249711, 5.579000502529400940, 11.49999999999998224 ) ) ;
#14836=CARTESIAN_POINT ( 'NONE',  ( 0.2619456584324066362, -5.995505046955607042, 23.52607193928647433 ) ) ;
#14841=AXIS2_PLACEMENT_3D ( 'NONE', #6611, #15113, #15035 ) ;
#14842=EDGE_CURVE ( 'NONE', #6001, #15154, #4136, .T. ) ;
#14847=CARTESIAN_POINT ( 'NONE',  ( -3.736532060718149140, 4.696070028785846340, 23.52622176056705783 ) ) ;
#14848=CARTESIAN_POINT ( 'NONE',  ( 1.000079958708342653, 5.916066267613666163, 24.63152738882033432 ) ) ;
#14850=CARTESIAN_POINT ( 'NONE',  ( 3.011899281037336173, -5.190111395030321262, 23.69977782616121331 ) ) ;
#14852=CARTESIAN_POINT ( 'NONE',  ( -4.416678568553842332, 4.422441866694120094, 24.23763026556123634 ) ) ;
#14853=CARTESIAN_POINT ( 'NONE',  ( 5.931793676715082952, 0.9035324301689496851, 5.262398918055979813 ) ) ;
#14855=FACE_BOUND ( 'NONE', #4708, .T. ) ;
#14856=EDGE_CURVE ( 'NONE', #3740, #5609, #4217, .T. ) ;
#14859=CARTESIAN_POINT ( 'NONE',  ( -3.882673863916255463, -4.899192824800964630, 10.52591457665827512 ) ) ;
#14862=CARTESIAN_POINT ( 'NONE',  ( -4.005361199355110813, 4.468319061418669413, 18.80022217383877958 ) ) ;
#14867=CARTESIAN_POINT ( 'NONE',  ( 5.770331821586440313, -2.404225004693508527, 12.37380055247394672 ) ) ;
#14869=CYLINDRICAL_SURFACE ( 'NONE', #13953, 1.000000000000000222 ) ;
#14870=CARTESIAN_POINT ( 'NONE',  ( 5.915699123067200027, -1.003533581835301280, 25.00389795015983552 ) ) ;
#14873=CARTESIAN_POINT ( 'NONE',  ( 5.531757352715619191, -2.326874507723291963, 10.62619317285287934 ) ) ;
#14874=CARTESIAN_POINT ( 'NONE',  ( -0.1306070469492023600, -6.250000000000004441, 16.99999999999999289 ) ) ;
#14876=CARTESIAN_POINT ( 'NONE',  ( -7.799024015210663130, -1.482594289697217294, 5.000000000000004441 ) ) ;
#14881=ADVANCED_FACE ( 'NONE', ( #3025 ), #1821, .F. ) ;
#14883=CARTESIAN_POINT ( 'NONE',  ( -5.665308849928751833, -1.980336949702712790, 23.50007997643738022 ) ) ;
#14884=VERTEX_POINT ( 'NONE', #10423 ) ;
#14885=CARTESIAN_POINT ( 'NONE',  ( 0.000000000000000000, 0.000000000000000000, 0.000000000000000000 ) ) ;
#14890=CARTESIAN_POINT ( 'NONE',  ( 0.2638277032948923018, 5.995407492418038053, 5.973320552815183149 ) ) ;
#14892=LINE ( 'NONE', #328, #1327 ) ;
#14894=FACE_OUTER_BOUND ( 'NONE', #6228, .T. ) ;
#14895=CARTESIAN_POINT ( 'NONE',  ( 3.633127580202317741, -4.776802569231024975, 32.00007961174476634 ) ) ;
#14897=CARTESIAN_POINT ( 'NONE',  ( 5.770288754215145310, -2.404361317819922572, 10.62618035954928253 ) ) ;
#14898=CARTESIAN_POINT ( 'NONE',  ( 3.011899281037413889, 5.190111395030279517, 12.30022217383879024 ) ) ;
#14900=EDGE_LOOP ( 'NONE', ( #1354, #15135 ) ) ;
#14902=ORIENTED_EDGE ( 'NONE', *, *, #14994, .F. ) ;
#14904=CARTESIAN_POINT ( 'NONE',  ( 4.435347140101010055, 4.403429997944536822, 5.000000000000004441 ) ) ;
#14906=CARTESIAN_POINT ( 'NONE',  ( -5.558508435838124484, -2.857531096719054808, 17.86939309276500154 ) ) ;
#14907=CARTESIAN_POINT ( 'NONE',  ( 0.5043776560898699524, -6.230795654995827881, 18.87337476296010053 ) ) ;
#14908=CARTESIAN_POINT ( 'NONE',  ( -0.2622538972263916968, 6.245673238944478456, 18.97385994369195572 ) ) ;
#14911=CARTESIAN_POINT ( 'NONE',  ( -2.817313151351372724, 5.579000502529338767, 24.49999999999999289 ) ) ;
#14912=CARTESIAN_POINT ( 'NONE',  ( -4.070863287254184115, 4.743975846881713920, 10.62694108445697161 ) ) ;
#14913=VECTOR ( 'NONE', #11137, 1000.000000000000000 ) ;
#14914=CARTESIAN_POINT ( 'NONE',  ( 2.668367453516506504, 5.373994336898192614, 17.99999999999998934 ) ) ;
#14920=ORIENTED_EDGE ( 'NONE', *, *, #9262, .T. ) ;
#14921=CARTESIAN_POINT ( 'NONE',  ( -5.866923913994642525, 1.260079467906539241, 12.29952054102714243 ) ) ;
#14924=CARTESIAN_POINT ( 'NONE',  ( -1.000049271338485646, 6.169473353325552800, 4.869696127045516576 ) ) ;
#14927=CARTESIAN_POINT ( 'NONE',  ( 3.459597053047843040, 5.206576120509745387, 5.974085423341712442 ) ) ;
#14929=CARTESIAN_POINT ( 'NONE',  ( 2.692335458626892386, 5.362264153667214650, 4.737601081944043280 ) ) ;
#14931=DIRECTION ( 'NONE',  ( -0.9510565162951544194, 0.3090169943749447312, 0.000000000000000000 ) ) ;
#14933=FACE_BOUND ( 'NONE', #11644, .T. ) ;
#14940=CARTESIAN_POINT ( 'NONE',  ( 5.649053410273137565, -2.675685104943120507, 18.61517780375842790 ) ) ;
#14944=CARTESIAN_POINT ( 'NONE',  ( -6.000000000000000888, 0.000000000000000000, 53.67766952966368876 ) ) ;
#14947=CARTESIAN_POINT ( 'NONE',  ( -5.131373506000878493, 7.062729720843910819, 24.49999999999999289 ) ) ;
#14954=B_SPLINE_CURVE_WITH_KNOTS ( 'NONE', 3,
 ( #9655, #14496, #1674, #7805, #405, #7573, #10275, #7649, #6627, #13922, #14976, #12498, #331, #1596, #634, #12728, #8937, #485 ),
 .UNSPECIFIED., .F., .F.,
 ( 4, 2, 2, 2, 2, 2, 2, 2, 4 ),
 ( 0.000000000000000000, 0.0003914898357794939715, 0.0007829796715589879431, 0.001174469507338482023, 0.001565959343117975886, 0.001957449178897469749, 0.002348939014676962745, 0.002740428850456455741, 0.003131918686235948303 ),
 .UNSPECIFIED. ) ;
#14955=CARTESIAN_POINT ( 'NONE',  ( 3.419318284370305161, -4.932111238568102962, 5.999920023562623328 ) ) ;
#14957=CARTESIAN_POINT ( 'NONE',  ( -3.312341048453446568, 5.004306261885469453, 30.02601979877761451 ) ) ;
#14958=DIRECTION ( 'NONE',  ( 0.9510565162951499785, 0.3090169943749582204, 0.000000000000000000 ) ) ;
#14966=ORIENTED_EDGE ( 'NONE', *, *, #474, .T. ) ;
#14968=ORIENTED_EDGE ( 'NONE', *, *, #10709, .T. ) ;
#14970=CARTESIAN_POINT ( 'NONE',  ( -3.883588957979220879, 4.898466244118957036, 4.026227171247318104 ) ) ;
#14972=CARTESIAN_POINT ( 'NONE',  ( -5.131373506000823426, 7.062729720843950787, 17.99999999999998934 ) ) ;
#14975=CARTESIAN_POINT ( 'NONE',  ( 7.347881242120658060E-16, 6.000000000000000888, 4.000000000000004441 ) ) ;
#14976=CARTESIAN_POINT ( 'NONE',  ( -3.735642931251015320, -4.696778275484483345, 10.52591947216897239 ) ) ;
#14979=CARTESIAN_POINT ( 'NONE',  ( 6.155973317223302210, -1.081218830693633670, 10.99691356133952169 ) ) ;
#14983=EDGE_LOOP ( 'NONE', ( #6242, #13598, #15039, #3193 ) ) ;
#14986=CARTESIAN_POINT ( 'NONE',  ( 4.435347140101010943, 4.403429997944537710, 4.867658743658316745 ) ) ;
#14987=B_SPLINE_CURVE_WITH_KNOTS ( 'NONE', 3,
 ( #15368, #5665, #4464, #9395, #9318, #14233, #8208, #13045, #5822, #10664, #15524, #9725, #13211, #2551, #4786, #9952, #13287, #10907 ),
 .UNSPECIFIED., .F., .F.,
 ( 4, 2, 2, 2, 2, 2, 2, 2, 4 ),
 ( 0.003131918686235956543, 0.003523310662250248981, 0.003914702638264540985, 0.004306094614278833423, 0.004697486590293125860, 0.005088878566307418298, 0.005480270542321710736, 0.005871662518336003174, 0.006263054494350295612 ),
 .UNSPECIFIED. ) ;
#14989=CARTESIAN_POINT ( 'NONE',  ( -6.142844459177212890, -1.156093792145330479, 17.38439807107078749 ) ) ;
#14990=CARTESIAN_POINT ( 'NONE',  ( 0.9999502950802301449, -5.916088184763877322, 31.13108149190011176 ) ) ;
#14991=CARTESIAN_POINT ( 'NONE',  ( -5.317509234263968487, 2.779225709350972906, 5.130616955321390726 ) ) ;
#14994=EDGE_CURVE ( 'NONE', #11999, #14255, #3870, .T. ) ;
#14997=CARTESIAN_POINT ( 'NONE',  ( 5.747343991580207145, 1.727858744772199584, 18.99992002356260556 ) ) ;
#15006=ORIENTED_EDGE ( 'NONE', *, *, #3583, .F. ) ;
#15007=CARTESIAN_POINT ( 'NONE',  ( -6.172639027853111138, 0.9816353142772042961, 17.73774718278285434 ) ) ;
#15008=CARTESIAN_POINT ( 'NONE',  ( -6.155867707731091265, 1.081837891426014941, 23.99563030319847812 ) ) ;
#15009=CARTESIAN_POINT ( 'NONE',  ( -0.9735954530125274786, 6.173909381473990265, 5.262817935852436513 ) ) ;
#15010=CARTESIAN_POINT ( 'NONE',  ( 0.9737778612007512713, 5.920671847850482727, 24.23736375884649874 ) ) ;
#15012=CARTESIAN_POINT ( 'NONE',  ( -2.841519077896096590, -5.566940434250041925, 31.26379616840806719 ) ) ;
#15014=CARTESIAN_POINT ( 'NONE',  ( 3.922396193919041263, 4.541970110199453181, 4.126193172852894442 ) ) ;
#15016=DIRECTION ( 'NONE',  ( 0.000000000000000000, 1.000000000000000000, 0.000000000000000000 ) ) ;
#15020=CARTESIAN_POINT ( 'NONE',  ( 4.290381260516221928, 4.545736887716255836, 12.11517780375842790 ) ) ;
#15023=CARTESIAN_POINT ( 'NONE',  ( 5.558508435838292350, -2.857531096718732844, 18.13237410716305220 ) ) ;
#15028=CARTESIAN_POINT ( 'NONE',  ( -5.408775798201205021, 2.598833957129572436, 4.386022610569177083 ) ) ;
#15032=CARTESIAN_POINT ( 'NONE',  ( 5.487097279078464673, -2.429065649168742347, 10.70047945897284336 ) ) ;
#15033=FACE_OUTER_BOUND ( 'NONE', #12311, .T. ) ;
#15035=DIRECTION ( 'NONE',  ( -0.3090169943749584425, 0.9510565162951498674, 0.000000000000000000 ) ) ;
#15036=VERTEX_POINT ( 'NONE', #3704 ) ;
#15039=ORIENTED_EDGE ( 'NONE', *, *, #13485, .T. ) ;
#15040=CARTESIAN_POINT ( 'NONE',  ( -5.940390500375820615, 6.474944468551430354, 24.49999999999999289 ) ) ;
#15042=DIRECTION ( 'NONE',  ( -0.3090169943749584425, 0.9510565162951498674, 0.000000000000000000 ) ) ;
#15044=VERTEX_POINT ( 'NONE', #13333 ) ;
#15045=CARTESIAN_POINT ( 'NONE',  ( -5.486741141153769874, -2.429871531109777383, 30.20111757752059134 ) ) ;
#15046=CARTESIAN_POINT ( 'NONE',  ( -4.154121946520915820, 4.670585111242934850, 4.201121615766615136 ) ) ;
#15047=FACE_OUTER_BOUND ( 'NONE', #4332, .T. ) ;
#15051=CARTESIAN_POINT ( 'NONE',  ( -2.692693252389710690, 5.362085866495045927, 17.73617396794403689 ) ) ;
#15059=VERTEX_POINT ( 'NONE', #12216 ) ;
#15061=CARTESIAN_POINT ( 'NONE',  ( 4.416397290909928941, -4.422724436066409304, 11.76379616840804232 ) ) ;
#15062=CARTESIAN_POINT ( 'NONE',  ( 6.081590040723058976, 1.446205118473082862, 4.126326713640078303 ) ) ;
#15065=CARTESIAN_POINT ( 'NONE',  ( 0.2622538972265521795, -6.245673238944470462, 18.97385994369199480 ) ) ;
#15066=CARTESIAN_POINT ( 'NONE',  ( -5.620879908643986234, 2.102487719021839840, 5.973778239432934178 ) ) ;
#15067=CARTESIAN_POINT ( 'NONE',  ( 0.8738239080081156018, 6.188820299975580141, 18.50355795710150986 ) ) ;
#15071=CARTESIAN_POINT ( 'NONE',  ( -3.779082820360787132, 4.979770177899181860, 19.00004906876531763 ) ) ;
#15076=EDGE_LOOP ( 'NONE', ( #882, #2145, #11222, #12625 ) ) ;
#15078=EDGE_CURVE ( 'NONE', #6002, #6522, #8821, .T. ) ;
#15080=CARTESIAN_POINT ( 'NONE',  ( -2.841519077896279999, 5.566940434249946890, 17.73620383159192926 ) ) ;
#15081=CARTESIAN_POINT ( 'NONE',  ( -5.984595133899138553, 1.806709459528792916, 23.50004921015706216 ) ) ;
#15083=CARTESIAN_POINT ( 'NONE',  ( -0.8002720181890968787, 6.199262377003405433, 4.386062624655573394 ) ) ;
#15084=CARTESIAN_POINT ( 'NONE',  ( 5.649200442566169933, 2.675373855294122638, 12.11560192892920718 ) ) ;
#15086=CARTESIAN_POINT ( 'NONE',  ( -3.459447313391792012, -5.206669755181024151, 31.97400098023329917 ) ) ;
#15087=CARTESIAN_POINT ( 'NONE',  ( -4.344762547369755090, -4.493114738039176714, 18.50308643866044278 ) ) ;
#15089=CARTESIAN_POINT ( 'NONE',  ( -3.634089073485383903, -4.776071126502727360, 31.99992002356261978 ) ) ;
#15091=CARTESIAN_POINT ( 'NONE',  ( -7.490007020835705909, -2.433650805992367161, 5.000000000000004441 ) ) ;
#15094=FACE_BOUND ( 'NONE', #9268, .T. ) ;
#15095=B_SPLINE_CURVE_WITH_KNOTS ( 'NONE', 3,
 ( #8243, #10781, #3538, #9831, #3846, #8493, #8799, #3922, #37, #271, #12360, #2742, #9678, #9987, #6256, #14836, #1381, #12049 ),
 .UNSPECIFIED., .F., .F.,
 ( 4, 2, 2, 2, 2, 2, 2, 2, 4 ),
 ( 0.000000000000000000, 0.0003914904498596255512, 0.0007829808997192511024, 0.001174471349578876545, 0.001565961799438502205, 0.001957452249298127864, 0.002348942699157753090, 0.002740433149017378750, 0.003131923598877004410 ),
 .UNSPECIFIED. ) ;
#15099=CARTESIAN_POINT ( 'NONE',  ( -5.487348639458818234, -2.428538342494575453, 18.80022217383878669 ) ) ;
#15103=CARTESIAN_POINT ( 'NONE',  ( -4.286401442266628337, -4.198423832313095794, 17.99999999999998934 ) ) ;
#15104=CARTESIAN_POINT ( 'NONE',  ( 5.903230462362985875, -1.077253041748709173, 17.38557478428062097 ) ) ;
#15108=FACE_OUTER_BOUND ( 'NONE', #6941, .T. ) ;
#15109=CARTESIAN_POINT ( 'NONE',  ( -5.866984344570842502, -1.259800266528583013, 5.799318062581741984 ) ) ;
#15111=CARTESIAN_POINT ( 'NONE',  ( 5.770331821586412779, -2.404225004693576029, 5.873800552473965375 ) ) ;
#15113=DIRECTION ( 'NONE',  ( 0.9510565162951500895, 0.3090169943749582204, 0.000000000000000000 ) ) ;
#15117=CARTESIAN_POINT ( 'NONE',  ( -5.903057025253874102, -1.078199533779696573, 23.88438267301394191 ) ) ;
#15118=ADVANCED_FACE ( 'NONE', ( #5068 ), #4178, .F. ) ;
#15120=FACE_OUTER_BOUND ( 'NONE', #10185, .T. ) ;
#15122=CARTESIAN_POINT ( 'NONE',  ( -3.420311045507748116, -4.931422832349356966, 6.000079611744768115 ) ) ;
#15123=CARTESIAN_POINT ( 'NONE',  ( -4.435347140101074004, 4.403429997944470209, 4.869393092765016640 ) ) ;
#15124=CARTESIAN_POINT ( 'NONE',  ( -4.435347140101009167, -4.403429997944534158, 5.130606907234994019 ) ) ;
#15126=EDGE_CURVE ( 'NONE', #10812, #10806, #2338, .T. ) ;
#15127=CARTESIAN_POINT ( 'NONE',  ( -6.172639027853119131, -0.9816353142771574447, 5.262252817217141221 ) ) ;
#15131=FACE_OUTER_BOUND ( 'NONE', #8695, .T. ) ;
#15135=ORIENTED_EDGE ( 'NONE', *, *, #7132, .F. ) ;
#15137=CARTESIAN_POINT ( 'NONE',  ( -6.105861027178945299, -1.337741388557017963, 10.70045537531157542 ) ) ;
#15139=AXIS2_PLACEMENT_3D ( 'NONE', #1956, #2034, #12773 ) ;
#15145=CARTESIAN_POINT ( 'NONE',  ( -5.317509234263969375, 2.779225709350973350, 5.000000000000004441 ) ) ;
#15150=CARTESIAN_POINT ( 'NONE',  ( 5.867109477881248480, 1.259218163100889631, 18.79888242247938734 ) ) ;
#15154=VERTEX_POINT ( 'NONE', #7760 ) ;
#15157=CARTESIAN_POINT ( 'NONE',  ( 2.930600586413043107, -5.520563544161711356, 5.503086438660451662 ) ) ;
#15159=DIRECTION ( 'NONE',  ( 0.9510565162951499785, 0.3090169943749582204, 0.000000000000000000 ) ) ;
#15161=CARTESIAN_POINT ( 'NONE',  ( -7.799024015210601846, -1.482594289697409140, 24.49999999999999289 ) ) ;
#15164=CARTESIAN_POINT ( 'NONE',  ( 3.779681992289775749, -4.979315417303914693, 17.00004921015705506 ) ) ;
#15167=CARTESIAN_POINT ( 'NONE',  ( -4.435347140101024266, -4.403429997944519947, 31.00000000000000000 ) ) ;
#15170=FACE_BOUND ( 'NONE', #13046, .T. ) ;
#15171=CARTESIAN_POINT ( 'NONE',  ( 0.7988860301924620710, 6.199427171881305654, 23.88455580536198397 ) ) ;
#15174=CARTESIAN_POINT ( 'NONE',  ( 1.353717517954364224E-13, -6.250000000000000888, 17.99999999999998934 ) ) ;
#15177=EDGE_CURVE ( 'NONE', #1121, #12191, #9546, .T. ) ;
#15179=B_SPLINE_CURVE_WITH_KNOTS ( 'NONE', 3,
 ( #8043, #14075, #3496, #15520, #8204, #10432, #2300, #8368, #9472, #3257, #4459, #5818, #13040, #4702, #4386, #10508, #11925, #13117 ),
 .UNSPECIFIED., .F., .F.,
 ( 4, 2, 2, 2, 2, 2, 2, 2, 4 ),
 ( 0.003131486019301986824, 0.003522824630466693530, 0.003914163241631400669, 0.004305501852796107809, 0.004696840463960814081, 0.005088179075125520354, 0.005479517686290226626, 0.005870856297454932898, 0.006262194908619639171 ),
 .UNSPECIFIED. ) ;
#15180=CARTESIAN_POINT ( 'NONE',  ( 5.317509234264033324, -2.779225709350853002, 17.86763921416088152 ) ) ;
#15182=CARTESIAN_POINT ( 'NONE',  ( -5.842945980534631545, 1.369128644669023176, 23.62621569129737509 ) ) ;
#15184=EDGE_CURVE ( 'NONE', #7351, #3463, #8810, .T. ) ;
#15189=CARTESIAN_POINT ( 'NONE',  ( 6.155973317223325303, -1.081218830693501998, 23.99691356133952169 ) ) ;
#15190=CARTESIAN_POINT ( 'NONE',  ( -6.081464507797648800, 1.446657058464131840, 4.126199447526042619 ) ) ;
#15191=CARTESIAN_POINT ( 'NONE',  ( -3.107688324358644838, -5.133887830459872958, 30.12621569129737154 ) ) ;
#15192=ORIENTED_EDGE ( 'NONE', *, *, #10955, .T. ) ;
#15196=CARTESIAN_POINT ( 'NONE',  ( 3.010624175977964612, 5.190832888732229478, 30.20111757752060200 ) ) ;
#15199=CARTESIAN_POINT ( 'NONE',  ( -5.131373506000715068, 7.062729720844030723, 5.000000000000004441 ) ) ;
#15200=CARTESIAN_POINT ( 'NONE',  ( -5.317509234263919637, -2.779225709351067053, 30.86938304467861016 ) ) ;
#15201=CARTESIAN_POINT ( 'NONE',  ( 1.354942165200771727E-13, 6.000000000000000888, 16.99999999999998579 ) ) ;
#15210=EDGE_LOOP ( 'NONE', ( #5, #6148 ) ) ;
#15213=EDGE_LOOP ( 'NONE', ( #3967, #2148, #9171, #6243 ) ) ;
#15214=CARTESIAN_POINT ( 'NONE',  ( -6.172552660730974416, -0.9821660343539097004, 11.23620383159194880 ) ) ;
#15218=CARTESIAN_POINT ( 'NONE',  ( -5.935543223013843850, -0.8771126767607685393, 31.13239388001635177 ) ) ;
#15222=CARTESIAN_POINT ( 'NONE',  ( -4.291255145204149635, 4.544933371694606095, 18.61396179408071561 ) ) ;
#15233=CARTESIAN_POINT ( 'NONE',  ( -0.1306394121198675706, 6.250000000000001776, 10.49999999999998579 ) ) ;
#15234=B_SPLINE_CURVE_WITH_KNOTS ( 'NONE', 3,
 ( #3840, #12353, #1449, #7430, #6327, #3995, #4079, #8713, #6485, #9825, #8640, #2655, #6408, #13546, #5127, #1685, #13472, #9979 ),
 .UNSPECIFIED., .F., .F.,
 ( 4, 2, 2, 2, 2, 2, 2, 2, 4 ),
 ( 0.003131490185286086615, 0.003522829482338686678, 0.003914168779391286740, 0.004305508076443887236, 0.004696847373496487732, 0.005088186670549088228, 0.005479525967601688724, 0.005870865264654288353, 0.006262204561706888849 ),
 .UNSPECIFIED. ) ;
#15236=CARTESIAN_POINT ( 'NONE',  ( 6.155912734541151288, 1.081577393120788821, 23.99610786875030044 ) ) ;
#15238=CYLINDRICAL_SURFACE ( 'NONE', #8435, 1.000000000000000222 ) ;
#15239=FACE_BOUND ( 'NONE', #12643, .T. ) ;
#15240=CARTESIAN_POINT ( 'NONE',  ( 3.159612573729182028, -5.393342049074657751, 17.19973484982323697 ) ) ;
#15242=CARTESIAN_POINT ( 'NONE',  ( -3.736532060717939085, -4.696070028786012429, 31.97377823943293151 ) ) ;
#15243=SHAPE_REPRESENTATION_RELATIONSHIP ( 'NONE' , 'NONE' ,  #9569, #4039 ) ;
#15244=LINE ( 'NONE', #4344, #7012 ) ;
#15248=CARTESIAN_POINT ( 'NONE',  ( 1.353717517954364224E-13, -6.250000000000000888, 17.99999999999998934 ) ) ;
#15249=CARTESIAN_POINT ( 'NONE',  ( 0.6156133477427582212, 6.220296490279936030, 25.29872387345520579 ) ) ;
#15253=CARTESIAN_POINT ( 'NONE',  ( 2.996920846510414460, -5.485395142346829900, 25.11441947245483419 ) ) ;
#15262=CARTESIAN_POINT ( 'NONE',  ( -0.2619456584321807613, 5.995505046955615924, 30.02607193928647433 ) ) ;
#15263=B_SPLINE_CURVE_WITH_KNOTS ( 'NONE', 3,
 ( #13471, #2573, #5048, #6325, #11008, #7429, #8871, #10055, #3839, #2654, #10135, #8638, #263, #7507, #5202, #13702, #14986, #14904 ),
 .UNSPECIFIED., .F., .F.,
 ( 4, 2, 2, 2, 2, 2, 2, 2, 4 ),
 ( 0.003131486019301986824, 0.003522824630466693096, 0.003914163241631399802, 0.004305501852796106074, 0.004696840463960812347, 0.005088179075125518619, 0.005479517686290224891, 0.005870856297454931164, 0.006262194908619637436 ),
 .UNSPECIFIED. ) ;
#15265=CARTESIAN_POINT ( 'NONE',  ( 5.984377695197236946, -1.807429553002246614, 6.000049068765331839 ) ) ;
#15268=VERTEX_POINT ( 'NONE', #10462 ) ;
#15272=B_SPLINE_CURVE_WITH_KNOTS ( 'NONE', 3,
 ( #1268, #14482, #14395, #10981, #2303, #6062, #6223, #2385, #9640, #3656, #3500, #12011, #9557, #4785, #9797, #12090, #4705, #8371 ),
 .UNSPECIFIED., .F., .F.,
 ( 4, 2, 2, 2, 2, 2, 2, 2, 4 ),
 ( 0.000000000000000000, 0.0003914357524127468893, 0.0007828715048254937785, 0.001174307257238240559, 0.001565743009650987557, 0.001957178762063732820, 0.002348614514476478517, 0.002740050266889223780, 0.003131486019301969476 ),
 .UNSPECIFIED. ) ;
#15273=ORIENTED_EDGE ( 'NONE', *, *, #6110, .T. ) ;
#15277=CARTESIAN_POINT ( 'NONE',  ( -5.935543223013844738, -0.8771126767607686503, 30.86763921416089573 ) ) ;
#15281=CARTESIAN_POINT ( 'NONE',  ( -2.997753866155722591, -5.484939622623898003, 5.615601928929210729 ) ) ;
#15283=CARTESIAN_POINT ( 'NONE',  ( 3.922288969639810663, -4.542045818322500317, 10.62621569129736976 ) ) ;
#15286=CARTESIAN_POINT ( 'NONE',  ( -5.409007216690611131, -2.598315788643874136, 17.38557478428061742 ) ) ;
#15287=CARTESIAN_POINT ( 'NONE',  ( 5.131373506000546314, 7.062729720844130199, 11.49999999999998224 ) ) ;
#15289=B_SPLINE_CURVE_WITH_KNOTS ( 'NONE', 3,
 ( #12612, #1708, #520, #13962, #5470, #5391, #10238, #15242, #15089, #4184, #9055, #13880, #4582, #15486, #13244, #4498, #8083, #12923 ),
 .UNSPECIFIED., .F., .F.,
 ( 4, 2, 2, 2, 2, 2, 2, 2, 4 ),
 ( 0.003131918686235972155, 0.003523310662250262858, 0.003914702638264553995, 0.004306094614278844698, 0.004697486590293134534, 0.005088878566307424370, 0.005480270542321714206, 0.005871662518336004041, 0.006263054494350293010 ),
 .UNSPECIFIED. ) ;
#15291=ORIENTED_EDGE ( 'NONE', *, *, #8070, .F. ) ;
#15293=CARTESIAN_POINT ( 'NONE',  ( 3.780072143464223711, -4.979057943639742412, 12.50008219321555103 ) ) ;
#15294=DIRECTION ( 'NONE',  ( 0.000000000000000000, 0.000000000000000000, 1.000000000000000000 ) ) ;
#15295=ORIENTED_EDGE ( 'NONE', *, *, #7586, .F. ) ;
#15299=CARTESIAN_POINT ( 'NONE',  ( 6.106056299406759535, 1.336851112280623921, 18.79887838423337598 ) ) ;
#15305=AXIS2_PLACEMENT_3D ( 'NONE', #1280, #9886, #12182 ) ;
#15306=CARTESIAN_POINT ( 'NONE',  ( -5.931734679891446760, -0.9039278060244212432, 4.736173967944048435 ) ) ;
#15309=ORIENTED_EDGE ( 'NONE', *, *, #2500, .T. ) ;
#15312=FACE_OUTER_BOUND ( 'NONE', #14735, .T. ) ;
#15318=VERTEX_POINT ( 'NONE', #11798 ) ;
#15320=FACE_BOUND ( 'NONE', #5767, .T. ) ;
#15321=B_SPLINE_CURVE_WITH_KNOTS ( 'NONE', 3,
 ( #7527, #3936, #12689, #1787, #6661, #1632, #596, #4260, #5388, #6508, #14927, #8812, #4019, #8895, #11341, #438, #10235, #9128 ),
 .UNSPECIFIED., .F., .F.,
 ( 4, 2, 2, 2, 2, 2, 2, 2, 4 ),
 ( 0.000000000000000000, 0.0003914357524127489493, 0.0007828715048254978985, 0.001174307257238246848, 0.001565743009650994713, 0.001957178762063743228, 0.002348614514476490660, 0.002740050266889238959, 0.003131486019301986824 ),
 .UNSPECIFIED. ) ;
#15323=CARTESIAN_POINT ( 'NONE',  ( -4.416678568553779272, -4.422441866694181378, 24.76236973443873168 ) ) ;
#15326=EDGE_CURVE ( 'NONE', #5344, #11668, #4816, .T. ) ;
#15328=FACE_BOUND ( 'NONE', #11960, .T. ) ;
#15330=CARTESIAN_POINT ( 'NONE',  ( 0.2623718222037388359, 6.245654667075775990, 23.52627829713835439 ) ) ;
#15341=EDGE_CURVE ( 'NONE', #6786, #6278, #7267, .T. ) ;
#15344=DIRECTION ( 'NONE',  ( 0.8090169943749421222, 0.5877852522924802425, 0.000000000000000000 ) ) ;
#15347=FACE_BOUND ( 'NONE', #10386, .T. ) ;
#15348=CARTESIAN_POINT ( 'NONE',  ( 2.082642335314403343E-14, 6.000000000000000888, 32.00000000000000000 ) ) ;
#15350=B_SPLINE_CURVE_WITH_KNOTS ( 'NONE', 3,
 ( #6670, #11503, #604, #13969, #3077, #7925, #7744, #13859, #6489, #13624, #577, #13709, #12671, #4240, #5293, #2817, #6412, #7666 ),
 .UNSPECIFIED., .F., .F.,
 ( 4, 2, 2, 2, 2, 2, 2, 2, 4 ),
 ( 0.003131486019301976849, 0.003522824630466684856, 0.003914163241631392863, 0.004305501852796100870, 0.004696840463960809745, 0.005088179075125516884, 0.005479517686290225759, 0.005870856297454933766, 0.006262194908619641773 ),
 .UNSPECIFIED. ) ;
#15351=EDGE_CURVE ( 'NONE', #11236, #8072, #5383, .T. ) ;
#15352=ORIENTED_EDGE ( 'NONE', *, *, #4948, .T. ) ;
#15354=CARTESIAN_POINT ( 'NONE',  ( 4.141923667210638094, 4.342011609040473452, 30.38438267301394902 ) ) ;
#15355=VERTEX_POINT ( 'NONE', #3607 ) ;
#15356=CARTESIAN_POINT ( 'NONE',  ( -4.286401442266532413, -4.198423832313194382, 4.869350386511452911 ) ) ;
#15358=DIRECTION ( 'NONE',  ( -0.9510565162951545304, 0.3090169943749447867, 0.000000000000000000 ) ) ;
#15359=CARTESIAN_POINT ( 'NONE',  ( 5.935543223013868719, 0.8771126767606117758, 17.86935038651144936 ) ) ;
#15361=CARTESIAN_POINT ( 'NONE',  ( 5.931793676715125585, -0.9035324301686619153, 24.23760108194402108 ) ) ;
#15365=DIRECTION ( 'NONE',  ( -0.9510565162951544194, 0.3090169943749447312, 0.000000000000000000 ) ) ;
#15366=CARTESIAN_POINT ( 'NONE',  ( 4.153663429050758360, 4.670992970568392799, 31.79933148907576523 ) ) ;
#15368=CARTESIAN_POINT ( 'NONE',  ( 5.935543223013856284, 0.8771126767606806096, 11.49999999999998224 ) ) ;
#15369=AXIS2_PLACEMENT_3D ( 'NONE', #6629, #5508, #3035 ) ;
#15370=VERTEX_POINT ( 'NONE', #7282 ) ;
#15373=CARTESIAN_POINT ( 'NONE',  ( -6.020865209844587618, -1.681180471732168780, 10.52599901976669194 ) ) ;
#15374=CARTESIAN_POINT ( 'NONE',  ( 5.558508435838190209, 2.857531096718933128, 4.867625892836953128 ) ) ;
#15375=ORIENTED_EDGE ( 'NONE', *, *, #13774, .F. ) ;
#15377=CARTESIAN_POINT ( 'NONE',  ( -5.866984344570836285, -1.259800266528611878, 31.79931806258174376 ) ) ;
#15381=DIRECTION ( 'NONE',  ( -0.3090169943749579429, 0.9510565162951502005, 0.000000000000000000 ) ) ;
#15385=CARTESIAN_POINT ( 'NONE',  ( 4.435347140101073116, -4.403429997944470209, 5.000000000000004441 ) ) ;
#15389=B_SPLINE_CURVE_WITH_KNOTS ( 'NONE', 3,
 ( #6623, #15123, #2873, #629, #400, #15046, #11224, #14970, #12416, #10346, #5186, #10040, #12571, #13764, #2953, #12723, #2795, #7800 ),
 .UNSPECIFIED., .F., .F.,
 ( 4, 2, 2, 2, 2, 2, 2, 2, 4 ),
 ( 0.003131486019301987257, 0.003522824630466693530, 0.003914163241631399802, 0.004305501852796106074, 0.004696840463960813214, 0.005088179075125520354, 0.005479517686290226626, 0.005870856297454934633, 0.006262194908619640905 ),
 .UNSPECIFIED. ) ;
#15390=ORIENTED_EDGE ( 'NONE', *, *, #12497, .T. ) ;
#15393=VERTEX_POINT ( 'NONE', #15553 ) ;
#15394=CARTESIAN_POINT ( 'NONE',  ( 3.882809187879016299, -4.899079348629983954, 5.974000980233302727 ) ) ;
#15395=CARTESIAN_POINT ( 'NONE',  ( 4.286401442266496886, -4.198423832313229020, 17.99999999999998934 ) ) ;
#15398=CARTESIAN_POINT ( 'NONE',  ( -5.842945980534647532, 1.369128644668957451, 17.12621569129737154 ) ) ;
#15399=FACE_BOUND ( 'NONE', #4649, .T. ) ;
#15406=DIRECTION ( 'NONE',  ( 0.000000000000000000, 1.000000000000000000, 0.000000000000000000 ) ) ;
#15407=CARTESIAN_POINT ( 'NONE',  ( 0.7995524673976757146, 6.199337389817257460, 25.11453679452471732 ) ) ;
#15410=CARTESIAN_POINT ( 'NONE',  ( 4.416397290909830353, -4.422724436066506115, 24.76379616840805653 ) ) ;
#15414=CARTESIAN_POINT ( 'NONE',  ( -4.435347140101074004, 4.403429997944469321, 5.000000000000004441 ) ) ;
#15419=DIRECTION ( 'NONE',  ( -0.9510565162951545304, 0.3090169943749447867, 0.000000000000000000 ) ) ;
#15420=CARTESIAN_POINT ( 'NONE',  ( -0.7993282387950892964, 5.947240459526512701, 31.61484358216958057 ) ) ;
#15424=CARTESIAN_POINT ( 'NONE',  ( 5.558508435838221295, 2.857531096718871844, 11.36762589283694247 ) ) ;
#15431=EDGE_CURVE ( 'NONE', #12139, #10038, #3085, .T. ) ;
#15433=EDGE_CURVE ( 'NONE', #3038, #2035, #15234, .T. ) ;
#15434=CARTESIAN_POINT ( 'NONE',  ( -2.668367453516630849, -5.373994336898132218, 5.000000000000004441 ) ) ;
#15436=EDGE_CURVE ( 'NONE', #4624, #6402, #8017, .T. ) ;
#15437=CARTESIAN_POINT ( 'NONE',  ( 4.416397290909816142, 4.422724436066522102, 17.73620383159193281 ) ) ;
#15439=CARTESIAN_POINT ( 'NONE',  ( -4.344762547369660943, -4.493114738039267309, 5.503086438660448110 ) ) ;
#15443=CARTESIAN_POINT ( 'NONE',  ( 5.859155363331435495, -2.178872204144838509, 17.02599901976669017 ) ) ;
#15444=CARTESIAN_POINT ( 'NONE',  ( 0.8002720181891173068, -6.199262377003402769, 30.38606262465556895 ) ) ;
#15448=AXIS2_PLACEMENT_3D ( 'NONE', #14947, #7702, #9940 ) ;
#15450=ORIENTED_EDGE ( 'NONE', *, *, #13085, .T. ) ;
#15451=ORIENTED_EDGE ( 'NONE', *, *, #5331, .T. ) ;
#15454=VERTEX_POINT ( 'NONE', #5204 ) ;
#15456=AXIS2_PLACEMENT_3D ( 'NONE', #3236, #11748, #11817 ) ;
#15457=CARTESIAN_POINT ( 'NONE',  ( 0.9740807849836119470, -5.920620690450689949, 4.738501197006694809 ) ) ;
#15458=CARTESIAN_POINT ( 'NONE',  ( 3.459597053047676507, 5.206576120509858185, 25.47408542334170889 ) ) ;
#15461=CYLINDRICAL_SURFACE ( 'NONE', #9741, 0.9999999999999998890 ) ;
#15469=ORIENTED_EDGE ( 'NONE', *, *, #5331, .F. ) ;
#15473=CARTESIAN_POINT ( 'NONE',  ( 1.000082492230738085, 6.169467968613703057, 31.13152538105391898 ) ) ;
#15475=CARTESIAN_POINT ( 'NONE',  ( 7.347881242120658060E-16, 6.000000000000000888, 4.000000000000004441 ) ) ;
#15476=EDGE_CURVE ( 'NONE', #14884, #15154, #14470, .T. ) ;
#15477=EDGE_LOOP ( 'NONE', ( #8771, #2450, #3969, #1646 ) ) ;
#15478=CARTESIAN_POINT ( 'NONE',  ( -5.621278735166202800, 2.101423246382537968, 17.02591947216897950 ) ) ;
#15479=CARTESIAN_POINT ( 'NONE',  ( 7.347880431581855163E-16, -6.250000000000000888, 4.000000000000004441 ) ) ;
#15482=FACE_BOUND ( 'NONE', #12158, .T. ) ;
#15486=CARTESIAN_POINT ( 'NONE',  ( -2.849573632035199644, -5.280958870664642646, 31.61561732698606875 ) ) ;
#15492=CARTESIAN_POINT ( 'NONE',  ( 5.782895619916161856, 1.604017620858061655, 10.52591947216897594 ) ) ;
#15496=CARTESIAN_POINT ( 'NONE',  ( -3.779082820360838646, 4.979770177899141004, 25.50004906876532473 ) ) ;
#15498=ORIENTED_EDGE ( 'NONE', *, *, #5166, .F. ) ;
#15499=CARTESIAN_POINT ( 'NONE',  ( -6.172552660730974416, 0.9821660343538980431, 18.26379616840806008 ) ) ;
#15502=CARTESIAN_POINT ( 'NONE',  ( 5.726049995854515906, 2.506679546901768418, 25.29954462468842991 ) ) ;
#15506=FACE_BOUND ( 'NONE', #9100, .T. ) ;
#15510=CARTESIAN_POINT ( 'NONE',  ( -5.558508435838095174, -2.857531096719115649, 24.49999999999999289 ) ) ;
#15512=ORIENTED_EDGE ( 'NONE', *, *, #6612, .F. ) ;
#15513=CARTESIAN_POINT ( 'NONE',  ( 7.490007020835728113, -2.433650805992114918, 17.99999999999998934 ) ) ;
#15515=CARTESIAN_POINT ( 'NONE',  ( -2.692215568229824108, 5.362327947133604944, 31.26229037835932090 ) ) ;
#15516=CARTESIAN_POINT ( 'NONE',  ( 5.329945432499631153, 2.755769831645132228, 17.73770962164070397 ) ) ;
#15518=CARTESIAN_POINT ( 'NONE',  ( 3.735808404764950463, -4.696639218303163332, 18.97398020122238549 ) ) ;
#15520=CARTESIAN_POINT ( 'NONE',  ( -5.615811513735010863, -2.743665920700458116, 4.496913561339539456 ) ) ;
#15522=CARTESIAN_POINT ( 'NONE',  ( 4.435347140101073116, -4.403429997944470209, 5.000000000000004441 ) ) ;
#15524=CARTESIAN_POINT ( 'NONE',  ( 5.621197618055705725, 2.101623592078435188, 12.47398020122238016 ) ) ;
#15526=VERTEX_POINT ( 'NONE', #14911 ) ;
#15529=CARTESIAN_POINT ( 'NONE',  ( 4.290130679986543072, 4.545972905167758427, 30.38439807107077684 ) ) ;
#15531=MANIFOLD_SOLID_BREP ( 'CirPattern1', #11307 ) ;
#15534=B_SPLINE_CURVE_WITH_KNOTS ( 'NONE', 3,
 ( #6795, #13707, #11324, #5520, #7821, #1612, #345, #6642, #12670, #10060, #12818, #14018, #5209, #3048, #13784, #11399, #8953, #5292 ),
 .UNSPECIFIED., .F., .F.,
 ( 4, 2, 2, 2, 2, 2, 2, 2, 4 ),
 ( 0.000000000000000000, 0.0003914357524127469435, 0.0007828715048254938870, 0.001174307257238240776, 0.001565743009650987774, 0.001957178762063734555, 0.002348614514476482420, 0.002740050266889230719, 0.003131486019301978150 ),
 .UNSPECIFIED. ) ;
#15536=CARTESIAN_POINT ( 'NONE',  ( 6.176542424588125968, 0.9554180641284963915, 17.99999999999998934 ) ) ;
#15544=CARTESIAN_POINT ( 'NONE',  ( 3.254737477228069942, -5.337033878705166323, 4.126326713640079191 ) ) ;
#15546=CARTESIAN_POINT ( 'NONE',  ( 3.779681992289694481, 4.979315417303977753, 18.99995078984292363 ) ) ;
#15550=EDGE_LOOP ( 'NONE', ( #6404, #4451, #2250, #1277 ) ) ;
#15551=CARTESIAN_POINT ( 'NONE',  ( -6.142844459177213778, 1.156093792145326260, 25.11560192892921606 ) ) ;
#15552=CARTESIAN_POINT ( 'NONE',  ( 1.353717517954364224E-13, -6.250000000000000888, 17.99999999999998934 ) ) ;
#15553=CARTESIAN_POINT ( 'NONE',  ( 2.094888798833199608E-14, -6.000000000000000888, 30.00000000000000000 ) ) ;
#15556=CARTESIAN_POINT ( 'NONE',  ( -5.858813228503671588, 2.179803269293220325, 31.97377282875268989 ) ) ;
#15557=CARTESIAN_POINT ( 'NONE',  ( -0.2637975869347825020, -6.245592211692892803, 5.973328399491914631 ) ) ;
#15558=FACE_BOUND ( 'NONE', #11621, .T. ) ;
#15564=CARTESIAN_POINT ( 'NONE',  ( 5.558508435838291462, -2.857531096718732400, 17.99999999999998934 ) ) ;
#15567=CARTESIAN_POINT ( 'NONE',  ( 5.375913338529070273, 2.664979843780479030, 31.50428920362020335 ) ) ;
#15568=VECTOR ( 'NONE', #7379, 1000.000000000000000 ) ;
#15569=ORIENTED_EDGE ( 'NONE', *, *, #11916, .T. ) ;
#15570=CARTESIAN_POINT ( 'NONE',  ( 7.799024015210693328, -1.482594289696895551, 24.49999999999999289 ) ) ;
#15571=CARTESIAN_POINT ( 'NONE',  ( 0.1306497350717998329, -6.000000000000000888, 10.49999999999998224 ) ) ;
#15573=VERTEX_POINT ( 'NONE', #7591 ) ;
#15581=CARTESIAN_POINT ( 'NONE',  ( -2.931156713028464811, 5.520271803279225509, 5.504369696801525436 ) ) ;
#15583=DIRECTION ( 'NONE',  ( 0.000000000000000000, 0.000000000000000000, -1.000000000000000000 ) ) ;
#15585=CARTESIAN_POINT ( 'NONE',  ( 0.9737778612005694168, 5.920671847850513814, 30.73736375884650585 ) ) ;
#15586=VERTEX_POINT ( 'NONE', #2819 ) ;
#15590=CARTESIAN_POINT ( 'NONE',  ( 5.782895619916200936, 1.604017620857918436, 23.52591947216898305 ) ) ;
#15591=EDGE_LOOP ( 'NONE', ( #14825, #4249 ) ) ;
#15593=B_SPLINE_CURVE_WITH_KNOTS ( 'NONE', 3,
 ( #4373, #9231, #14546, #3567, #141, #4692, #1177, #7161, #9859, #8673, #11998, #12078, #6131, #5006, #15669, #3485, #9709, #3643 ),
 .UNSPECIFIED., .F., .F.,
 ( 4, 2, 2, 2, 2, 2, 2, 2, 4 ),
 ( 0.003131486019301968609, 0.003522824630466677917, 0.003914163241631387659, 0.004305501852796097401, 0.004696840463960805408, 0.005088179075125514282, 0.005479517686290222289, 0.005870856297454931164, 0.006262194908619639171 ),
 .UNSPECIFIED. ) ;
#15595=CARTESIAN_POINT ( 'NONE',  ( 5.317509234263971152, -2.779225709350972906, 5.132393880016354437 ) ) ;
#15596=CARTESIAN_POINT ( 'NONE',  ( -4.143041610105363759, 4.340967609746979150, 31.61397738943081492 ) ) ;
#15597=CARTESIAN_POINT ( 'NONE',  ( 6.780834061396424457E-14, 6.250000000000000888, 10.49999999999998224 ) ) ;
#15599=CARTESIAN_POINT ( 'NONE',  ( 4.267936573529280686, -4.217499624512167422, 30.73770962164067200 ) ) ;
#15601=CARTESIAN_POINT ( 'NONE',  ( -6.250000000000000888, 0.000000000000000000, 36.00000000000000711 ) ) ;
#15606=ADVANCED_FACE ( 'NONE', ( #11327 ), #11246, .F. ) ;
#15608=ORIENTED_EDGE ( 'NONE', *, *, #7820, .T. ) ;
#15611=ORIENTED_EDGE ( 'NONE', *, *, #9262, .F. ) ;
#15613=CARTESIAN_POINT ( 'NONE',  ( -0.5039079366030397855, 5.980031194523169447, 23.62637068109811977 ) ) ;
#15614=CARTESIAN_POINT ( 'NONE',  ( 5.571002711501385818, 2.833546409886330775, 31.26379616840806719 ) ) ;
#15619=CARTESIAN_POINT ( 'NONE',  ( 4.322356511625540243, 7.650514973136639973, 17.99999999999998934 ) ) ;
#15621=LINE ( 'NONE', #7114, #7494 ) ;
#15624=LINE ( 'NONE', #1135, #9353 ) ;
#15625=ORIENTED_EDGE ( 'NONE', *, *, #734, .T. ) ;
#15626=EDGE_LOOP ( 'NONE', ( #4766, #12829, #12019, #10250 ) ) ;
#15627=CARTESIAN_POINT ( 'NONE',  ( 0.2623718222035403280, 6.245654667075782207, 30.02627829713834728 ) ) ;
#15628=VECTOR ( 'NONE', #2213, 1000.000000000000114 ) ;
#15630=CARTESIAN_POINT ( 'NONE',  ( -3.882673863916357160, -4.899192824800883805, 23.52591457665828401 ) ) ;
#15633=CARTESIAN_POINT ( 'NONE',  ( 3.106366801612014950, -5.134708448381275048, 12.37303779027049799 ) ) ;
#15634=B_SPLINE_CURVE_WITH_KNOTS ( 'NONE', 3,
 ( #10751, #2073, #13294, #6947, #9647, #7099, #14488, #14400, #14165, #5749, #9402, #3507, #3586, #6068, #4629, #8459, #3346, #7180 ),
 .UNSPECIFIED., .F., .F.,
 ( 4, 2, 2, 2, 2, 2, 2, 2, 4 ),
 ( 0.000000000000000000, 0.0003914898357794970073, 0.0007829796715589940146, 0.001174469507338490913, 0.001565959343117988029, 0.001957449178897484928, 0.002348939014676983128, 0.002740428850456480894, 0.003131918686235978661 ),
 .UNSPECIFIED. ) ;
#15635=CARTESIAN_POINT ( 'NONE',  ( -0.6156133477426863898, -6.220296490279942248, 5.798723873455115196 ) ) ;
#15636=CARTESIAN_POINT ( 'NONE',  ( -0.6156133477424821088, -6.220296490279960011, 25.29872387345510987 ) ) ;
#15638=CARTESIAN_POINT ( 'NONE',  ( 5.782895619916152086, 1.604017620858103177, 30.02591947216899371 ) ) ;
#15639=CARTESIAN_POINT ( 'NONE',  ( -3.459447313391949663, -5.206669755180918457, 25.47400098023329562 ) ) ;
#15644=CARTESIAN_POINT ( 'NONE',  ( 4.142173849413740783, 4.341773579105408842, 31.61519382448851090 ) ) ;
#15646=ORIENTED_EDGE ( 'NONE', *, *, #12732, .T. ) ;
#15647=CARTESIAN_POINT ( 'NONE',  ( -3.923477796648561888, 4.541042560386441274, 4.126962209729494901 ) ) ;
#15648=CARTESIAN_POINT ( 'NONE',  ( 0.8736516769107610658, -5.936271176698223684, 10.99606771578675612 ) ) ;
#15649=CARTESIAN_POINT ( 'NONE',  ( 5.747343991580224021, 1.727858744772142741, 25.49992002356261622 ) ) ;
#15651=CARTESIAN_POINT ( 'NONE',  ( 0.1306171417090646603, 5.999999999999993783, 23.49999999999999289 ) ) ;
#15653=CARTESIAN_POINT ( 'NONE',  ( -4.416678568553646933, -4.422441866694312829, 31.26236973443874945 ) ) ;
#15657=CARTESIAN_POINT ( 'NONE',  ( -6.172552660730985963, 0.9821660343538300975, 11.76379616840804943 ) ) ;
#15659=CARTESIAN_POINT ( 'NONE',  ( -3.567624405365297680, 5.133384272590741482, 5.999950789842938725 ) ) ;
#15661=EDGE_CURVE ( 'NONE', #4525, #15318, #14095, .T. ) ;
#15662=CARTESIAN_POINT ( 'NONE',  ( -2.692693252389608993, 5.362085866495096553, 30.73617396794405821 ) ) ;
#15664=CARTESIAN_POINT ( 'NONE',  ( 5.770331821586426102, 2.404225004693546275, 17.12619944752603729 ) ) ;
#15667=ADVANCED_FACE ( 'NONE', ( #307 ), #14869, .F. ) ;
#15669=CARTESIAN_POINT ( 'NONE',  ( -2.931212650151639565, -5.520239928492829407, 12.00425949503009093 ) ) ;
#15671=CARTESIAN_POINT ( 'NONE',  ( -3.632151824461158363, -4.777505256984540871, 23.49995067926686687 ) ) ;
#15672=B_SPLINE_CURVE_WITH_KNOTS ( 'NONE', 3,
 ( #10851, #9672, #10695, #15715, #13390, #14593, #4815, #15556, #13473, #11876, #4655, #9508, #1296, #14342, #3608, #8316, #32, #419 ),
 .UNSPECIFIED., .F., .F.,
 ( 4, 2, 2, 2, 2, 2, 2, 2, 4 ),
 ( 0.003131486019301988125, 0.003522824630466695264, 0.003914163241631402404, 0.004305501852796108676, 0.004696840463960815816, 0.005088179075125522956, 0.005479517686290229228, 0.005870856297454936368, 0.006262194908619643507 ),
 .UNSPECIFIED. ) ;
#15678=CARTESIAN_POINT ( 'NONE',  ( 2.782468714962443190, -5.316055268221400176, 30.49610204984016448 ) ) ;
#15680=LINE ( 'NONE', #4942, #4787 ) ;
#15681=CARTESIAN_POINT ( 'NONE',  ( -6.000000000000000888, 0.000000000000000000, 0.000000000000000000 ) ) ;
#15683=CARTESIAN_POINT ( 'NONE',  ( 5.317509234263932960, 2.779225709351047069, 4.867606119983654445 ) ) ;
#15687=ORIENTED_EDGE ( 'NONE', *, *, #14615, .F. ) ;
#15688=B_SPLINE_CURVE_WITH_KNOTS ( 'NONE', 3,
 ( #2675, #5949, #15653, #284, #5466, #1706, #10158, #12373, #12610, #5231, #15086, #1554, #13802, #13731, #2837, #15012, #6352, #12455 ),
 .UNSPECIFIED., .F., .F.,
 ( 4, 2, 2, 2, 2, 2, 2, 2, 4 ),
 ( 0.003131486019301990293, 0.003522824630466696565, 0.003914163241631402404, 0.004305501852796108676, 0.004696840463960814949, 0.005088179075125520354, 0.005479517686290227493, 0.005870856297454932898, 0.006262194908619639171 ),
 .UNSPECIFIED. ) ;
#15690=VERTEX_POINT ( 'NONE', #5563 ) ;
#15692=CARTESIAN_POINT ( 'NONE',  ( 5.859155363331417732, 2.178872204144886471, 18.97400098023329562 ) ) ;
#15694=CARTESIAN_POINT ( 'NONE',  ( 6.081836621194427472, 1.445163676684881882, 31.87305891554300530 ) ) ;
#15697=AXIS2_PLACEMENT_3D ( 'NONE', #11204, #12392, #2854 ) ;
#15701=CARTESIAN_POINT ( 'NONE',  ( 3.568242062701590722, -5.132954954975464723, 29.99995093123466816 ) ) ;
#15704=VERTEX_POINT ( 'NONE', #7783 ) ;
#15705=VERTEX_POINT ( 'NONE', #10409 ) ;
#15708=ORIENTED_EDGE ( 'NONE', *, *, #2897, .F. ) ;
#15710=CARTESIAN_POINT ( 'NONE',  ( -6.172552660730978857, -0.9821660343538717308, 30.73620383159192571 ) ) ;
#15712=CARTESIAN_POINT ( 'NONE',  ( 3.421280866381102292, -4.930711975950938353, 16.99995067926686687 ) ) ;
#15713=B_SPLINE_CURVE_WITH_KNOTS ( 'NONE', 3,
 ( #8180, #13096, #4281, #14053, #3318, #5561, #15182, #3161, #2039, #8018, #2193, #12856, #613, #924, #1961, #689, #10329, #7937 ),
 .UNSPECIFIED., .F., .F.,
 ( 4, 2, 2, 2, 2, 2, 2, 2, 4 ),
 ( 0.000000000000000000, 0.0003914898357794970615, 0.0007829796715589941230, 0.001174469507338491130, 0.001565959343117988246, 0.001957449178897485362, 0.002348939014676982261, 0.002740428850456479593, 0.003131918686235976492 ),
 .UNSPECIFIED. ) ;
#15714=CARTESIAN_POINT ( 'NONE',  ( -3.736532060718080306, -4.696070028785897854, 25.47377823943292796 ) ) ;
#15715=CARTESIAN_POINT ( 'NONE',  ( -5.615811513735035732, 2.743665920700399496, 31.50308643866046054 ) ) ;
#15716=B_SPLINE_CURVE_WITH_KNOTS ( 'NONE', 3,
 ( #7298, #3626, #14526, #12291, #3548, #2353, #6265, #11027, #15649, #12215, #8332, #13411, #12138, #2519, #14612, #1239, #13331, #6111 ),
 .UNSPECIFIED., .F., .F.,
 ( 4, 2, 2, 2, 2, 2, 2, 2, 4 ),
 ( 0.003131918686235976058, 0.003523310662250265460, 0.003914702638264554863, 0.004306094614278844698, 0.004697486590293134534, 0.005088878566307424370, 0.005480270542321714206, 0.005871662518336003174, 0.006263054494350293010 ),
 .UNSPECIFIED. ) ;
#15718=CARTESIAN_POINT ( 'NONE',  ( -0.8730628416137191650, -6.188929913094963986, 4.495049298931171222 ) ) ;
#15719=CARTESIAN_POINT ( 'NONE',  ( -3.634089073485423427, -4.776071126502695385, 12.49992002356259313 ) ) ;
#15722=CARTESIAN_POINT ( 'NONE',  ( 5.866817325727495813, 1.260653813892030017, 30.19977782616120621 ) ) ;
ENDSEC;
END-ISO-10303-21;
